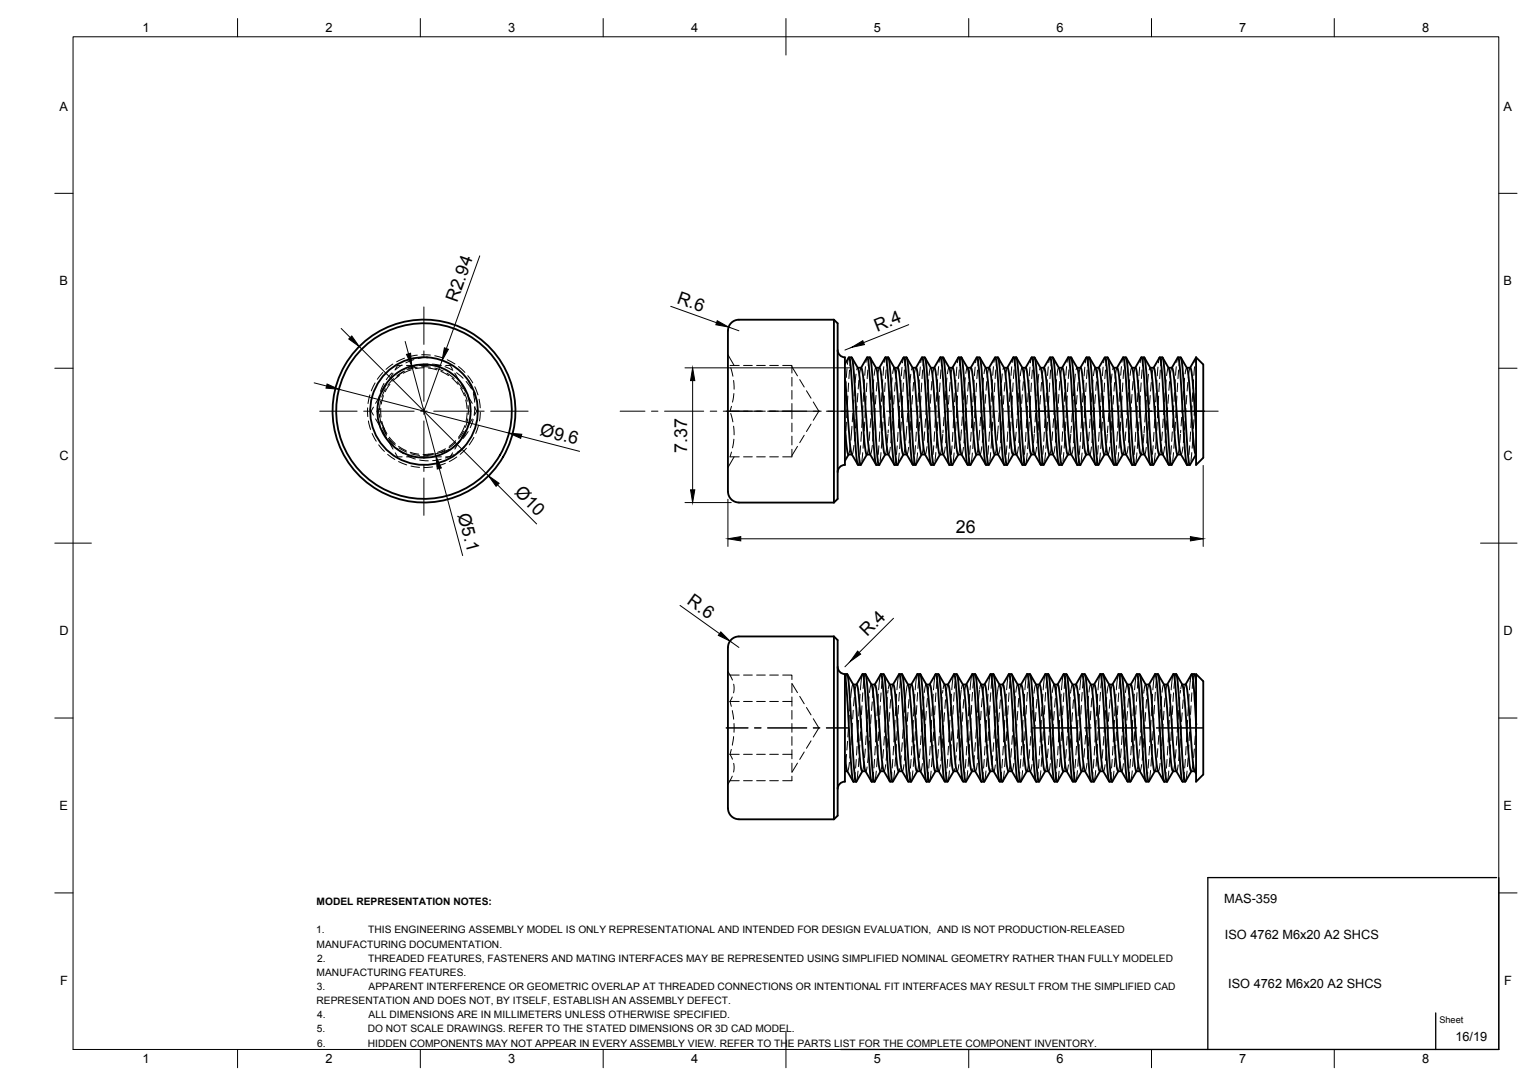
ISO-10303-21;
HEADER;
/* Generated by software containing ST-Developer
 * from STEP Tools, Inc. (www.steptools.com) 
 */

FILE_DESCRIPTION(
/* description */ (''),
/* implementation_level */ '2;1');

FILE_NAME(
/* name */ 'ISO 4762 M6x20 A2 SHCS.step',
/* time_stamp */ '2026-10-15T14:25:16-07:00',
/* author */ (''),
/* organization */ (''),
/* preprocessor_version */ 'ST-DEVELOPER v20.2',
/* originating_system */ 'Autodesk Translation Framework v15.15.0.0',
/* authorisation */ '');

FILE_SCHEMA (('AUTOMOTIVE_DESIGN { 1 0 10303 214 3 1 1 }'));
ENDSEC;

DATA;
#10=MECHANICAL_DESIGN_GEOMETRIC_PRESENTATION_REPRESENTATION('',(#338),#86429);
#157=TOROIDAL_SURFACE('',#17154,0.3342,0.04);
#158=TOROIDAL_SURFACE('',#17170,0.44,0.06);
#256=B_SPLINE_SURFACE_WITH_KNOTS('',3,3,((#76225,#76226,#76227,#76228,#76229,
#76230,#76231,#76232,#76233,#76234,#76235,#76236,#76237,#76238,#76239,#76240,
#76241,#76242,#76243,#76244,#76245,#76246,#76247,#76248,#76249,#76250,#76251,
#76252,#76253,#76254,#76255,#76256,#76257,#76258,#76259,#76260,#76261,#76262,
#76263,#76264,#76265,#76266,#76267,#76268,#76269,#76270,#76271,#76272,#76273,
#76274,#76275,#76276,#76277,#76278,#76279,#76280,#76281,#76282,#76283,#76284,
#76285,#76286,#76287,#76288,#76289,#76290,#76291,#76292,#76293,#76294,#76295,
#76296,#76297,#76298,#76299,#76300,#76301,#76302,#76303,#76304,#76305,#76306,
#76307,#76308,#76309,#76310,#76311,#76312,#76313,#76314,#76315,#76316,#76317,
#76318,#76319,#76320,#76321,#76322,#76323,#76324,#76325,#76326,#76327,#76328,
#76329,#76330,#76331,#76332,#76333,#76334,#76335,#76336,#76337,#76338,#76339,
#76340,#76341,#76342,#76343,#76344,#76345,#76346,#76347,#76348,#76349,#76350),
(#76351,#76352,#76353,#76354,#76355,#76356,#76357,#76358,#76359,#76360,
#76361,#76362,#76363,#76364,#76365,#76366,#76367,#76368,#76369,#76370,#76371,
#76372,#76373,#76374,#76375,#76376,#76377,#76378,#76379,#76380,#76381,#76382,
#76383,#76384,#76385,#76386,#76387,#76388,#76389,#76390,#76391,#76392,#76393,
#76394,#76395,#76396,#76397,#76398,#76399,#76400,#76401,#76402,#76403,#76404,
#76405,#76406,#76407,#76408,#76409,#76410,#76411,#76412,#76413,#76414,#76415,
#76416,#76417,#76418,#76419,#76420,#76421,#76422,#76423,#76424,#76425,#76426,
#76427,#76428,#76429,#76430,#76431,#76432,#76433,#76434,#76435,#76436,#76437,
#76438,#76439,#76440,#76441,#76442,#76443,#76444,#76445,#76446,#76447,#76448,
#76449,#76450,#76451,#76452,#76453,#76454,#76455,#76456,#76457,#76458,#76459,
#76460,#76461,#76462,#76463,#76464,#76465,#76466,#76467,#76468,#76469,#76470,
#76471,#76472,#76473,#76474,#76475,#76476),(#76477,#76478,#76479,#76480,
#76481,#76482,#76483,#76484,#76485,#76486,#76487,#76488,#76489,#76490,#76491,
#76492,#76493,#76494,#76495,#76496,#76497,#76498,#76499,#76500,#76501,#76502,
#76503,#76504,#76505,#76506,#76507,#76508,#76509,#76510,#76511,#76512,#76513,
#76514,#76515,#76516,#76517,#76518,#76519,#76520,#76521,#76522,#76523,#76524,
#76525,#76526,#76527,#76528,#76529,#76530,#76531,#76532,#76533,#76534,#76535,
#76536,#76537,#76538,#76539,#76540,#76541,#76542,#76543,#76544,#76545,#76546,
#76547,#76548,#76549,#76550,#76551,#76552,#76553,#76554,#76555,#76556,#76557,
#76558,#76559,#76560,#76561,#76562,#76563,#76564,#76565,#76566,#76567,#76568,
#76569,#76570,#76571,#76572,#76573,#76574,#76575,#76576,#76577,#76578,#76579,
#76580,#76581,#76582,#76583,#76584,#76585,#76586,#76587,#76588,#76589,#76590,
#76591,#76592,#76593,#76594,#76595,#76596,#76597,#76598,#76599,#76600,#76601,
#76602),(#76603,#76604,#76605,#76606,#76607,#76608,#76609,#76610,#76611,
#76612,#76613,#76614,#76615,#76616,#76617,#76618,#76619,#76620,#76621,#76622,
#76623,#76624,#76625,#76626,#76627,#76628,#76629,#76630,#76631,#76632,#76633,
#76634,#76635,#76636,#76637,#76638,#76639,#76640,#76641,#76642,#76643,#76644,
#76645,#76646,#76647,#76648,#76649,#76650,#76651,#76652,#76653,#76654,#76655,
#76656,#76657,#76658,#76659,#76660,#76661,#76662,#76663,#76664,#76665,#76666,
#76667,#76668,#76669,#76670,#76671,#76672,#76673,#76674,#76675,#76676,#76677,
#76678,#76679,#76680,#76681,#76682,#76683,#76684,#76685,#76686,#76687,#76688,
#76689,#76690,#76691,#76692,#76693,#76694,#76695,#76696,#76697,#76698,#76699,
#76700,#76701,#76702,#76703,#76704,#76705,#76706,#76707,#76708,#76709,#76710,
#76711,#76712,#76713,#76714,#76715,#76716,#76717,#76718,#76719,#76720,#76721,
#76722,#76723,#76724,#76725,#76726,#76727,#76728)),.UNSPECIFIED.,.F.,.F.,
 .F.,(4,4),(4,1,1,1,1,1,1,1,1,1,1,1,1,1,1,1,1,1,1,1,1,1,1,1,1,1,1,1,1,1,
1,1,1,1,1,1,1,1,1,1,1,1,1,1,1,1,1,1,1,1,1,1,1,1,1,1,1,1,1,1,1,1,1,1,1,1,
1,1,1,1,1,1,1,1,1,1,1,1,1,1,1,1,1,1,1,1,1,1,1,1,1,1,1,1,1,1,1,1,1,1,1,1,
1,1,1,1,1,1,1,1,1,1,1,1,1,1,1,1,1,1,1,1,1,4),(-0.000489095128896854,0.0662888134554226),
(8.30725886192223,9.30549431301254,10.303511073624,11.3015278342355,12.299544594847,
13.2975613554585,14.29557811607,15.2935948766815,16.291611637293,17.2896283979046,
18.287645158516,19.2856619191276,20.2836786797391,21.2816954403506,22.2797122009621,
23.2777289615736,24.2757457221851,25.2737624827966,26.2717792434081,27.2697960040196,
28.2678127646311,29.2658295252426,30.2638462858541,31.2618630464656,32.2598798070771,
33.2578965676886,34.2559133283001,35.2539300889116,36.2519468495231,37.2499636101346,
38.2479803707461,39.2459971313576,40.2440138919691,41.2420306525806,42.2400474131921,
43.2380641738036,44.2360809344151,45.2340976950266,46.2321144556381,47.2301312162496,
48.2281479768611,49.2261647374726,50.2241814980841,51.2221982586956,52.2202150193071,
53.2182317799186,54.2162485405301,55.2142653011416,56.2122820617531,57.2102988223646,
58.2083155829761,59.2063323435876,60.2043491041991,61.2023658648106,62.2003826254221,
63.1983993860336,64.1964161466451,65.1944329072566,66.1924496678681,67.1904664284796,
68.1884831890911,69.1864999497026,70.1845167103141,71.1825334709256,72.1805502315371,
73.1785669921486,74.1765837527601,75.1746005133716,76.1726172739831,77.1706340345946,
78.1686507952061,79.1666675558176,80.1646843164291,81.1627010770406,82.1607178376521,
83.1587345982636,84.1567513588751,85.1547681194866,86.1527848800981,87.1508016407096,
88.1488184013211,89.1468351619326,90.1448519225441,91.1428686831556,92.1408854437671,
93.1389022043786,94.1369189649901,95.1349357256016,96.1329524862131,97.1309692468246,
98.1289860074361,99.1270027680476,100.125019528659,101.123036289271,102.121053049882,
103.119069810494,104.117086571105,105.115103331717,106.113120092328,107.11113685294,
108.109153613551,109.107170374163,110.105187134774,111.103203895386,112.101220655997,
113.099237416609,114.09725417722,115.095270937832,116.093287698443,117.091304459055,
118.089321219666,119.087337980278,120.085354740889,121.083371501501,122.081388262112,
123.079405022724,124.077421783335,125.075438543947,126.073455304558,127.07147206517,
128.069488825781,129.067505586393,130.065522347004,131.064028202745),
 .UNSPECIFIED.);
#257=B_SPLINE_SURFACE_WITH_KNOTS('',3,3,((#76851,#76852,#76853,#76854,#76855,
#76856,#76857,#76858,#76859,#76860,#76861,#76862,#76863,#76864,#76865,#76866,
#76867,#76868,#76869,#76870,#76871,#76872,#76873,#76874,#76875,#76876,#76877,
#76878,#76879,#76880,#76881,#76882,#76883,#76884,#76885,#76886,#76887,#76888,
#76889,#76890,#76891,#76892,#76893,#76894,#76895,#76896,#76897,#76898,#76899,
#76900,#76901,#76902,#76903,#76904,#76905,#76906,#76907,#76908,#76909,#76910,
#76911,#76912,#76913,#76914,#76915,#76916,#76917,#76918,#76919,#76920,#76921,
#76922,#76923,#76924,#76925,#76926,#76927,#76928,#76929,#76930,#76931,#76932,
#76933,#76934,#76935,#76936,#76937,#76938,#76939,#76940,#76941,#76942,#76943,
#76944,#76945,#76946,#76947,#76948,#76949,#76950,#76951,#76952,#76953,#76954,
#76955,#76956,#76957,#76958,#76959,#76960,#76961,#76962,#76963,#76964,#76965,
#76966,#76967,#76968,#76969,#76970,#76971,#76972,#76973,#76974,#76975,#76976),
(#76977,#76978,#76979,#76980,#76981,#76982,#76983,#76984,#76985,#76986,
#76987,#76988,#76989,#76990,#76991,#76992,#76993,#76994,#76995,#76996,#76997,
#76998,#76999,#77000,#77001,#77002,#77003,#77004,#77005,#77006,#77007,#77008,
#77009,#77010,#77011,#77012,#77013,#77014,#77015,#77016,#77017,#77018,#77019,
#77020,#77021,#77022,#77023,#77024,#77025,#77026,#77027,#77028,#77029,#77030,
#77031,#77032,#77033,#77034,#77035,#77036,#77037,#77038,#77039,#77040,#77041,
#77042,#77043,#77044,#77045,#77046,#77047,#77048,#77049,#77050,#77051,#77052,
#77053,#77054,#77055,#77056,#77057,#77058,#77059,#77060,#77061,#77062,#77063,
#77064,#77065,#77066,#77067,#77068,#77069,#77070,#77071,#77072,#77073,#77074,
#77075,#77076,#77077,#77078,#77079,#77080,#77081,#77082,#77083,#77084,#77085,
#77086,#77087,#77088,#77089,#77090,#77091,#77092,#77093,#77094,#77095,#77096,
#77097,#77098,#77099,#77100,#77101,#77102),(#77103,#77104,#77105,#77106,
#77107,#77108,#77109,#77110,#77111,#77112,#77113,#77114,#77115,#77116,#77117,
#77118,#77119,#77120,#77121,#77122,#77123,#77124,#77125,#77126,#77127,#77128,
#77129,#77130,#77131,#77132,#77133,#77134,#77135,#77136,#77137,#77138,#77139,
#77140,#77141,#77142,#77143,#77144,#77145,#77146,#77147,#77148,#77149,#77150,
#77151,#77152,#77153,#77154,#77155,#77156,#77157,#77158,#77159,#77160,#77161,
#77162,#77163,#77164,#77165,#77166,#77167,#77168,#77169,#77170,#77171,#77172,
#77173,#77174,#77175,#77176,#77177,#77178,#77179,#77180,#77181,#77182,#77183,
#77184,#77185,#77186,#77187,#77188,#77189,#77190,#77191,#77192,#77193,#77194,
#77195,#77196,#77197,#77198,#77199,#77200,#77201,#77202,#77203,#77204,#77205,
#77206,#77207,#77208,#77209,#77210,#77211,#77212,#77213,#77214,#77215,#77216,
#77217,#77218,#77219,#77220,#77221,#77222,#77223,#77224,#77225,#77226,#77227,
#77228),(#77229,#77230,#77231,#77232,#77233,#77234,#77235,#77236,#77237,
#77238,#77239,#77240,#77241,#77242,#77243,#77244,#77245,#77246,#77247,#77248,
#77249,#77250,#77251,#77252,#77253,#77254,#77255,#77256,#77257,#77258,#77259,
#77260,#77261,#77262,#77263,#77264,#77265,#77266,#77267,#77268,#77269,#77270,
#77271,#77272,#77273,#77274,#77275,#77276,#77277,#77278,#77279,#77280,#77281,
#77282,#77283,#77284,#77285,#77286,#77287,#77288,#77289,#77290,#77291,#77292,
#77293,#77294,#77295,#77296,#77297,#77298,#77299,#77300,#77301,#77302,#77303,
#77304,#77305,#77306,#77307,#77308,#77309,#77310,#77311,#77312,#77313,#77314,
#77315,#77316,#77317,#77318,#77319,#77320,#77321,#77322,#77323,#77324,#77325,
#77326,#77327,#77328,#77329,#77330,#77331,#77332,#77333,#77334,#77335,#77336,
#77337,#77338,#77339,#77340,#77341,#77342,#77343,#77344,#77345,#77346,#77347,
#77348,#77349,#77350,#77351,#77352,#77353,#77354)),.UNSPECIFIED.,.F.,.F.,
 .F.,(4,4),(4,1,1,1,1,1,1,1,1,1,1,1,1,1,1,1,1,1,1,1,1,1,1,1,1,1,1,1,1,1,
1,1,1,1,1,1,1,1,1,1,1,1,1,1,1,1,1,1,1,1,1,1,1,1,1,1,1,1,1,1,1,1,1,1,1,1,
1,1,1,1,1,1,1,1,1,1,1,1,1,1,1,1,1,1,1,1,1,1,1,1,1,1,1,1,1,1,1,1,1,1,1,1,
1,1,1,1,1,1,1,1,1,1,1,1,1,1,1,1,1,1,1,1,1,4),(-0.000418746624015696,0.0663359285465069),
(11.6145437174728,12.6130496084297,13.6110663690412,14.6090831296527,15.6070998902642,
16.6051166508757,17.6031334114872,18.6011501720987,19.5991669327102,20.5971836933217,
21.5952004539332,22.5932172145448,23.5912339751562,24.5892507357678,25.5872674963793,
26.5852842569908,27.5833010176023,28.5813177782138,29.5793345388253,30.5773512994368,
31.5753680600483,32.5733848206598,33.5714015812713,34.5694183418828,35.5674351024943,
36.5654518631058,37.5634686237173,38.5614853843288,39.5595021449403,40.5575189055518,
41.5555356661633,42.5535524267748,43.5515691873863,44.5495859479978,45.5476027086093,
46.5456194692208,47.5436362298323,48.5416529904438,49.5396697510553,50.5376865116668,
51.5357032722783,52.5337200328898,53.5317367935013,54.5297535541128,55.5277703147243,
56.5257870753358,57.5238038359473,58.5218205965588,59.5198373571703,60.5178541177818,
61.5158708783933,62.5138876390048,63.5119043996163,64.5099211602278,65.5079379208393,
66.5059546814508,67.5039714420623,68.5019882026738,69.5000049632853,70.4980217238968,
71.4960384845083,72.4940552451198,73.4920720057313,74.4900887663428,75.4881055269543,
76.4861222875658,77.4841390481773,78.4821558087888,79.4801725694003,80.4781893300118,
81.4762060906233,82.4742228512348,83.4722396118463,84.4702563724578,85.4682731330693,
86.4662898936808,87.4643066542923,88.4623234149038,89.4603401755153,90.4583569361268,
91.4563736967383,92.4543904573498,93.4524072179613,94.4504239785728,95.4484407391843,
96.4464574997958,97.4444742604073,98.4424910210188,99.4405077816303,100.438524542242,
101.436541302853,102.434558063465,103.432574824076,104.430591584688,105.428608345299,
106.426625105911,107.424641866522,108.422658627134,109.420675387745,110.418692148357,
111.416708908968,112.41472566958,113.412742430191,114.410759190803,115.408775951414,
116.406792712026,117.404809472637,118.402826233249,119.40084299386,120.398859754472,
121.396876515083,122.394893275695,123.392910036306,124.390926796918,125.388943557529,
126.386960318141,127.384977078752,128.382993839364,129.381010599975,130.379027360587,
131.377044121198,132.37506088181,133.373077642421,134.371094403033),
 .UNSPECIFIED.);
#273=(
BOUNDED_CURVE()
B_SPLINE_CURVE(2,(#77369,#77370,#77371),.UNSPECIFIED.,.F.,.F.)
B_SPLINE_CURVE_WITH_KNOTS((3,3),(-0.639366558443436,-0.433164349146202),
 .UNSPECIFIED.)
CURVE()
GEOMETRIC_REPRESENTATION_ITEM()
RATIONAL_B_SPLINE_CURVE((1.35866716012837,1.4637604307034,1.4637604307034))
REPRESENTATION_ITEM('')
);
#274=(
BOUNDED_CURVE()
B_SPLINE_CURVE(2,(#77373,#77374,#77375),.UNSPECIFIED.,.F.,.F.)
B_SPLINE_CURVE_WITH_KNOTS((3,3),(0.0319010196424347,0.336489692457453),
 .UNSPECIFIED.)
CURVE()
GEOMETRIC_REPRESENTATION_ITEM()
RATIONAL_B_SPLINE_CURVE((1.03712812921102,1.19757240916823,1.03712812921102))
REPRESENTATION_ITEM('')
);
#275=(
BOUNDED_CURVE()
B_SPLINE_CURVE(2,(#77377,#77378,#77379),.UNSPECIFIED.,.F.,.F.)
B_SPLINE_CURVE_WITH_KNOTS((3,3),(0.0319010196424348,0.336489692457454),
 .UNSPECIFIED.)
CURVE()
GEOMETRIC_REPRESENTATION_ITEM()
RATIONAL_B_SPLINE_CURVE((1.03712812921102,1.19757240916823,1.03712812921102))
REPRESENTATION_ITEM('')
);
#276=(
BOUNDED_CURVE()
B_SPLINE_CURVE(2,(#77381,#77382,#77383),.UNSPECIFIED.,.F.,.F.)
B_SPLINE_CURVE_WITH_KNOTS((3,3),(0.031901019642435,0.336489692457454),
 .UNSPECIFIED.)
CURVE()
GEOMETRIC_REPRESENTATION_ITEM()
RATIONAL_B_SPLINE_CURVE((1.03712812921102,1.19757240916823,1.03712812921102))
REPRESENTATION_ITEM('')
);
#277=(
BOUNDED_CURVE()
B_SPLINE_CURVE(2,(#77385,#77386,#77387),.UNSPECIFIED.,.F.,.F.)
B_SPLINE_CURVE_WITH_KNOTS((3,3),(0.0319010196424349,0.336489692457453),
 .UNSPECIFIED.)
CURVE()
GEOMETRIC_REPRESENTATION_ITEM()
RATIONAL_B_SPLINE_CURVE((1.03712812921102,1.19757240916823,1.03712812921102))
REPRESENTATION_ITEM('')
);
#278=(
BOUNDED_CURVE()
B_SPLINE_CURVE(2,(#77389,#77390,#77391),.UNSPECIFIED.,.F.,.F.)
B_SPLINE_CURVE_WITH_KNOTS((3,3),(0.0319010196424348,0.336489692457453),
 .UNSPECIFIED.)
CURVE()
GEOMETRIC_REPRESENTATION_ITEM()
RATIONAL_B_SPLINE_CURVE((1.03712812921102,1.19757240916823,1.03712812921102))
REPRESENTATION_ITEM('')
);
#279=(
BOUNDED_CURVE()
B_SPLINE_CURVE(2,(#77392,#77393,#77394),.UNSPECIFIED.,.F.,.F.)
B_SPLINE_CURVE_WITH_KNOTS((3,3),(-0.433164349146202,-0.226962139848967),
 .UNSPECIFIED.)
CURVE()
GEOMETRIC_REPRESENTATION_ITEM()
RATIONAL_B_SPLINE_CURVE((1.4637604307034,1.4637604307034,1.35866716012837))
REPRESENTATION_ITEM('')
);
#302=SHAPE_REPRESENTATION_RELATIONSHIP('SRR','None',#86517,#320);
#320=ADVANCED_BREP_SHAPE_REPRESENTATION('',(#356),#86426);
#338=STYLED_ITEM('',(#86616),#356);
#356=MANIFOLD_SOLID_BREP('Body1',#15628);
#947=B_SPLINE_CURVE_WITH_KNOTS('',3,(#66636,#66637,#66638,#66639,#66640,
#66641,#66642,#66643,#66644,#66645,#66646,#66647,#66648,#66649,#66650,#66651,
#66652,#66653,#66654,#66655,#66656,#66657,#66658,#66659,#66660,#66661,#66662,
#66663,#66664,#66665,#66666,#66667,#66668,#66669,#66670,#66671,#66672,#66673,
#66674,#66675,#66676,#66677,#66678,#66679,#66680,#66681,#66682,#66683,#66684,
#66685,#66686,#66687,#66688,#66689,#66690,#66691,#66692,#66693,#66694,#66695,
#66696,#66697,#66698,#66699,#66700,#66701,#66702,#66703,#66704,#66705,#66706,
#66707,#66708,#66709,#66710,#66711),.UNSPECIFIED.,.F.,.F.,(4,3,3,3,3,3,
3,3,3,3,3,3,3,3,3,3,3,3,3,3,3,3,3,3,3,4),(10.3765110117404,10.553450790841,
10.7300519237118,10.9066404614712,11.0832321762531,11.2602038202997,11.3015278342355,
11.4805049057995,11.6591300536428,11.837736646534,12.0163195055085,12.1953225046721,
12.299544594847,12.477964982007,12.6560183737272,12.8340392590285,13.0120277045372,
13.190434319541,13.2975613554585,13.4762752215219,13.6546274568134,13.8329507487056,
14.0112440633789,14.1899534235983,14.29557811607,14.315035395632),
 .UNSPECIFIED.);
#948=B_SPLINE_CURVE_WITH_KNOTS('',3,(#66714,#66715,#66716,#66717,#66718,
#66719,#66720,#66721,#66722,#66723,#66724,#66725,#66726,#66727,#66728,#66729,
#66730,#66731,#66732,#66733,#66734,#66735,#66736,#66737,#66738,#66739,#66740,
#66741,#66742,#66743,#66744,#66745,#66746,#66747,#66748,#66749,#66750,#66751,
#66752,#66753,#66754,#66755,#66756,#66757,#66758,#66759,#66760,#66761,#66762),
 .UNSPECIFIED.,.F.,.F.,(4,3,3,3,3,3,3,3,3,3,3,3,3,3,3,3,4),(11.6150328478182,
11.7979606486813,11.9807538318031,12.1637609224241,12.3468733973939,12.5304979994706,
12.6130496084297,12.7898803693582,12.9663087351348,13.1426740016011,13.3189861820381,
13.4957160141166,13.6110663690412,13.790004086606,13.9685863611197,14.1471565225389,
14.3143732599613),.UNSPECIFIED.);
#949=B_SPLINE_CURVE_WITH_KNOTS('',3,(#66768,#66769,#66770,#66771,#66772,
#66773,#66774,#66775,#66776,#66777,#66778,#66779,#66780,#66781,#66782,#66783,
#66784,#66785,#66786,#66787,#66788,#66789,#66790,#66791,#66792,#66793,#66794,
#66795,#66796,#66797,#66798,#66799,#66800,#66801,#66802,#66803,#66804,#66805,
#66806,#66807,#66808,#66809,#66810,#66811,#66812,#66813,#66814,#66815,#66816,
#66817,#66818,#66819,#66820,#66821,#66822,#66823,#66824,#66825,#66826,#66827,
#66828,#66829,#66830,#66831,#66832,#66833,#66834,#66835,#66836,#66837,#66838,
#66839,#66840,#66841,#66842,#66843,#66844,#66845,#66846,#66847,#66848,#66849,
#66850,#66851,#66852,#66853,#66854,#66855,#66856,#66857,#66858,#66859,#66860,
#66861,#66862,#66863,#66864,#66865,#66866,#66867,#66868,#66869,#66870,#66871,
#66872,#66873,#66874,#66875,#66876,#66877,#66878,#66879,#66880,#66881,#66882,
#66883,#66884,#66885,#66886,#66887,#66888,#66889,#66890,#66891,#66892,#66893,
#66894,#66895,#66896,#66897,#66898,#66899,#66900,#66901,#66902,#66903,#66904,
#66905,#66906,#66907,#66908,#66909,#66910,#66911,#66912,#66913,#66914,#66915,
#66916,#66917,#66918,#66919,#66920,#66921,#66922,#66923,#66924,#66925,#66926,
#66927,#66928,#66929,#66930,#66931,#66932,#66933,#66934,#66935,#66936,#66937,
#66938,#66939,#66940,#66941,#66942,#66943),.UNSPECIFIED.,.F.,.F.,(4,2,2,
2,2,2,2,2,2,2,2,2,2,2,2,2,2,2,2,2,2,2,2,2,2,2,2,2,2,2,2,2,2,2,2,2,2,2,2,
2,2,2,2,2,2,2,2,2,2,2,2,2,2,2,2,2,2,2,2,2,2,2,2,2,2,2,2,2,2,2,2,2,2,2,2,
2,2,2,2,2,2,2,2,2,2,2,2,4),(-1.16393024442893,-1.1221121315859,-1.10881872775493,
-1.09544934716449,-1.09173058973152,-1.08953019556074,-1.08752664172342,
-1.08475168761754,-1.07807017871904,-1.06837433006326,-1.03766271561164,
-0.986967317852749,-0.977454673078762,-0.972924462585128,-0.969395708425164,
-0.965480163368157,-0.958971176180976,-0.932462287603271,-0.898938534238497,
-0.862323864343115,-0.856094385560679,-0.853588717151212,-0.851567613516379,
-0.849448493062549,-0.846097056573953,-0.835079364231314,-0.81540391299286,
-0.803966476133666,-0.749205411550143,-0.739933534931748,-0.735449519421135,
-0.731926722665925,-0.727986733892083,-0.721362440590357,-0.693068305980396,
-0.661126188336577,-0.62498318336144,-0.618724065166356,-0.616213585950999,
-0.614191439698589,-0.612074386397869,-0.608732469713031,-0.597803658723205,
-0.578369392903072,-0.565103910874299,-0.512002169030124,-0.502609093783704,
-0.498101699222849,-0.494575904380125,-0.490648422164753,-0.484083268407897,
-0.456726688401616,-0.424134078931558,-0.387566159612312,-0.38133545021858,
-0.37882929357464,-0.376807817974159,-0.374687075157398,-0.371333009017104,
-0.360304955609168,-0.340603341285605,-0.333711435315054,-0.273565360251425,
-0.264992529056898,-0.260586706715257,-0.257245427320754,-0.253405341354982,
-0.249363595655126,-0.24334388884479,-0.232352183683043,-0.205509402738985,
-0.167177413247694,-0.146863476916789,-0.142705047485694,-0.14038371096495,
-0.138409430867859,-0.135855093702301,-0.130411237430462,-0.123009150411749,
-0.103368057562215,-0.0503645383585366,-0.0314881958645743,-0.02544491739472,
-0.0216335334546739,-0.0182616452424589,-0.0148096369960941,-0.00864602604130215,
-0.00070557473632002),.UNSPECIFIED.);
#950=B_SPLINE_CURVE_WITH_KNOTS('',3,(#66944,#66945,#66946,#66947,#66948,
#66949,#66950,#66951,#66952,#66953,#66954,#66955,#66956,#66957,#66958,#66959,
#66960,#66961,#66962,#66963,#66964,#66965,#66966,#66967,#66968,#66969,#66970,
#66971),.UNSPECIFIED.,.F.,.F.,(4,3,3,3,3,3,3,3,3,4),(14.315035395632,14.4936872514172,
14.6719976991658,14.8502987123366,15.0285878152494,15.2072891407824,15.2935948766815,
15.4900540694702,15.685111908359,15.7079632676251),.UNSPECIFIED.);
#951=B_SPLINE_CURVE_WITH_KNOTS('',3,(#66973,#66974,#66975,#66976,#66977,
#66978,#66979,#66980,#66981,#66982,#66983,#66984,#66985,#66986,#66987,#66988,
#66989,#66990,#66991,#66992,#66993,#66994,#66995,#66996,#66997,#66998,#66999,
#67000),.UNSPECIFIED.,.F.,.F.,(4,3,3,3,3,3,3,3,3,4),(14.3143732599613,14.4932818470659,
14.6090831296527,14.7880601048648,14.9666851520948,15.1452916394554,15.3238743899854,
15.5028772782052,15.6070998902642,15.7079632679489),.UNSPECIFIED.);
#952=B_SPLINE_CURVE_WITH_KNOTS('',3,(#67001,#67002,#67003,#67004,#67005,
#67006,#67007,#67008,#67009,#67010,#67011,#67012,#67013,#67014,#67015,#67016,
#67017,#67018,#67019,#67020,#67021,#67022,#67023,#67024,#67025,#67026,#67027,
#67028,#67029,#67030,#67031,#67032,#67033,#67034,#67035,#67036,#67037,#67038,
#67039,#67040,#67041,#67042,#67043,#67044,#67045,#67046,#67047,#67048,#67049,
#67050,#67051,#67052,#67053,#67054,#67055,#67056,#67057,#67058,#67059,#67060,
#67061,#67062,#67063,#67064,#67065,#67066,#67067,#67068,#67069,#67070,#67071,
#67072,#67073,#67074,#67075,#67076,#67077,#67078,#67079,#67080,#67081,#67082,
#67083,#67084,#67085,#67086,#67087,#67088,#67089,#67090,#67091,#67092,#67093,
#67094,#67095,#67096,#67097,#67098,#67099,#67100,#67101,#67102,#67103,#67104,
#67105,#67106,#67107,#67108,#67109,#67110,#67111,#67112,#67113,#67114,#67115,
#67116,#67117,#67118,#67119,#67120,#67121,#67122,#67123,#67124,#67125,#67126,
#67127,#67128,#67129,#67130,#67131,#67132,#67133,#67134,#67135,#67136,#67137,
#67138,#67139,#67140,#67141,#67142,#67143,#67144,#67145,#67146,#67147,#67148,
#67149,#67150,#67151,#67152,#67153,#67154,#67155,#67156,#67157,#67158,#67159,
#67160,#67161,#67162),.UNSPECIFIED.,.F.,.F.,(4,2,2,2,2,2,2,2,2,2,2,2,2,
2,2,2,2,2,2,2,2,2,2,2,2,2,2,2,2,2,2,2,2,2,2,2,2,2,2,2,2,2,2,2,2,2,2,2,2,
2,2,2,2,2,2,2,2,2,2,2,2,2,2,2,2,2,2,2,2,2,2,2,2,2,2,2,2,2,2,2,4),(-2.98942615939622,
-2.94687744843447,-2.90737887780196,-2.90028833462003,-2.89626757009887,
-2.89278736806544,-2.88850740594506,-2.88194860504523,-2.83799867893463,
-2.79959280759611,-2.78803138120337,-2.78284147994681,-2.7788283302866,
-2.77655245813013,-2.7747160432841,-2.77226099931904,-2.76840197913877,
-2.74684477299445,-2.7014833079237,-2.66913041899145,-2.66227335609882,
-2.65827801354727,-2.65475565048187,-2.65033879153963,-2.64173110989955,
-2.58217996827536,-2.57531649807323,-2.55547164910086,-2.54439033061707,
-2.5410244222646,-2.53889684010004,-2.53687348626668,-2.53436524742632,
-2.52813036525468,-2.4917679525961,-2.45944377174351,-2.43180998977834,
-2.42522856169367,-2.42129812597274,-2.41777390166482,-2.41327434396693,
-2.40391952697214,-2.35010438134218,-2.33761336325053,-2.31801429303953,
-2.30702655289876,-2.30367990062065,-2.30156294068283,-2.29954488717194,
-2.29704277121525,-2.29082111843716,-2.25423947569581,-2.22151065226755,
-2.19433476155473,-2.18778874877106,-2.18386961472211,-2.18034945389465,
-2.17584679667526,-2.16645503385871,-2.11336918408685,-2.10013504463255,
-2.08062743095894,-2.06967603867303,-2.06633508998146,-2.06422055344751,
-2.06220017101256,-2.05969362054567,-2.05345255268914,-2.01714235715239,
-1.98492427180508,-1.95706758364123,-1.9504713292746,-1.94653757415735,
-1.94301382477905,-1.9385196018074,-1.92919317744503,-1.87520561547252,
-1.83454429703135,-1.83001991115689,-1.8276461646142,-1.82654679620979),
 .UNSPECIFIED.);
#953=B_SPLINE_CURVE_WITH_KNOTS('',3,(#67167,#67168,#67169,#67170,#67171,
#67172,#67173,#67174,#67175,#67176,#67177,#67178,#67179,#67180,#67181,#67182,
#67183,#67184,#67185,#67186,#67187,#67188,#67189,#67190,#67191,#67192,#67193,
#67194,#67195,#67196,#67197,#67198,#67199,#67200,#67201,#67202,#67203,#67204,
#67205,#67206,#67207,#67208,#67209,#67210,#67211,#67212,#67213,#67214,#67215,
#67216,#67217,#67218,#67219,#67220,#67221,#67222,#67223,#67224,#67225,#67226,
#67227,#67228,#67229,#67230,#67231,#67232,#67233,#67234,#67235,#67236,#67237,
#67238,#67239,#67240,#67241,#67242,#67243,#67244,#67245,#67246,#67247,#67248,
#67249,#67250,#67251,#67252,#67253,#67254,#67255,#67256,#67257,#67258,#67259,
#67260,#67261,#67262,#67263,#67264,#67265,#67266,#67267,#67268,#67269,#67270,
#67271,#67272,#67273,#67274,#67275,#67276,#67277,#67278,#67279,#67280,#67281,
#67282,#67283,#67284,#67285,#67286,#67287,#67288,#67289,#67290,#67291,#67292,
#67293,#67294,#67295,#67296,#67297,#67298,#67299,#67300,#67301,#67302,#67303,
#67304,#67305,#67306,#67307,#67308,#67309,#67310,#67311,#67312,#67313,#67314,
#67315,#67316,#67317,#67318,#67319,#67320,#67321,#67322,#67323,#67324,#67325,
#67326,#67327,#67328,#67329,#67330,#67331,#67332,#67333,#67334,#67335,#67336,
#67337,#67338,#67339,#67340,#67341,#67342,#67343,#67344,#67345,#67346,#67347,
#67348,#67349,#67350,#67351,#67352,#67353,#67354,#67355,#67356,#67357,#67358,
#67359,#67360,#67361,#67362,#67363,#67364,#67365,#67366,#67367,#67368,#67369,
#67370,#67371,#67372,#67373,#67374,#67375,#67376,#67377,#67378,#67379,#67380,
#67381,#67382),.UNSPECIFIED.,.F.,.F.,(4,2,2,2,2,2,2,2,2,2,2,2,2,2,2,2,2,
2,2,2,2,2,2,2,2,2,2,2,2,2,2,2,2,2,2,2,2,2,2,2,2,2,2,2,2,2,2,2,2,2,2,2,2,
2,2,2,2,2,2,2,2,2,2,2,2,2,2,2,2,2,2,2,2,2,2,2,2,2,2,2,2,2,2,2,2,2,2,2,2,
2,2,2,2,2,2,2,2,2,2,2,2,2,2,2,2,2,2,4),(-2.65811385973918,-2.64341887280631,
-2.63685547945785,-2.63292924488921,-2.62940468727833,-2.62489903708624,
-2.61551025001664,-2.56238128523994,-2.54919264361674,-2.52971894580261,
-2.51877761208218,-2.51543481805796,-2.51331789853485,-2.51129633688125,
-2.50878716273528,-2.50253408200726,-2.46640007387792,-2.43445651631383,
-2.40623004475929,-2.39961108197887,-2.39567265610066,-2.39215024322409,
-2.38766531765506,-2.37838640297329,-2.32371253981176,-2.31218416854247,
-2.29250660917671,-2.28148985781449,-2.27813883561977,-2.27602003237057,
-2.27399956303752,-2.27149476126776,-2.26526776294454,-2.22872118194875,
-2.1961529858716,-2.16881232025688,-2.16224953615428,-2.1583231805186,-2.15479821019637,
-2.15029161224657,-2.14089927817996,-2.08780637972958,-2.07456150657982,
-2.05509772052212,-2.04415967673414,-2.04081702101019,-2.03869999347207,
-2.03667816505093,-2.03416848444712,-2.02791325698376,-1.99179456385597,
-1.95987879084501,-1.93160587948036,-1.924983541931,-1.92104413243149,-1.91752147569834,
-1.91303711126042,-1.90376257244495,-1.84901801727298,-1.83755339109749,
-1.81786820831232,-1.80684826104643,-1.80349666903814,-1.8013775956048,
-1.79935691668679,-1.79685192957958,-1.79062483873777,-1.75406198815898,
-1.72147300873686,-1.69415644155959,-1.68759468993854,-1.68366826775868,
-1.68014280788343,-1.67563498858127,-1.66623787311483,-1.61320062663609,
-1.57165631512584,-1.56711236676727,-1.56473481914091,-1.56276388018841,
-1.56027892884346,-1.55632224374582,-1.53211804490594,-1.49545586039646,
-1.45803901320214,-1.45087621560002,-1.44677758808614,-1.44330536420355,
-1.43906067168766,-1.43099906766286,-1.38669425295883,-1.33778773774552,
-1.33106359083246,-1.32847789303883,-1.32661927783257,-1.32456966534925,
-1.32154352722031,-1.31319780845717,-1.30005877224877,-1.27130435927623,
-1.22453385002851,-1.21502442574756,-1.21047808041805,-1.20693773371413,
-1.20307033969169,-1.19678165452462,-1.17322533761841,-1.16393024442893),
 .UNSPECIFIED.);
#954=B_SPLINE_CURVE_WITH_KNOTS('',3,(#67383,#67384,#67385,#67386,#67387,
#67388,#67389,#67390,#67391,#67392,#67393,#67394,#67395,#67396,#67397,#67398,
#67399,#67400,#67401,#67402,#67403,#67404,#67405,#67406,#67407,#67408,#67409,
#67410,#67411,#67412,#67413,#67414,#67415,#67416,#67417,#67418,#67419,#67420,
#67421,#67422,#67423,#67424,#67425,#67426,#67427,#67428,#67429,#67430,#67431,
#67432,#67433,#67434,#67435,#67436,#67437,#67438,#67439,#67440,#67441,#67442,
#67443,#67444,#67445,#67446,#67447,#67448,#67449,#67450,#67451,#67452,#67453,
#67454,#67455,#67456,#67457,#67458,#67459,#67460,#67461,#67462,#67463,#67464,
#67465,#67466,#67467,#67468,#67469,#67470,#67471,#67472,#67473,#67474,#67475,
#67476,#67477,#67478,#67479,#67480,#67481,#67482,#67483,#67484,#67485,#67486,
#67487,#67488,#67489,#67490,#67491,#67492,#67493,#67494,#67495,#67496,#67497,
#67498,#67499,#67500,#67501,#67502,#67503,#67504,#67505,#67506,#67507,#67508,
#67509,#67510,#67511,#67512,#67513,#67514,#67515,#67516,#67517,#67518,#67519,
#67520,#67521,#67522,#67523,#67524,#67525,#67526,#67527,#67528,#67529,#67530,
#67531,#67532,#67533,#67534,#67535,#67536,#67537,#67538,#67539,#67540,#67541,
#67542,#67543,#67544,#67545,#67546,#67547,#67548,#67549,#67550,#67551,#67552,
#67553,#67554,#67555,#67556,#67557,#67558,#67559,#67560,#67561,#67562,#67563,
#67564,#67565,#67566,#67567,#67568,#67569,#67570,#67571,#67572,#67573,#67574,
#67575,#67576,#67577,#67578,#67579,#67580,#67581,#67582,#67583,#67584,#67585,
#67586,#67587,#67588,#67589,#67590,#67591,#67592),.UNSPECIFIED.,.F.,.F.,
(4,2,2,2,2,2,2,2,2,2,2,2,2,2,2,2,2,2,2,2,2,2,2,2,2,2,2,2,2,2,2,2,2,2,2,
2,2,2,2,2,2,2,2,2,2,2,2,2,2,2,2,2,2,2,2,2,2,2,2,2,2,2,2,2,2,2,2,2,2,2,2,
2,2,2,2,2,2,2,2,2,2,2,2,2,2,2,2,2,2,2,2,2,2,2,2,2,2,2,2,2,2,2,2,2,4),(-1.82654679620979,
-1.82567514256061,-1.82318578987642,-1.81921319040424,-1.7945975999961,
-1.78085997278393,-1.7509591994889,-1.72013307652391,-1.71336497138031,
-1.70939473836614,-1.7058785560794,-1.70144836983348,-1.69274827174082,
-1.63351771519777,-1.59712820036903,-1.59263831113477,-1.59027268554199,
-1.58830213870627,-1.58580575376867,-1.58180878732842,-1.55563188197764,
-1.54336480304901,-1.51968739046691,-1.49541669681936,-1.48036462094594,
-1.4747971116956,-1.47145663595873,-1.4678957223663,-1.46312196202823,-1.45224427397563,
-1.4122393108637,-1.3631967470555,-1.35660554113805,-1.35404011821867,-1.35218727325777,
-1.35013310945877,-1.34708239148078,-1.33855327348186,-1.32500659946013,
-1.25894060115722,-1.24314452828203,-1.23747258219032,-1.23411196404678,
-1.23056076484228,-1.22585342218376,-1.21536014310749,-1.20098137192243,
-1.15815776541184,-1.12236958235826,-1.118324968688,-1.11581402318508,-1.11384229735801,
-1.11148754612972,-1.10705055497943,-1.0743623081271,-1.02123830959475,
-1.00570661802811,-1.00007250684677,-0.996719268033883,-0.99316482249979,
-0.988434287423803,-0.977807444331893,-0.963186142593477,-0.918897988539242,
-0.885062430743449,-0.880985310049003,-0.878464863782423,-0.876492741512126,
-0.874145914767134,-0.869746244582656,-0.838975300467984,-0.79077979564977,
-0.769698590801541,-0.76340651574252,-0.759539578751323,-0.756001334220189,
-0.751382768040408,-0.741383638800634,-0.727888289896724,-0.689928879494222,
-0.650504547981136,-0.6443072230176,-0.641807771155571,-0.639788998631064,
-0.637668699900011,-0.634309761118168,-0.623215004476113,-0.603326541332951,
-0.595162166258294,-0.536884376366843,-0.52796871893014,-0.5235543137147,
-0.520039551252073,-0.51605907889055,-0.509243845237497,-0.477522095825476,
-0.430973442848463,-0.40989771349916,-0.405690896618916,-0.403359372530627,
-0.401385809699974,-0.398845112426623,-0.393478933319888,-0.355248774809182,
-0.332190119670129),.UNSPECIFIED.);
#955=B_SPLINE_CURVE_WITH_KNOTS('',3,(#67598,#67599,#67600,#67601,#67602,
#67603,#67604,#67605,#67606,#67607,#67608,#67609,#67610,#67611,#67612,#67613,
#67614,#67615,#67616,#67617,#67618,#67619,#67620,#67621,#67622,#67623,#67624,
#67625,#67626,#67627,#67628,#67629,#67630,#67631,#67632,#67633,#67634,#67635,
#67636,#67637,#67638,#67639,#67640,#67641,#67642,#67643,#67644,#67645,#67646,
#67647,#67648,#67649,#67650,#67651,#67652,#67653,#67654,#67655,#67656,#67657,
#67658,#67659,#67660,#67661,#67662,#67663,#67664,#67665,#67666,#67667,#67668,
#67669,#67670,#67671,#67672,#67673,#67674,#67675,#67676,#67677,#67678,#67679,
#67680,#67681,#67682,#67683,#67684,#67685,#67686,#67687,#67688,#67689,#67690,
#67691,#67692,#67693,#67694,#67695,#67696,#67697,#67698,#67699,#67700,#67701,
#67702,#67703,#67704,#67705,#67706,#67707,#67708,#67709,#67710,#67711,#67712,
#67713,#67714,#67715,#67716,#67717,#67718,#67719,#67720,#67721,#67722,#67723,
#67724,#67725,#67726,#67727,#67728,#67729,#67730,#67731,#67732,#67733,#67734,
#67735,#67736,#67737,#67738,#67739,#67740,#67741,#67742,#67743,#67744,#67745,
#67746,#67747,#67748,#67749,#67750,#67751,#67752,#67753,#67754,#67755,#67756,
#67757,#67758,#67759,#67760,#67761,#67762,#67763),.UNSPECIFIED.,.F.,.F.,
(4,2,2,2,2,2,2,2,2,2,2,2,2,2,2,2,2,2,2,2,2,2,2,2,2,2,2,2,2,2,2,2,2,2,2,
2,2,2,2,2,2,2,2,2,2,2,2,2,2,2,2,2,2,2,2,2,2,2,2,2,2,2,2,2,2,2,2,2,2,2,2,
2,2,2,2,2,2,2,2,2,2,2,4),(-1.16365104910194,-1.16198873409848,-1.11873333451251,
-1.08007682483228,-1.07289533808751,-1.06879292991221,-1.06532147429848,
-1.06108261121265,-1.05304736223389,-1.01380643672128,-0.974354768874303,
-0.955615421727428,-0.95154095556962,-0.949238925381929,-0.947279975777236,
-0.944706537452359,-0.939168763503621,-0.931601350956711,-0.911272521420545,
-0.864697156551351,-0.841359959454907,-0.834859417924407,-0.830946538256954,
-0.827418656268732,-0.822887438665612,-0.813364699776189,-0.800702995228171,
-0.766805215685698,-0.721392566400016,-0.715391258738159,-0.712957370947077,
-0.710954958021573,-0.708805444312101,-0.705315425122888,-0.692920314092189,
-0.669266049918139,-0.611703523646731,-0.600662162343852,-0.596217640945699,
-0.592926913172538,-0.589328930082488,-0.584341614312926,-0.572173887692835,
-0.506645012856004,-0.504000582658459,-0.493537335427797,-0.480167288699852,
-0.476449005709923,-0.474249008124355,-0.47224603922321,-0.4694720984499,
-0.462793799245578,-0.45310336172613,-0.422417340554128,-0.37169541728193,
-0.362185648162151,-0.357656682611973,-0.35412885374973,-0.35021429531376,
-0.343706866024677,-0.317203459323662,-0.28368579624041,-0.247072372632416,
-0.240849064767332,-0.238124138572478,-0.236151648600852,-0.234309633850536,
-0.231056093345189,-0.220914738422784,-0.203536525041064,-0.150699833390058,
-0.128996687355292,-0.122647285439585,-0.118767180860785,-0.11523123553389,
-0.110636222873976,-0.1007701932916,-0.0875102476811494,-0.0507450523485492,
-0.00710859726825555,-0.00274825577811126,-0.00126848880133153,-0.000702321398189432),
 .UNSPECIFIED.);
#956=B_SPLINE_CURVE_WITH_KNOTS('',3,(#67764,#67765,#67766,#67767,#67768,
#67769,#67770,#67771,#67772,#67773,#67774,#67775,#67776,#67777,#67778,#67779,
#67780,#67781,#67782,#67783,#67784,#67785,#67786,#67787,#67788,#67789,#67790,
#67791,#67792,#67793,#67794,#67795,#67796,#67797,#67798,#67799,#67800,#67801,
#67802,#67803,#67804,#67805,#67806,#67807,#67808,#67809,#67810,#67811,#67812,
#67813,#67814,#67815),.UNSPECIFIED.,.F.,.F.,(4,2,2,2,2,2,2,2,2,2,2,2,2,
2,2,2,2,2,2,2,2,2,2,2,2,4),(-2.9893848513208,-2.98893747316369,-2.9876025158476,
-2.98546557946283,-2.98216250725133,-2.97197352792502,-2.96355815815491,
-2.90631730564084,-2.88926272540383,-2.87733951087504,-2.87239217835099,
-2.86880219859959,-2.86550441099093,-2.86102835754096,-2.84979189282628,
-2.77362471164541,-2.76248320507388,-2.75507907488132,-2.75285138792675,
-2.75074533201809,-2.74881523310293,-2.7460912084198,-2.739870957641,-2.7033280354885,
-2.67077630094081,-2.65811385973918),.UNSPECIFIED.);
#957=B_SPLINE_CURVE_WITH_KNOTS('',3,(#67817,#67818,#67819,#67820,#67821,
#67822,#67823,#67824,#67825,#67826,#67827,#67828,#67829,#67830,#67831,#67832,
#67833,#67834,#67835,#67836,#67837,#67838,#67839,#67840,#67841,#67842,#67843,
#67844,#67845,#67846,#67847,#67848,#67849,#67850,#67851,#67852,#67853,#67854,
#67855,#67856,#67857,#67858,#67859,#67860,#67861,#67862,#67863,#67864,#67865,
#67866,#67867,#67868,#67869,#67870,#67871,#67872,#67873,#67874,#67875,#67876,
#67877,#67878,#67879,#67880,#67881,#67882,#67883,#67884,#67885,#67886,#67887,
#67888,#67889,#67890,#67891,#67892,#67893,#67894,#67895,#67896,#67897,#67898,
#67899,#67900,#67901,#67902,#67903,#67904,#67905,#67906,#67907,#67908,#67909,
#67910,#67911,#67912),.UNSPECIFIED.,.F.,.F.,(4,2,2,2,2,2,2,2,2,2,2,2,2,
2,2,2,2,2,2,2,2,2,2,2,2,2,2,2,2,2,2,2,2,2,2,2,2,2,2,2,2,2,2,2,2,2,2,4),
(-0.332190119670129,-0.299974256783078,-0.29076182289428,-0.286290157332493,
-0.282769813927846,-0.282625201287161,-0.282512604791512,-0.282424919666148,
-0.282356617668773,-0.282303400836696,-0.282223074884288,-0.2821468634119,
-0.282074529573626,-0.282005851482837,-0.281940621293291,-0.281878644309835,
-0.281819738143039,-0.281763731896355,-0.281710465402988,-0.281659788503258,
-0.281611560369081,-0.281565648872144,-0.281521929981461,-0.281480287226152,
-0.28144061117419,-0.281402798955855,-0.281366753823448,-0.277086765497933,
-0.268113946574196,-0.25627891769557,-0.226021878457394,-0.178535972958935,
-0.17031557559799,-0.167215471896808,-0.165356270008634,-0.163309071896805,
-0.160291684989588,-0.152003104953454,-0.10448895096256,-0.0779098348769532,
-0.05747216958326,-0.0512538036654406,-0.0474028352405869,-0.0438597472645543,
-0.0403992630740389,-0.0358762841793266,-0.023929538719514,-0.000702291658524479),
 .UNSPECIFIED.);
#958=B_SPLINE_CURVE_WITH_KNOTS('',3,(#67913,#67914,#67915,#67916,#67917,
#67918,#67919,#67920,#67921,#67922,#67923,#67924,#67925,#67926,#67927,#67928,
#67929,#67930,#67931,#67932,#67933,#67934,#67935,#67936,#67937,#67938,#67939,
#67940,#67941,#67942,#67943,#67944,#67945,#67946,#67947,#67948,#67949,#67950,
#67951,#67952,#67953,#67954,#67955,#67956,#67957,#67958,#67959,#67960,#67961,
#67962,#67963,#67964,#67965,#67966,#67967,#67968,#67969,#67970,#67971,#67972,
#67973,#67974,#67975,#67976,#67977,#67978,#67979,#67980,#67981,#67982,#67983,
#67984,#67985,#67986,#67987,#67988,#67989,#67990,#67991,#67992,#67993,#67994,
#67995,#67996,#67997,#67998,#67999,#68000,#68001,#68002,#68003,#68004,#68005,
#68006,#68007,#68008,#68009,#68010,#68011,#68012,#68013,#68014,#68015,#68016,
#68017,#68018,#68019,#68020,#68021,#68022,#68023,#68024,#68025,#68026,#68027,
#68028,#68029,#68030,#68031,#68032,#68033,#68034,#68035,#68036,#68037,#68038,
#68039,#68040,#68041,#68042,#68043,#68044,#68045,#68046,#68047,#68048,#68049,
#68050,#68051,#68052,#68053,#68054,#68055,#68056,#68057,#68058,#68059,#68060,
#68061,#68062,#68063,#68064,#68065,#68066,#68067,#68068,#68069,#68070,#68071,
#68072,#68073,#68074,#68075,#68076,#68077,#68078,#68079,#68080,#68081,#68082,
#68083,#68084,#68085,#68086,#68087,#68088,#68089,#68090,#68091,#68092,#68093,
#68094,#68095,#68096,#68097,#68098,#68099,#68100,#68101,#68102,#68103,#68104,
#68105,#68106,#68107,#68108),.UNSPECIFIED.,.F.,.F.,(4,2,2,2,2,2,2,2,2,2,
2,2,2,2,2,2,2,2,2,2,2,2,2,2,2,2,2,2,2,2,2,2,2,2,2,2,2,2,2,2,2,2,2,2,2,2,
2,2,2,2,2,2,2,2,2,2,2,2,2,2,2,2,2,2,2,2,2,2,2,2,2,2,2,2,2,2,2,2,2,2,2,2,
2,2,2,2,2,2,2,2,2,2,2,2,2,2,2,4),(-2.98897358008687,-2.92769314209762,-2.92283635649671,
-2.91891607758328,-2.91667246239068,-2.91468429829351,-2.9120511288804,
-2.90602483674824,-2.85973597595541,-2.82644850336208,-2.81392147458867,
-2.80456842641748,-2.80028193766707,-2.80021757807928,-2.80014854592242,
-2.80007429804235,-2.79999420251525,-2.79990751963336,-2.79981337778569,
-2.79971074256605,-2.79959837680186,-2.79947478825607,-2.7993381603811,
-2.79918625944562,-2.79910282444393,-2.79894676733214,-2.7986404194696,
-2.79512089876872,-2.79065274727909,-2.78145663265082,-2.7261184372274,
-2.68653475198969,-2.68201786236957,-2.67964667784219,-2.6776764846138,
-2.67518682288345,-2.67121230847029,-2.6465385500168,-2.60381980183744,
-2.57218735140361,-2.56537747406849,-2.56139840445967,-2.55788383669279,
-2.55346828700893,-2.54454549542632,-2.48629755644931,-2.47808810643394,
-2.45818707535278,-2.44708889637699,-2.44372974284319,-2.44160952912779,
-2.4395909662627,-2.43709198168734,-2.43089673012719,-2.3914888195501,-2.35356167696314,
-2.34007362068281,-2.33007780218808,-2.32545997520698,-2.32192195528628,
-2.31805492340576,-2.3117619328311,-2.29066986050776,-2.24245176471885,
-2.21166913656067,-2.20726891292452,-2.20492200279276,-2.20294992363011,
-2.20042969097544,-2.19635325451221,-2.16252425488423,-2.1577595822794,
-2.12368275873593,-2.09697182148208,-2.09045172116841,-2.08653517742575,
-2.08300913125178,-2.07848745284167,-2.06901214652698,-2.01745666702726,
-1.98731902900585,-1.97772631630079,-1.9710993642418,-1.96833439561336,
-1.96633333461326,-1.96413046746479,-1.96039731815009,-1.94685350251339,
-1.93673283316637,-1.92126868736453,-1.8800268546076,-1.86592293387262,
-1.85558121982064,-1.85090091581163,-1.84735388977835,-1.84351479821116,
-1.83735142483573,-1.82625073863295),.UNSPECIFIED.);
#959=B_SPLINE_CURVE_WITH_KNOTS('',3,(#68113,#68114,#68115,#68116,#68117,
#68118,#68119,#68120,#68121,#68122,#68123,#68124,#68125,#68126,#68127,#68128,
#68129,#68130,#68131,#68132,#68133,#68134,#68135,#68136,#68137,#68138,#68139,
#68140,#68141,#68142,#68143,#68144,#68145,#68146,#68147,#68148,#68149,#68150,
#68151,#68152,#68153,#68154,#68155,#68156,#68157,#68158,#68159,#68160,#68161,
#68162,#68163,#68164,#68165,#68166,#68167,#68168,#68169,#68170,#68171,#68172,
#68173,#68174,#68175,#68176,#68177,#68178,#68179,#68180,#68181,#68182,#68183,
#68184,#68185,#68186,#68187,#68188,#68189,#68190,#68191,#68192,#68193,#68194,
#68195,#68196,#68197,#68198,#68199,#68200,#68201,#68202,#68203,#68204,#68205,
#68206,#68207,#68208,#68209,#68210,#68211,#68212,#68213,#68214,#68215,#68216,
#68217,#68218,#68219,#68220,#68221,#68222,#68223,#68224,#68225,#68226,#68227,
#68228,#68229,#68230,#68231,#68232,#68233,#68234,#68235,#68236,#68237,#68238,
#68239,#68240,#68241,#68242,#68243,#68244,#68245,#68246,#68247,#68248,#68249,
#68250,#68251,#68252,#68253,#68254,#68255,#68256,#68257,#68258,#68259,#68260,
#68261,#68262,#68263,#68264,#68265,#68266,#68267,#68268,#68269,#68270,#68271,
#68272,#68273,#68274,#68275,#68276,#68277,#68278,#68279,#68280,#68281,#68282,
#68283,#68284,#68285,#68286,#68287,#68288,#68289,#68290,#68291,#68292,#68293,
#68294,#68295,#68296,#68297,#68298,#68299,#68300,#68301,#68302,#68303,#68304,
#68305,#68306,#68307,#68308,#68309,#68310,#68311,#68312,#68313,#68314,#68315,
#68316,#68317,#68318,#68319,#68320,#68321,#68322,#68323,#68324,#68325,#68326,
#68327,#68328,#68329,#68330,#68331,#68332),.UNSPECIFIED.,.F.,.F.,(4,2,2,
2,2,2,2,2,2,2,2,2,2,2,2,2,2,2,2,2,2,2,2,2,2,2,2,2,2,2,2,2,2,2,2,2,2,2,2,
2,2,2,2,2,2,2,2,2,2,2,2,2,2,2,2,2,2,2,2,2,2,2,2,2,2,2,2,2,2,2,2,2,2,2,2,
2,2,2,2,2,2,2,2,2,2,2,2,2,2,2,2,2,2,2,2,2,2,2,2,2,2,2,2,2,2,2,2,2,2,4),
(-2.65746774305231,-2.65261804205566,-2.64584623324261,-2.62617272996607,
-2.615158715998,-2.61180870310401,-2.60969057770515,-2.60767078381733,-2.60516685459269,
-2.59894220127053,-2.56240086795725,-2.52983407927815,-2.5025163264511,
-2.4959566011589,-2.49203172690838,-2.48850786796351,-2.48400238850228,
-2.47461125209531,-2.42156657618331,-2.40828353613625,-2.38883638532185,
-2.37790572301896,-2.37456456956123,-2.37244832301837,-2.37042708978095,
-2.36791799108521,-2.36166341956384,-2.3255746626612,-2.2936985406124,-2.26539500955471,
-2.25877237795713,-2.25483372512526,-2.25131232252042,-2.24683034551568,
-2.23756365834511,-2.18277827436322,-2.17137556262963,-2.1516918972459,
-2.14067375523214,-2.13732307541338,-2.13520466037621,-2.13318470453986,
-2.13068069407162,-2.12445643857931,-2.08788702671947,-2.0551634332501,
-2.02799948587829,-2.02144936529857,-2.0175263187276,-2.01400164189302,
-2.00949171294237,-2.00007853200098,-1.94738375203425,-1.91806825964147,
-1.90862556174804,-1.90207648863689,-1.89932450422995,-1.89732548159356,
-1.89511670599879,-1.89135670056093,-1.87751250941603,-1.86804159384396,
-1.82509180481262,-1.79421630215818,-1.78565730401293,-1.78131308838638,
-1.77780387481513,-1.77377471181276,-1.76691604016749,-1.73688615852472,
-1.68578013459207,-1.66727315857274,-1.66332871016514,-1.66107944988934,
-1.6590919804408,-1.65646702327566,-1.65048992885583,-1.60317010610248,
-1.55639897987041,-1.54815030595161,-1.54386836370732,-1.54036272421504,
-1.53628518103136,-1.5292125310971,-1.49473056438907,-1.46722289421195,
-1.46251149378335,-1.43097650505498,-1.4269038680685,-1.42438472433374,
-1.42241262300298,-1.42006456128484,-1.41565919958629,-1.38460982826758,
-1.33569511012369,-1.31546921485392,-1.30927375427337,-1.30542774023406,
-1.30188303067876,-1.29721857384015,-1.28696539389295,-1.27301799952048,
-1.20017970924618,-1.19119696202027,-1.18798359961284,-1.1861022609768,
-1.18407387501954,-1.18115436225658,-1.17354740652748,-1.16365104910194),
 .UNSPECIFIED.);
#960=B_SPLINE_CURVE_WITH_KNOTS('',3,(#68333,#68334,#68335,#68336,#68337,
#68338,#68339,#68340,#68341,#68342,#68343,#68344,#68345,#68346,#68347,#68348,
#68349,#68350,#68351,#68352,#68353,#68354,#68355,#68356,#68357,#68358,#68359,
#68360,#68361,#68362,#68363,#68364,#68365,#68366,#68367,#68368,#68369,#68370,
#68371,#68372,#68373,#68374,#68375,#68376,#68377,#68378,#68379,#68380,#68381,
#68382,#68383,#68384,#68385,#68386,#68387,#68388,#68389,#68390,#68391,#68392,
#68393,#68394,#68395,#68396,#68397,#68398,#68399,#68400,#68401,#68402,#68403,
#68404,#68405,#68406,#68407,#68408,#68409,#68410,#68411,#68412,#68413,#68414,
#68415,#68416,#68417,#68418,#68419,#68420,#68421,#68422,#68423,#68424,#68425,
#68426,#68427,#68428,#68429,#68430,#68431,#68432,#68433,#68434,#68435,#68436,
#68437,#68438,#68439,#68440,#68441,#68442,#68443,#68444,#68445,#68446,#68447,
#68448,#68449,#68450,#68451,#68452,#68453,#68454,#68455,#68456,#68457,#68458,
#68459,#68460,#68461,#68462,#68463,#68464,#68465,#68466,#68467,#68468,#68469,
#68470,#68471,#68472,#68473,#68474,#68475,#68476,#68477,#68478,#68479,#68480,
#68481,#68482,#68483,#68484,#68485,#68486,#68487,#68488,#68489,#68490,#68491,
#68492,#68493,#68494,#68495,#68496,#68497,#68498,#68499,#68500,#68501,#68502,
#68503,#68504,#68505,#68506,#68507,#68508,#68509,#68510,#68511,#68512,#68513,
#68514,#68515,#68516,#68517,#68518,#68519,#68520,#68521,#68522,#68523,#68524,
#68525,#68526,#68527,#68528,#68529,#68530,#68531,#68532,#68533,#68534,#68535,
#68536,#68537,#68538,#68539,#68540,#68541,#68542,#68543,#68544),
 .UNSPECIFIED.,.F.,.F.,(4,2,2,2,2,2,2,2,2,2,2,2,2,2,2,2,2,2,2,2,2,2,2,2,
2,2,2,2,2,2,2,2,2,2,2,2,2,2,2,2,2,2,2,2,2,2,2,2,2,2,2,2,2,2,2,2,2,2,2,2,
2,2,2,2,2,2,2,2,2,2,2,2,2,2,2,2,2,2,2,2,2,2,2,2,2,2,2,2,2,2,2,2,2,2,2,2,
2,2,2,2,2,2,2,2,2,4),(-1.82625073863295,-1.81743048083367,-1.76819131431197,
-1.7370057602039,-1.73259681582595,-1.73024795135637,-1.72827585061212,
-1.72575766004703,-1.72168845751425,-1.69070653630609,-1.65995402162083,
-1.63551189232338,-1.6251599607778,-1.61701484637726,-1.61275381803255,
-1.60958890756908,-1.60561783324043,-1.59884743904035,-1.57172333339439,
-1.57012941610718,-1.5175731179029,-1.49886167212502,-1.49490514287303,
-1.49265312027545,-1.49066610548489,-1.48799963132586,-1.48194934058225,
-1.47345024551375,-1.44894084451354,-1.38857164734317,-1.3800187117489,
-1.37561883703829,-1.3721049547582,-1.36811401181362,-1.36125184949231,
-1.3285933809597,-1.28218877469639,-1.26188622135384,-1.25772928959791,
-1.25540878585404,-1.25343370313395,-1.25087701062807,-1.24542761236607,
-1.23801716266803,-1.21834663865769,-1.20682946572698,-1.15215376976889,
-1.14287592453066,-1.13839133487293,-1.13486912035124,-1.1309308663737,
-1.12431214512924,-1.09609335014294,-1.06409684036266,-1.02791937825338,
-1.02166335560134,-1.01915371437839,-1.0171320839256,-1.01501548487916,
-1.01167399187847,-1.0007439690132,-0.98130423258884,-0.968028781115128,
-0.914962610035953,-0.905570343790112,-0.901064113184676,-0.897539589849428,
-0.893613914261244,-0.887052774060993,-0.859734433934364,-0.827109429478095,
-0.790514602968309,-0.784285731805667,-0.781780760959654,-0.779760412203886,
-0.777642073798023,-0.774292473562495,-0.763286511599889,-0.743640856571713,
-0.731864035548962,-0.677451036256476,-0.668153166831811,-0.663664940887641,
-0.660142527666568,-0.65620680828103,-0.649599014408321,-0.621550080724126,
-0.589434878029331,-0.553184169763361,-0.546934358455406,-0.544425868211862,
-0.542404632110245,-0.54028778475524,-0.536944751713608,-0.525999154515777,
-0.506516698972738,-0.493440679296154,-0.440228348932964,-0.430846043315784,
-0.426341876093813,-0.422817783558311,-0.418891368708921,-0.412326071473523,
-0.384939270089989,-0.352363406606311,-0.33180592744104),.UNSPECIFIED.);
#961=B_SPLINE_CURVE_WITH_KNOTS('',3,(#68550,#68551,#68552,#68553,#68554,
#68555,#68556,#68557,#68558,#68559,#68560,#68561,#68562,#68563,#68564,#68565,
#68566,#68567,#68568,#68569,#68570,#68571,#68572,#68573,#68574,#68575,#68576,
#68577,#68578,#68579,#68580,#68581,#68582,#68583,#68584,#68585,#68586,#68587,
#68588,#68589,#68590,#68591,#68592,#68593,#68594,#68595,#68596,#68597,#68598,
#68599,#68600,#68601,#68602,#68603,#68604,#68605,#68606,#68607,#68608,#68609,
#68610,#68611,#68612,#68613,#68614,#68615,#68616,#68617,#68618,#68619,#68620,
#68621,#68622,#68623,#68624,#68625,#68626,#68627,#68628,#68629,#68630,#68631,
#68632,#68633,#68634,#68635,#68636,#68637,#68638,#68639,#68640,#68641,#68642,
#68643,#68644,#68645,#68646,#68647,#68648,#68649,#68650,#68651,#68652,#68653,
#68654,#68655,#68656,#68657,#68658,#68659,#68660,#68661,#68662,#68663,#68664,
#68665,#68666,#68667,#68668,#68669,#68670,#68671,#68672,#68673,#68674,#68675,
#68676,#68677,#68678,#68679,#68680,#68681,#68682,#68683,#68684,#68685,#68686,
#68687,#68688,#68689,#68690,#68691,#68692,#68693,#68694,#68695,#68696,#68697,
#68698,#68699,#68700,#68701,#68702,#68703,#68704,#68705,#68706,#68707,#68708,
#68709,#68710,#68711,#68712,#68713,#68714,#68715,#68716,#68717,#68718,#68719,
#68720,#68721,#68722,#68723,#68724,#68725,#68726,#68727,#68728,#68729),
 .UNSPECIFIED.,.F.,.F.,(4,2,2,2,2,2,2,2,2,2,2,2,2,2,2,2,2,2,2,2,2,2,2,2,
2,2,2,2,2,2,2,2,2,2,2,2,2,2,2,2,2,2,2,2,2,2,2,2,2,2,2,2,2,2,2,2,2,2,2,2,
2,2,2,2,2,2,2,2,2,2,2,2,2,2,2,2,2,2,2,2,2,2,2,2,2,2,2,2,2,4),(-1.16363369234352,
-1.16295790678583,-1.15898823988006,-1.15222521336478,-1.12151620897351,
-1.0914958340154,-1.07796261271634,-1.05309843885021,-1.04911505999603,
-1.04662240929076,-1.04465156623561,-1.04228158322413,-1.0377723225715,
-0.999306261595195,-0.942744148510771,-0.933643853752399,-0.929193356432228,
-0.925674754874985,-0.921716221149426,-0.915003741001527,-0.885201841163423,
-0.854535777790885,-0.848020169730516,-0.815955518207676,-0.811881134326602,
-0.809361399704959,-0.807389161869915,-0.805041325635805,-0.800637404062841,
-0.769667244373821,-0.720955423652076,-0.700490299246686,-0.694268838917962,
-0.69041704342088,-0.686873898821883,-0.682221590823078,-0.672037005029608,
-0.658212364211504,-0.587646533901273,-0.576690947281024,-0.573223401629135,
-0.57107887319902,-0.569050507351872,-0.566131347764967,-0.558527132688328,
-0.54697430039157,-0.503767844145718,-0.465050987403647,-0.457868502874748,
-0.453765792591738,-0.450294235154145,-0.446055437065266,-0.438020902376893,
-0.398980220917527,-0.359911337502345,-0.340637027524395,-0.33653319357697,
-0.334224483342421,-0.332266412336735,-0.32970263543321,-0.32421663468579,
-0.316741411562477,-0.296800924411448,-0.257284792886249,-0.227183245499586,
-0.220308635565535,-0.216275186853487,-0.212922047147884,-0.212799261089963,
-0.212686912750328,-0.212583554354981,-0.212487997172239,-0.212399255293022,
-0.212316503547186,-0.212239045552849,-0.212166289148202,-0.21209772728177,
-0.207829510722542,-0.202892439011164,-0.194675785088698,-0.177398604672938,
-0.107522448590471,-0.10071895347576,-0.0981229310198588,-0.0962616113804328,
-0.0942146686741461,-0.0912019036092385,-0.0829525861352058,-0.0700249612576247,
-0.000702836714805313),.UNSPECIFIED.);
#962=B_SPLINE_CURVE_WITH_KNOTS('',3,(#68730,#68731,#68732,#68733,#68734,
#68735,#68736,#68737,#68738,#68739,#68740,#68741,#68742,#68743,#68744,#68745,
#68746,#68747,#68748,#68749,#68750,#68751,#68752,#68753,#68754,#68755,#68756,
#68757,#68758,#68759,#68760,#68761,#68762,#68763,#68764,#68765,#68766,#68767,
#68768,#68769,#68770,#68771,#68772,#68773,#68774,#68775,#68776,#68777,#68778,
#68779,#68780,#68781,#68782,#68783),.UNSPECIFIED.,.F.,.F.,(4,2,2,2,2,2,
2,2,2,2,2,2,2,2,2,2,2,2,2,2,2,2,2,2,2,2,4),(-2.98872595129121,-2.97578488693837,
-2.97135777031141,-2.96792934948171,-2.96453074422925,-2.96066679337635,
-2.95438691435237,-2.93333516725447,-2.89683441943583,-2.86718109747591,
-2.85767739453118,-2.85109695767192,-2.8483400404559,-2.84634053495174,
-2.84413463115462,-2.84038652557546,-2.82667029217726,-2.81346715947534,
-2.76270086129221,-2.74713932280744,-2.73949074450365,-2.7331382232944,
-2.72930337547387,-2.72596856016156,-2.72157180516364,-2.71303000503505,
-2.65746774305231),.UNSPECIFIED.);
#963=B_SPLINE_CURVE_WITH_KNOTS('',3,(#68785,#68786,#68787,#68788,#68789,
#68790,#68791,#68792,#68793,#68794,#68795,#68796,#68797,#68798,#68799,#68800,
#68801,#68802,#68803,#68804,#68805,#68806,#68807,#68808,#68809,#68810,#68811,
#68812,#68813,#68814,#68815,#68816,#68817,#68818,#68819,#68820,#68821,#68822,
#68823,#68824,#68825,#68826,#68827,#68828,#68829,#68830,#68831,#68832,#68833,
#68834,#68835,#68836,#68837,#68838,#68839,#68840,#68841,#68842,#68843,#68844,
#68845,#68846),.UNSPECIFIED.,.F.,.F.,(4,2,2,2,2,2,2,2,2,2,2,2,2,2,2,2,2,
2,2,2,2,2,2,2,2,2,2,2,2,2,4),(-0.33180592744104,-0.315805296192904,-0.30957522893432,
-0.307070148343933,-0.305049859303639,-0.302931767633533,-0.299582878262543,
-0.288582218983313,-0.268950293727248,-0.223440144617194,-0.198289806895859,
-0.191646535975279,-0.187703225161834,-0.184182389210223,-0.184091452403489,
-0.184007491759481,-0.183929715066348,-0.183857446652311,-0.183790106661967,
-0.179513058052387,-0.170230254477495,-0.157798514338694,-0.124947258169611,
-0.0779185224010441,-0.071920600512571,-0.0692920138102425,-0.067304111089287,
-0.0650570519110233,-0.0611225601528712,-0.0562441162046279,-0.000702637539615483),
 .UNSPECIFIED.);
#964=B_SPLINE_CURVE_WITH_KNOTS('',3,(#68847,#68848,#68849,#68850,#68851,
#68852,#68853,#68854,#68855,#68856,#68857,#68858,#68859,#68860,#68861,#68862,
#68863,#68864,#68865,#68866,#68867,#68868,#68869,#68870,#68871,#68872,#68873,
#68874,#68875,#68876,#68877,#68878,#68879,#68880,#68881,#68882,#68883,#68884,
#68885,#68886,#68887,#68888,#68889,#68890,#68891,#68892,#68893,#68894,#68895,
#68896,#68897,#68898,#68899,#68900,#68901,#68902,#68903,#68904,#68905,#68906,
#68907,#68908,#68909,#68910,#68911,#68912,#68913,#68914,#68915,#68916,#68917,
#68918,#68919,#68920,#68921,#68922,#68923,#68924,#68925,#68926,#68927,#68928,
#68929,#68930,#68931,#68932,#68933,#68934,#68935,#68936,#68937,#68938,#68939,
#68940,#68941,#68942,#68943,#68944,#68945,#68946,#68947,#68948,#68949,#68950,
#68951,#68952,#68953,#68954,#68955,#68956,#68957,#68958,#68959,#68960,#68961,
#68962,#68963,#68964,#68965,#68966,#68967,#68968,#68969,#68970,#68971,#68972,
#68973,#68974,#68975,#68976,#68977,#68978,#68979,#68980,#68981,#68982,#68983,
#68984,#68985,#68986,#68987,#68988,#68989,#68990,#68991,#68992,#68993,#68994,
#68995,#68996,#68997,#68998,#68999,#69000,#69001,#69002,#69003,#69004,#69005,
#69006,#69007,#69008,#69009,#69010,#69011,#69012,#69013,#69014,#69015,#69016,
#69017,#69018,#69019,#69020,#69021,#69022,#69023,#69024,#69025,#69026,#69027,
#69028,#69029,#69030,#69031,#69032,#69033,#69034,#69035,#69036),
 .UNSPECIFIED.,.F.,.F.,(4,2,2,2,2,2,2,2,2,2,2,2,2,2,2,2,2,2,2,2,2,2,2,2,
2,2,2,2,2,2,2,2,2,2,2,2,2,2,2,2,2,2,2,2,2,2,2,2,2,2,2,2,2,2,2,2,2,2,2,2,
2,2,2,2,2,2,2,2,2,2,2,2,2,2,2,2,2,2,2,2,2,2,2,2,2,2,2,2,2,2,2,2,2,2,4),
(-2.98905990044328,-2.95356430823409,-2.94714927655617,-2.94294742412976,
-2.93958726252696,-2.93642035663075,-2.93247526267118,-2.92581920350916,
-2.90044284942758,-2.87218225969175,-2.83060653310438,-2.82352687778292,
-2.82064631723278,-2.81862606589344,-2.81673656311586,-2.81347769259623,
-2.80415918418035,-2.7576997624601,-2.7277905846504,-2.7160400495557,-2.70712101398718,
-2.7028506940356,-2.70281464991139,-2.70277684132149,-2.70273717109788,
-2.70269553584728,-2.70265182547647,-2.70260592270797,-2.70255770254141,
-2.7025070316726,-2.70245376787538,-2.69894590063035,-2.69491914062542,
-2.68806671512818,-2.65812725990795,-2.61794577478734,-2.59830842794534,
-2.58730814182006,-2.58396012805575,-2.58184279810661,-2.57982339578818,
-2.57731961897877,-2.5710937022775,-2.53458065956312,-2.50205664648718,
-2.47466666310888,-2.46810324453046,-2.46417821058729,-2.46065551227561,
-2.45615334249306,-2.44677607040895,-2.39350809743223,-2.38051082805457,
-2.36099740625163,-2.35004264717796,-2.3466994201717,-2.34458307379871,
-2.34256283750361,-2.34005617094636,-2.33381372445072,-2.29756491818998,
-2.26543748373493,-2.23747517261891,-2.23087486133189,-2.22694169388657,
-2.22342037326959,-2.21893190459706,-2.20962754530034,-2.1553123885653,
-2.1434364330009,-2.12378815647395,-2.112783461603,-2.10943475344116,-2.10731712971016,
-2.10529757302389,-2.10279373648018,-2.09656833243039,-2.06002683241007,
-2.02734362059603,-2.00010997057961,-1.99355628585345,-1.98963311096651,
-1.98610959762098,-1.9816029511122,-1.97220348671927,-1.91927345342404,
-1.90574678403011,-1.88638187126658,-1.87548174853486,-1.8721442025444,
-1.87002896382351,-1.86800762120678,-1.86549731430977,-1.85923432920162,
-1.82631764215159),.UNSPECIFIED.);
#965=B_SPLINE_CURVE_WITH_KNOTS('',3,(#69041,#69042,#69043,#69044,#69045,
#69046,#69047,#69048,#69049,#69050,#69051,#69052,#69053,#69054,#69055,#69056,
#69057,#69058,#69059,#69060,#69061,#69062,#69063,#69064,#69065,#69066,#69067,
#69068,#69069,#69070,#69071,#69072,#69073,#69074,#69075,#69076,#69077,#69078,
#69079,#69080,#69081,#69082,#69083,#69084,#69085,#69086,#69087,#69088,#69089,
#69090,#69091,#69092,#69093,#69094,#69095,#69096,#69097,#69098,#69099,#69100,
#69101,#69102,#69103,#69104,#69105,#69106,#69107,#69108,#69109,#69110,#69111,
#69112,#69113,#69114,#69115,#69116,#69117,#69118,#69119,#69120,#69121,#69122,
#69123,#69124,#69125,#69126,#69127,#69128,#69129,#69130,#69131,#69132,#69133,
#69134,#69135,#69136,#69137,#69138,#69139,#69140,#69141,#69142,#69143,#69144,
#69145,#69146,#69147,#69148,#69149,#69150,#69151,#69152,#69153,#69154,#69155,
#69156,#69157,#69158,#69159,#69160,#69161,#69162,#69163,#69164,#69165,#69166,
#69167,#69168,#69169,#69170,#69171,#69172,#69173,#69174,#69175,#69176,#69177,
#69178,#69179,#69180,#69181,#69182,#69183,#69184,#69185,#69186,#69187,#69188,
#69189,#69190,#69191,#69192,#69193,#69194,#69195,#69196,#69197,#69198,#69199,
#69200,#69201,#69202,#69203,#69204,#69205,#69206,#69207,#69208,#69209,#69210,
#69211,#69212,#69213,#69214,#69215,#69216,#69217,#69218,#69219,#69220,#69221,
#69222,#69223,#69224,#69225,#69226,#69227,#69228,#69229,#69230,#69231,#69232,
#69233,#69234,#69235,#69236,#69237,#69238,#69239,#69240,#69241,#69242,#69243,
#69244,#69245,#69246,#69247,#69248,#69249,#69250),.UNSPECIFIED.,.F.,.F.,
(4,2,2,2,2,2,2,2,2,2,2,2,2,2,2,2,2,2,2,2,2,2,2,2,2,2,2,2,2,2,2,2,2,2,2,
2,2,2,2,2,2,2,2,2,2,2,2,2,2,2,2,2,2,2,2,2,2,2,2,2,2,2,2,2,2,2,2,2,2,2,2,
2,2,2,2,2,2,2,2,2,2,2,2,2,2,2,2,2,2,2,2,2,2,2,2,2,2,2,2,2,2,2,2,2,4),(-2.6576697293675,
-2.62693356030965,-2.59963849603588,-2.59307946384318,-2.58915432577582,
-2.58562980474747,-2.58112289068937,-2.57172656090521,-2.51873274140474,
-2.48961858642228,-2.48021271551229,-2.47368269100481,-2.47093379075845,
-2.46893514628557,-2.46672473782423,-2.46295770961296,-2.44903636057712,
-2.43954294382804,-2.39436598165337,-2.36281043950389,-2.35600381304448,
-2.35202498359897,-2.34850960811236,-2.34409166081447,-2.33545163989856,
-2.27577310478329,-2.25085890700078,-2.23806197693863,-2.23453475396773,
-2.23237720420162,-2.23037924308025,-2.22796302615207,-2.22182444982963,
-2.17736848466244,-2.14290057013905,-2.13011709390181,-2.12052339222402,
-2.11597916116625,-2.11244999659881,-2.10854468958577,-2.10207793278101,
-2.07920785943265,-2.03232312870307,-2.01180635265277,-2.00048504251354,
-1.99710191148193,-1.99497609620949,-1.99296031424258,-1.99047317134783,
-1.98434861621092,-1.94257217718088,-1.89025929208093,-1.88225382280685,
-1.87802128220995,-1.87455031213367,-1.87044296804023,-1.86323859252951,
-1.81779630197473,-1.78212141129576,-1.76415924880125,-1.76024667591471,
-1.75800423330561,-1.75601480347933,-1.7533768933276,-1.7473267197513,-1.70154696723194,
-1.66792529726364,-1.65532409981282,-1.64583566378124,-1.64131107444241,
-1.63778416204394,-1.63386807193642,-1.62735205102452,-1.60381133978621,
-1.55276607090862,-1.53560612823849,-1.52882308708679,-1.52373322947704,
-1.521245662974,-1.51946507544915,-1.51717209842833,-1.51313743318411,-1.49504714805063,
-1.4450067163768,-1.41388150306682,-1.40696678787983,-1.40292451817069,
-1.39941582134603,-1.39508757850367,-1.38661091855988,-1.35633736598825,
-1.30995296866614,-1.29001898432536,-1.28588066376219,-1.28356424957872,
-1.28158848375927,-1.27902543211187,-1.27354285316252,-1.26607358491697,
-1.24615740771257,-1.23867188706878,-1.17962157045517,-1.17090847983914,
-1.16647506272123,-1.16363369234352),.UNSPECIFIED.);
#966=B_SPLINE_CURVE_WITH_KNOTS('',3,(#69251,#69252,#69253,#69254,#69255,
#69256,#69257,#69258,#69259,#69260,#69261,#69262,#69263,#69264,#69265,#69266,
#69267,#69268,#69269,#69270,#69271,#69272,#69273,#69274,#69275,#69276,#69277,
#69278,#69279,#69280,#69281,#69282,#69283,#69284,#69285,#69286,#69287,#69288,
#69289,#69290,#69291,#69292,#69293,#69294,#69295,#69296,#69297,#69298,#69299,
#69300,#69301,#69302,#69303,#69304,#69305,#69306,#69307,#69308,#69309,#69310,
#69311,#69312,#69313,#69314,#69315,#69316,#69317,#69318,#69319,#69320,#69321,
#69322,#69323,#69324,#69325,#69326,#69327,#69328,#69329,#69330,#69331,#69332,
#69333,#69334,#69335,#69336,#69337,#69338,#69339,#69340,#69341,#69342,#69343,
#69344,#69345,#69346,#69347,#69348,#69349,#69350,#69351,#69352,#69353,#69354,
#69355,#69356,#69357,#69358,#69359,#69360,#69361,#69362,#69363,#69364,#69365,
#69366,#69367,#69368,#69369,#69370,#69371,#69372,#69373,#69374,#69375,#69376,
#69377,#69378,#69379,#69380,#69381,#69382,#69383,#69384,#69385,#69386,#69387,
#69388,#69389,#69390,#69391,#69392,#69393,#69394,#69395,#69396,#69397,#69398,
#69399,#69400,#69401,#69402,#69403,#69404,#69405,#69406,#69407,#69408,#69409,
#69410,#69411,#69412,#69413,#69414,#69415,#69416,#69417,#69418,#69419,#69420,
#69421,#69422,#69423,#69424,#69425,#69426,#69427,#69428,#69429,#69430,#69431,
#69432,#69433,#69434,#69435,#69436,#69437,#69438,#69439,#69440,#69441,#69442,
#69443,#69444,#69445,#69446,#69447,#69448,#69449,#69450,#69451,#69452,#69453,
#69454,#69455,#69456,#69457,#69458,#69459,#69460,#69461,#69462,#69463,#69464),
 .UNSPECIFIED.,.F.,.F.,(4,2,2,2,2,2,2,2,2,2,2,2,2,2,2,2,2,2,2,2,2,2,2,2,
2,2,2,2,2,2,2,2,2,2,2,2,2,2,2,2,2,2,2,2,2,2,2,2,2,2,2,2,2,2,2,2,2,2,2,2,
2,2,2,2,2,2,2,2,2,2,2,2,2,2,2,2,2,2,2,2,2,2,2,2,2,2,2,2,2,2,2,2,2,2,2,2,
2,2,2,2,2,2,2,2,2,2,4),(-1.82631764215159,-1.82323974212304,-1.79152376162018,
-1.76298270207981,-1.75634601678174,-1.75240470270774,-1.7488844669152,
-1.74440884748864,-1.73517333886562,-1.68030290659254,-1.66893018834484,
-1.64923526092079,-1.63821301849764,-1.63486220669421,-1.63274397836327,
-1.63072447281904,-1.62822135636435,-1.62200103721747,-1.58529636144442,
-1.55240489308472,-1.53457520866803,-1.52225548237389,-1.51724535046799,
-1.5136442226595,-1.51035968068673,-1.50593724067268,-1.49502235607148,
-1.46641734018428,-1.41376880896186,-1.40143651065848,-1.39781812808716,
-1.39564074228537,-1.39362991864508,-1.39080498538834,-1.38380786990236,
-1.37348959983616,-1.33905515883292,-1.29336992537318,-1.28372885815686,
-1.27922518629899,-1.27569230725627,-1.27180675209643,-1.26542817952572,
-1.24069225165136,-1.21145855783858,-1.16831607828925,-1.16271586727901,
-1.15977174715401,-1.15775926294019,-1.1556295362013,-1.15222711975135,
-1.14071368640189,-1.11965761476887,-1.07149671322946,-1.05038166234853,
-1.04408730632017,-1.04022007618033,-1.03668228958125,-1.03206536782902,
-1.02207402192909,-1.00859207388014,-0.970698662292824,-0.931210051675819,
-0.925002414273407,-0.922501318435399,-0.9204822266186,-0.918362882974066,
-0.915007637560058,-0.903945438473393,-0.884144897893716,-0.87447230987607,
-0.817879517185717,-0.808781412387799,-0.804331924231257,-0.800814120046543,
-0.796856502207348,-0.790145679118282,-0.760357682053604,-0.729674442472779,
-0.723479132630582,-0.691080046457897,-0.687005713714386,-0.684486280566667,
-0.682514476102601,-0.680167455892698,-0.675765919938365,-0.644881191381222,
-0.59639145952434,-0.575658933696101,-0.569408308775917,-0.565550734919029,
-0.562010421665312,-0.557373719609624,-0.547272360132232,-0.533595227739597,
-0.465426385481745,-0.452249073871324,-0.448548758491545,-0.446353157148726,
-0.444349470748219,-0.44156802406071,-0.434840934298955,-0.425054789053505,
-0.393819644382117,-0.343853452397251,-0.334314329759046,-0.33219634213793),
 .UNSPECIFIED.);
#967=B_SPLINE_CURVE_WITH_KNOTS('',3,(#69470,#69471,#69472,#69473,#69474,
#69475,#69476,#69477,#69478,#69479,#69480,#69481,#69482,#69483,#69484,#69485,
#69486,#69487,#69488,#69489,#69490,#69491,#69492,#69493,#69494,#69495,#69496,
#69497,#69498,#69499,#69500,#69501,#69502,#69503,#69504,#69505,#69506,#69507,
#69508,#69509,#69510,#69511,#69512,#69513,#69514,#69515,#69516,#69517,#69518,
#69519,#69520,#69521,#69522,#69523,#69524,#69525,#69526,#69527,#69528,#69529,
#69530,#69531,#69532,#69533,#69534,#69535,#69536,#69537,#69538,#69539,#69540,
#69541,#69542,#69543,#69544,#69545,#69546,#69547,#69548,#69549,#69550,#69551,
#69552,#69553,#69554,#69555,#69556,#69557,#69558,#69559,#69560,#69561,#69562,
#69563,#69564,#69565,#69566,#69567,#69568,#69569,#69570,#69571,#69572,#69573,
#69574,#69575,#69576,#69577,#69578,#69579,#69580,#69581,#69582,#69583,#69584,
#69585,#69586,#69587,#69588,#69589,#69590,#69591,#69592,#69593,#69594,#69595,
#69596,#69597,#69598,#69599,#69600,#69601,#69602,#69603,#69604,#69605,#69606,
#69607,#69608,#69609,#69610,#69611,#69612,#69613,#69614,#69615,#69616,#69617,
#69618,#69619,#69620,#69621,#69622,#69623,#69624,#69625,#69626,#69627,#69628,
#69629,#69630,#69631,#69632,#69633,#69634,#69635,#69636,#69637,#69638,#69639),
 .UNSPECIFIED.,.F.,.F.,(4,2,2,2,2,2,2,2,2,2,2,2,2,2,2,2,2,2,2,2,2,2,2,2,
2,2,2,2,2,2,2,2,2,2,2,2,2,2,2,2,2,2,2,2,2,2,2,2,2,2,2,2,2,2,2,2,2,2,2,2,
2,2,2,2,2,2,2,2,2,2,2,2,2,2,2,2,2,2,2,2,2,2,2,2,4),(-1.16381432242618,-1.15034453016281,
-1.14631361253183,-1.14380639924013,-1.1418343141596,-1.13947512224484,
-1.13501933608295,-1.10126307762493,-1.0452562761488,-1.03269120026321,
-1.02750312689733,-1.02423060693756,-1.02061422553913,-1.01552903802334,
-1.00273318698385,-0.983952151595484,-0.952057083173095,-0.915945783339466,
-0.909684730090513,-0.907173882166337,-0.905151596850594,-0.903034654707083,
-0.899693143534105,-0.888767569158273,-0.869340850180665,-0.856065961602515,
-0.802992184677781,-0.793600653706283,-0.789093910665508,-0.785568581601447,
-0.781641572301792,-0.775077103363844,-0.747722473777219,-0.715128091659899,
-0.6785584465486,-0.672328478162737,-0.669822970196079,-0.667802145157618,
-0.66568320272998,-0.662332394461906,-0.651319826716066,-0.631657243601803,
-0.620145463170004,-0.565471201201982,-0.556194577841849,-0.55170975195013,
-0.548186959735666,-0.544247633236188,-0.537626020356028,-0.509371007157941,
-0.477410593962117,-0.441245410368045,-0.434998076656561,-0.432489660282702,
-0.430468112729463,-0.428350427699331,-0.425005112437636,-0.414042930755737,
-0.394516619777133,-0.354898625088743,-0.324321711259594,-0.317434046355778,
-0.31339760889738,-0.309887953821573,-0.305550787110016,-0.297030998979092,
-0.266448197437599,-0.238090252622209,-0.203906000392167,-0.197684221561562,
-0.195180178397643,-0.19315980353295,-0.191040424325782,-0.187904420915456,
-0.178134655517359,-0.161526159435422,-0.127555530489142,-0.0875799587176907,
-0.0803823977286344,-0.0762762174834137,-0.0728046715442998,-0.0685695107018069,
-0.0605531604702257,-0.0504090877965985,-0.000702609627408209),
 .UNSPECIFIED.);
#968=B_SPLINE_CURVE_WITH_KNOTS('',3,(#69640,#69641,#69642,#69643,#69644,
#69645,#69646,#69647,#69648,#69649,#69650,#69651,#69652,#69653,#69654,#69655,
#69656,#69657,#69658,#69659,#69660,#69661,#69662,#69663,#69664,#69665,#69666,
#69667,#69668,#69669,#69670,#69671,#69672,#69673,#69674,#69675,#69676,#69677,
#69678,#69679,#69680,#69681,#69682,#69683,#69684,#69685,#69686,#69687,#69688,
#69689,#69690,#69691,#69692,#69693),.UNSPECIFIED.,.F.,.F.,(4,2,2,2,2,2,
2,2,2,2,2,2,2,2,2,2,2,2,2,2,2,2,2,2,2,2,4),(-2.98863346158678,-2.95253752221994,
-2.94897276709526,-2.94663648454277,-2.94476052864309,-2.94278912902029,
-2.94027942844017,-2.93623823846993,-2.90733953023107,-2.8748582676774,
-2.84132911968313,-2.83243581119988,-2.82788190376301,-2.82435205343567,
-2.82045290143933,-2.8140125313558,-2.79167428337775,-2.73689658821841,
-2.72132198789988,-2.7119512193783,-2.70895448893227,-2.70683556543818,
-2.70481573709573,-2.70231252513109,-2.69609346536451,-2.65952388738373,
-2.6576697293675),.UNSPECIFIED.);
#969=B_SPLINE_CURVE_WITH_KNOTS('',3,(#69695,#69696,#69697,#69698,#69699,
#69700,#69701,#69702,#69703,#69704,#69705,#69706,#69707,#69708,#69709,#69710,
#69711,#69712,#69713,#69714,#69715,#69716,#69717,#69718,#69719,#69720,#69721,
#69722,#69723,#69724,#69725,#69726,#69727,#69728,#69729,#69730,#69731,#69732,
#69733,#69734,#69735,#69736,#69737,#69738,#69739,#69740,#69741,#69742,#69743,
#69744,#69745,#69746,#69747,#69748,#69749,#69750,#69751,#69752,#69753,#69754,
#69755,#69756,#69757,#69758,#69759,#69760,#69761,#69762,#69763,#69764,#69765,
#69766,#69767,#69768,#69769,#69770,#69771,#69772,#69773,#69774,#69775,#69776,
#69777,#69778,#69779,#69780,#69781,#69782,#69783,#69784,#69785,#69786,#69787,
#69788,#69789,#69790,#69791,#69792,#69793,#69794,#69795,#69796,#69797,#69798),
 .UNSPECIFIED.,.F.,.F.,(4,2,2,2,2,2,2,2,2,2,2,2,2,2,2,2,2,2,2,2,2,2,2,2,
2,2,2,2,2,2,2,2,2,2,2,2,2,2,2,2,2,2,2,2,2,2,2,2,2,2,2,4),(-0.33219634213793,
-0.329780700017932,-0.326253263705674,-0.322343264986936,-0.315853218990654,
-0.289583593405523,-0.240675456116879,-0.216126043784944,-0.212163567942123,
-0.209677339654646,-0.207707026878352,-0.207685818623493,-0.207665034510622,
-0.207644659488958,-0.207624679188235,-0.207605079886582,-0.207585848468491,
-0.207566972395925,-0.207548439674398,-0.207530238828,-0.207512358866656,
-0.207494789267665,-0.207477519942781,-0.207460541221191,-0.207443843830181,
-0.207427418870173,-0.207411257791869,-0.207395352392427,-0.207379694790389,
-0.207364277408578,-0.207349092953033,-0.207334134421264,-0.207319395067114,
-0.207304868397298,-0.207290548154628,-0.207276428318404,-0.207262503074969,
-0.207248766830948,-0.207235214184885,-0.204785005062128,-0.199598524919195,
-0.192479352495597,-0.173996545250957,-0.113184680549314,-0.0991360032477435,
-0.0937136929300639,-0.0904001021820661,-0.0868217068297628,-0.0819424221188083,
-0.0704389941047528,-0.0285220420113346,-0.000702939858132017),
 .UNSPECIFIED.);
#970=B_SPLINE_CURVE_WITH_KNOTS('',3,(#69799,#69800,#69801,#69802,#69803,
#69804,#69805,#69806,#69807,#69808,#69809,#69810,#69811,#69812,#69813,#69814,
#69815,#69816,#69817,#69818,#69819,#69820,#69821,#69822,#69823,#69824,#69825,
#69826,#69827,#69828,#69829,#69830,#69831,#69832,#69833,#69834,#69835,#69836,
#69837,#69838,#69839,#69840,#69841,#69842,#69843,#69844,#69845,#69846,#69847,
#69848,#69849,#69850,#69851,#69852,#69853,#69854,#69855,#69856,#69857,#69858,
#69859,#69860,#69861,#69862,#69863,#69864,#69865,#69866,#69867,#69868,#69869,
#69870,#69871,#69872,#69873,#69874,#69875,#69876,#69877,#69878,#69879,#69880,
#69881,#69882,#69883,#69884,#69885,#69886,#69887,#69888,#69889,#69890,#69891,
#69892,#69893,#69894,#69895,#69896,#69897,#69898,#69899,#69900,#69901,#69902,
#69903,#69904,#69905,#69906,#69907,#69908,#69909,#69910,#69911,#69912,#69913,
#69914,#69915,#69916,#69917,#69918,#69919,#69920,#69921,#69922,#69923,#69924,
#69925,#69926,#69927,#69928,#69929,#69930,#69931,#69932,#69933,#69934,#69935,
#69936,#69937,#69938,#69939,#69940,#69941,#69942,#69943,#69944,#69945,#69946,
#69947,#69948,#69949,#69950,#69951,#69952,#69953,#69954,#69955,#69956,#69957,
#69958,#69959,#69960,#69961,#69962,#69963,#69964,#69965,#69966,#69967,#69968,
#69969,#69970,#69971,#69972),.UNSPECIFIED.,.F.,.F.,(4,2,2,2,2,2,2,2,2,2,
2,2,2,2,2,2,2,2,2,2,2,2,2,2,2,2,2,2,2,2,2,2,2,2,2,2,2,2,2,2,2,2,2,2,2,2,
2,2,2,2,2,2,2,2,2,2,2,2,2,2,2,2,2,2,2,2,2,2,2,2,2,2,2,2,2,2,2,2,2,2,2,2,
2,2,2,2,4),(-2.98923116400283,-2.97350991870706,-2.96578664491632,-2.9631530988098,
-2.96118316215222,-2.9592775365693,-2.95706493410813,-2.95328622285423,
-2.93922573353853,-2.92064083730378,-2.87219444671895,-2.85163865333969,
-2.84561657895374,-2.841808671401,-2.83825146479957,-2.8335812399366,-2.82300397488092,
-2.76465820540062,-2.75925053834816,-2.7392229460933,-2.73172790408425,
-2.72787624518902,-2.72465974888029,-2.72258397350011,-2.72056443361432,
-2.71806131387319,-2.7118411834863,-2.67548974943746,-2.64324945824292,
-2.61543268406738,-2.60884070663828,-2.60490889453594,-2.60138653790194,
-2.59689365497973,-2.58756866962727,-2.53349571784819,-2.52135871295193,
-2.5017323717477,-2.49073507268459,-2.48738676635101,-2.48526898138358,
-2.48324891131145,-2.48074406192153,-2.47451424885665,-2.4380334791975,
-2.40556070204055,-2.37807405548288,-2.37150300797432,-2.36757561032967,
-2.36405216580092,-2.35955094101059,-2.35018273025426,-2.29671933990866,
-2.2839249369236,-2.26437509173773,-2.25340581595576,-2.25006041290713,
-2.24794319687135,-2.2459225708695,-2.24341588188789,-2.2371757040023,-2.20085924559626,
-2.16863315120153,-2.14078883202881,-2.13419461343616,-2.13026205995826,
-2.12673941009988,-2.12224666344367,-2.1129238549481,-2.05880304139706,
-2.04670865598095,-2.0270758444224,-2.01607577759781,-2.01272695298232,
-2.01060891308836,-2.00858866296235,-2.00608365635305,-1.99985378414873,
-1.9633581611097,-1.92979684230373,-1.90327938960164,-1.89677237860318,
-1.89285864026042,-1.88933192404235,-1.88480493343468,-1.87530159794066,
-1.82652150981059),.UNSPECIFIED.);
#971=B_SPLINE_CURVE_WITH_KNOTS('',3,(#69977,#69978,#69979,#69980,#69981,
#69982,#69983,#69984,#69985,#69986,#69987,#69988,#69989,#69990,#69991,#69992,
#69993,#69994,#69995,#69996,#69997,#69998,#69999,#70000,#70001,#70002,#70003,
#70004,#70005,#70006,#70007,#70008,#70009,#70010,#70011,#70012,#70013,#70014,
#70015,#70016,#70017,#70018,#70019,#70020,#70021,#70022,#70023,#70024,#70025,
#70026,#70027,#70028,#70029,#70030,#70031,#70032,#70033,#70034,#70035,#70036,
#70037,#70038,#70039,#70040,#70041,#70042,#70043,#70044,#70045,#70046,#70047,
#70048,#70049,#70050,#70051,#70052,#70053,#70054,#70055,#70056,#70057,#70058,
#70059,#70060,#70061,#70062,#70063,#70064,#70065,#70066,#70067,#70068,#70069,
#70070,#70071,#70072,#70073,#70074,#70075,#70076,#70077,#70078,#70079,#70080,
#70081,#70082,#70083,#70084,#70085,#70086,#70087,#70088,#70089,#70090,#70091,
#70092,#70093,#70094,#70095,#70096,#70097,#70098,#70099,#70100,#70101,#70102,
#70103,#70104,#70105,#70106,#70107,#70108,#70109,#70110,#70111,#70112,#70113,
#70114,#70115,#70116,#70117,#70118,#70119,#70120,#70121,#70122,#70123,#70124,
#70125,#70126,#70127,#70128,#70129,#70130,#70131,#70132,#70133,#70134,#70135,
#70136,#70137,#70138,#70139,#70140,#70141,#70142,#70143,#70144,#70145,#70146,
#70147,#70148,#70149,#70150,#70151,#70152,#70153,#70154,#70155,#70156,#70157,
#70158,#70159,#70160,#70161,#70162,#70163,#70164,#70165,#70166,#70167,#70168,
#70169,#70170,#70171,#70172,#70173,#70174,#70175,#70176,#70177,#70178,#70179,
#70180,#70181,#70182,#70183,#70184,#70185,#70186,#70187,#70188),
 .UNSPECIFIED.,.F.,.F.,(4,2,2,2,2,2,2,2,2,2,2,2,2,2,2,2,2,2,2,2,2,2,2,2,
2,2,2,2,2,2,2,2,2,2,2,2,2,2,2,2,2,2,2,2,2,2,2,2,2,2,2,2,2,2,2,2,2,2,2,2,
2,2,2,2,2,2,2,2,2,2,2,2,2,2,2,2,2,2,2,2,2,2,2,2,2,2,2,2,2,2,2,2,2,2,2,2,
2,2,2,2,2,2,2,2,2,4),(-2.65803045946379,-2.64226021210847,-2.60283391067027,
-2.58329218308692,-2.57232559666882,-2.56898002275199,-2.56686245524302,
-2.56484124395464,-2.56233351631105,-2.55608914706894,-2.51983657207268,
-2.48770456775849,-2.45973838077491,-2.45313557848874,-2.44920059574953,
-2.44567742349223,-2.44118625988331,-2.43187494238457,-2.37760922753121,
-2.36566710851047,-2.34602694774608,-2.33502386378854,-2.33167425304181,
-2.32955572556937,-2.32753498003707,-2.32502927639262,-2.3187972248936,
-2.28234678185918,-2.24991529951816,-2.2223714872902,-2.21579537799238,
-2.21186605827334,-2.2083415585927,-2.20383988559011,-2.19447396592438,
-2.14096410474271,-2.12821561928296,-2.10866622379194,-2.09769641923997,
-2.09435027580758,-2.09223244070186,-2.09021105455898,-2.08770319432126,
-2.08145892018467,-2.04519237863354,-2.01304098640779,-1.98509444778547,
-1.97849238621133,-1.97455730643255,-1.97103371215114,-1.96654154998093,
-1.95722645550784,-1.90299233039496,-1.89101087342035,-1.87137241950139,
-1.86036957593958,-1.8570197677433,-1.85490105458919,-1.85288007929234,
-1.85037403564063,-1.84414086154228,-1.80812709664916,-1.77646543545933,
-1.74783435016955,-1.74118964342165,-1.73724517377457,-1.73372309304624,
-1.72924643422808,-1.7200134416298,-1.66476460763362,-1.65378875234948,
-1.63406228019062,-1.62302684766798,-1.61967342170932,-1.61755383339211,
-1.6155332456158,-1.61302896097876,-1.60680657728929,-1.57009141689533,
-1.53718816520174,-1.51936037772267,-1.50704009861802,-1.50202816598132,
-1.4984251755891,-1.49513853463789,-1.48987097426619,-1.47582800570569,
-1.45444190853355,-1.4041905518344,-1.38695828426794,-1.38297652127089,
-1.38069523149252,-1.37891235013502,-1.37640686913393,-1.37122724071527,
-1.3294021330354,-1.27783010482171,-1.26835652616225,-1.26383403716591,
-1.26030661010196,-1.25638774530475,-1.24986187247666,-1.22309546951146,
-1.18888163607689,-1.17856793304868,-1.16381432242618),.UNSPECIFIED.);
#972=B_SPLINE_CURVE_WITH_KNOTS('',3,(#70189,#70190,#70191,#70192,#70193,
#70194,#70195,#70196,#70197,#70198,#70199,#70200,#70201,#70202,#70203,#70204,
#70205,#70206,#70207,#70208,#70209,#70210,#70211,#70212,#70213,#70214,#70215,
#70216,#70217,#70218,#70219,#70220,#70221,#70222,#70223,#70224,#70225,#70226,
#70227,#70228,#70229,#70230,#70231,#70232,#70233,#70234,#70235,#70236,#70237,
#70238,#70239,#70240,#70241,#70242,#70243,#70244,#70245,#70246,#70247,#70248,
#70249,#70250,#70251,#70252,#70253,#70254,#70255,#70256,#70257,#70258,#70259,
#70260,#70261,#70262,#70263,#70264,#70265,#70266,#70267,#70268,#70269,#70270,
#70271,#70272,#70273,#70274,#70275,#70276,#70277,#70278,#70279,#70280,#70281,
#70282,#70283,#70284,#70285,#70286,#70287,#70288,#70289,#70290,#70291,#70292,
#70293,#70294,#70295,#70296,#70297,#70298,#70299,#70300,#70301,#70302,#70303,
#70304,#70305,#70306,#70307,#70308,#70309,#70310,#70311,#70312,#70313,#70314,
#70315,#70316,#70317,#70318,#70319,#70320,#70321,#70322,#70323,#70324,#70325,
#70326,#70327,#70328,#70329,#70330,#70331,#70332,#70333,#70334,#70335,#70336,
#70337,#70338,#70339,#70340,#70341,#70342,#70343,#70344,#70345,#70346,#70347,
#70348,#70349,#70350,#70351,#70352,#70353,#70354,#70355,#70356,#70357,#70358,
#70359,#70360,#70361,#70362,#70363,#70364,#70365,#70366,#70367,#70368,#70369,
#70370,#70371,#70372,#70373,#70374,#70375,#70376,#70377,#70378,#70379,#70380,
#70381,#70382,#70383,#70384,#70385,#70386,#70387,#70388,#70389,#70390,#70391,
#70392,#70393,#70394,#70395,#70396,#70397,#70398,#70399,#70400),
 .UNSPECIFIED.,.F.,.F.,(4,2,2,2,2,2,2,2,2,2,2,2,2,2,2,2,2,2,2,2,2,2,2,2,
2,2,2,2,2,2,2,2,2,2,2,2,2,2,2,2,2,2,2,2,2,2,2,2,2,2,2,2,2,2,2,2,2,2,2,2,
2,2,2,2,2,2,2,2,2,2,2,2,2,2,2,2,2,2,2,2,2,2,2,2,2,2,2,2,2,2,2,2,2,2,2,2,
2,2,2,2,2,2,2,2,2,4),(-1.82652150981059,-1.82436938606574,-1.79378793382466,
-1.78411596669254,-1.77744810307633,-1.77467634253647,-1.77267417723345,
-1.7704742614324,-1.76675459371402,-1.75336091165485,-1.6854537792428,-1.6717962571914,
-1.66170480454782,-1.65706968032381,-1.65352934909423,-1.6496705532801,
-1.6434152559009,-1.62264517566521,-1.57414675257705,-1.54325403633256,
-1.53885155126314,-1.53650419059199,-1.53453218780341,-1.53201263398553,
-1.52793840012921,-1.49537953414415,-1.44223245314841,-1.42672908473889,
-1.42109907187152,-1.41774675802364,-1.41419217730081,-1.40945954768364,
-1.39881962681617,-1.38417414468498,-1.33973219926227,-1.30610337622242,
-1.30202704769492,-1.29950689948934,-1.29753488080779,-1.29518801651949,
-1.2907878489589,-1.25998445097343,-1.21170428108578,-1.19072634557033,
-1.18444592019726,-1.1805816385128,-1.17704286144627,-1.17241931567192,
-1.16239202254442,-1.14884662567139,-1.08260439396749,-1.06757070578081,
-1.06370087915275,-1.06146790572012,-1.05947618839625,-1.05677415115838,
-1.05051957739217,-1.02066649511195,-0.967610382248828,-0.952041164521902,
-0.946377203075412,-0.943018172531551,-0.939466357131643,-0.934754296025357,
-0.924233766514298,-0.909805721577833,-0.86669207607966,-0.831351099773498,
-0.827262855721576,-0.82473900642763,-0.822766525063352,-0.820422001333221,
-0.816033770940867,-0.785799250185063,-0.738975316723177,-0.716270409628,
-0.709819769837866,-0.705918173118031,-0.702388533057668,-0.697838333695937,
-0.68821160420976,-0.675369237612917,-0.640628009802294,-0.596500135967312,
-0.590339045007555,-0.587919334539117,-0.585920620319059,-0.583764996257844,
-0.58024619689557,-0.567539328414932,-0.542914600957942,-0.482756059080605,
-0.474177651954468,-0.469772685899731,-0.466258644472913,-0.46227171211274,
-0.455427054685808,-0.423119707345982,-0.372679578173585,-0.355690131192574,
-0.351724357055762,-0.349447245693079,-0.347664550423079,-0.3451553943584,
-0.339953846388684,-0.332047463449011),.UNSPECIFIED.);
#973=B_SPLINE_CURVE_WITH_KNOTS('',3,(#70406,#70407,#70408,#70409,#70410,
#70411,#70412,#70413,#70414,#70415,#70416,#70417,#70418,#70419,#70420,#70421,
#70422,#70423,#70424,#70425,#70426,#70427,#70428,#70429,#70430,#70431,#70432,
#70433,#70434,#70435,#70436,#70437,#70438,#70439,#70440,#70441,#70442,#70443,
#70444,#70445,#70446,#70447,#70448,#70449,#70450,#70451,#70452,#70453,#70454,
#70455,#70456,#70457,#70458,#70459,#70460,#70461,#70462,#70463,#70464,#70465,
#70466,#70467,#70468,#70469,#70470,#70471,#70472,#70473,#70474,#70475,#70476,
#70477,#70478,#70479,#70480,#70481,#70482,#70483,#70484,#70485,#70486,#70487,
#70488,#70489,#70490,#70491,#70492,#70493,#70494,#70495,#70496,#70497,#70498,
#70499,#70500,#70501,#70502,#70503,#70504,#70505,#70506,#70507,#70508,#70509,
#70510,#70511,#70512,#70513,#70514,#70515,#70516,#70517,#70518,#70519,#70520,
#70521,#70522,#70523,#70524,#70525,#70526,#70527,#70528,#70529,#70530,#70531,
#70532,#70533,#70534,#70535,#70536,#70537,#70538,#70539,#70540,#70541,#70542,
#70543,#70544,#70545,#70546,#70547,#70548,#70549,#70550,#70551,#70552,#70553,
#70554,#70555,#70556,#70557,#70558,#70559,#70560,#70561,#70562,#70563,#70564,
#70565,#70566,#70567,#70568,#70569,#70570,#70571),.UNSPECIFIED.,.F.,.F.,
(4,2,2,2,2,2,2,2,2,2,2,2,2,2,2,2,2,2,2,2,2,2,2,2,2,2,2,2,2,2,2,2,2,2,2,
2,2,2,2,2,2,2,2,2,2,2,2,2,2,2,2,2,2,2,2,2,2,2,2,2,2,2,2,2,2,2,2,2,2,2,2,
2,2,2,2,2,2,2,2,2,2,2,4),(-1.16361468862912,-1.13591070982436,-1.12739573960449,
-1.12300314660491,-1.11948904505838,-1.11549133158903,-1.10860087101055,
-1.07536536616905,-1.03468119985899,-1.02350544422435,-1.00866901374354,
-1.00482211471208,-1.00259374415639,-1.00059988696707,-0.997886349066067,
-0.991567796525987,-0.961059762306479,-0.906062231532777,-0.892488769249181,
-0.887138685455116,-0.883837361075105,-0.880247274618603,-0.875306672853713,
-0.863434395695005,-0.798766725195472,-0.772267092181893,-0.768268255093271,
-0.765770573040939,-0.763798912615855,-0.761431740382097,-0.756938082041445,
-0.720301903177363,-0.661447563139146,-0.652707571750098,-0.648267981057946,
-0.644749529661597,-0.640782213240854,-0.634032665434681,-0.603593145875492,
-0.573360863187782,-0.561008217312841,-0.545252152865808,-0.533343227395491,
-0.529768495348602,-0.527600103862438,-0.525583740406508,-0.522731221088097,
-0.515564440822858,-0.504907929194273,-0.468289967457178,-0.425388760078435,
-0.415721958917442,-0.411212280110281,-0.407677194443301,-0.403791761436236,
-0.397419218251263,-0.372788821436176,-0.343797863991551,-0.300246372096205,
-0.294062694279302,-0.291638978528376,-0.289638846278831,-0.287484041524802,
-0.284346546321442,-0.273747708882288,-0.255105795635437,-0.196363923715957,
-0.180923789444152,-0.175301120334041,-0.171949275305025,-0.168392295787703,
-0.163651470457424,-0.153740463298352,-0.122274699879399,-0.0929452027344989,
-0.0603217159816636,-0.0562457572621282,-0.0537252348857149,-0.0517525044125253,
-0.0494042292088944,-0.046882861007685,-0.0428648294254301,-0.000702153330958493),
 .UNSPECIFIED.);
#974=B_SPLINE_CURVE_WITH_KNOTS('',3,(#70572,#70573,#70574,#70575,#70576,
#70577,#70578,#70579,#70580,#70581,#70582,#70583,#70584,#70585,#70586,#70587,
#70588,#70589,#70590,#70591,#70592,#70593,#70594,#70595,#70596,#70597,#70598,
#70599,#70600,#70601,#70602,#70603,#70604,#70605,#70606,#70607,#70608,#70609,
#70610,#70611,#70612,#70613,#70614,#70615,#70616,#70617,#70618,#70619,#70620,
#70621,#70622,#70623),.UNSPECIFIED.,.F.,.F.,(4,2,2,2,2,2,2,2,2,2,2,2,2,
2,2,2,2,2,2,2,2,2,2,2,2,4),(-2.9894592038886,-2.94072867183443,-2.93345639399262,
-2.92890227577676,-2.92463163473601,-2.92112602038026,-2.91703802497621,
-2.90992050663652,-2.8742516809235,-2.84276493212935,-2.81243649597813,
-2.80759053660584,-2.80558680107853,-2.80358191501645,-2.80138808309417,
-2.79769690939084,-2.78462552240191,-2.73789202785937,-2.71125105675867,
-2.70031357867313,-2.69181076867664,-2.68747734045533,-2.68396834782805,
-2.67993006001617,-2.6730328140185,-2.65803045946379),.UNSPECIFIED.);
#975=B_SPLINE_CURVE_WITH_KNOTS('',3,(#70625,#70626,#70627,#70628,#70629,
#70630,#70631,#70632,#70633,#70634,#70635,#70636,#70637,#70638,#70639,#70640,
#70641,#70642,#70643,#70644,#70645,#70646,#70647,#70648,#70649,#70650,#70651,
#70652,#70653,#70654,#70655,#70656,#70657,#70658,#70659,#70660,#70661,#70662,
#70663,#70664,#70665,#70666,#70667,#70668,#70669,#70670,#70671,#70672,#70673,
#70674,#70675,#70676,#70677,#70678,#70679,#70680,#70681,#70682,#70683,#70684,
#70685,#70686,#70687,#70688,#70689,#70690),.UNSPECIFIED.,.F.,.F.,(4,2,2,
2,2,2,2,2,2,2,2,2,2,2,2,2,2,2,2,2,2,2,2,2,2,2,2,2,2,2,2,2,4),(-0.332047463449011,
-0.303400555046417,-0.245829991390745,-0.237026875411861,-0.232534989753045,
-0.229098968084146,-0.228612501900887,-0.228394127212428,-0.228237036682089,
-0.228118050538032,-0.228024810459153,-0.227949958397452,-0.227888773545902,
-0.227731450566128,-0.227578535673357,-0.227428881830288,-0.22728149732593,
-0.227135505124343,-0.226990112389834,-0.226844587029383,-0.222200697807029,
-0.21079088074934,-0.171354894123508,-0.12100868122166,-0.115305898626846,
-0.112729868070505,-0.11074861658915,-0.10847020567436,-0.10439159902682,
-0.0833266707054811,-0.0240188320508272,-0.00836037945646354,-0.000702471133105883),
 .UNSPECIFIED.);
#976=B_SPLINE_CURVE_WITH_KNOTS('',3,(#70691,#70692,#70693,#70694,#70695,
#70696,#70697,#70698,#70699,#70700,#70701,#70702,#70703,#70704,#70705,#70706,
#70707,#70708,#70709,#70710,#70711,#70712,#70713,#70714,#70715,#70716,#70717,
#70718,#70719,#70720,#70721,#70722,#70723,#70724,#70725,#70726,#70727,#70728,
#70729,#70730,#70731,#70732,#70733,#70734,#70735,#70736,#70737,#70738,#70739,
#70740,#70741,#70742,#70743,#70744,#70745,#70746,#70747,#70748,#70749,#70750,
#70751,#70752,#70753,#70754,#70755,#70756,#70757,#70758,#70759,#70760,#70761,
#70762,#70763,#70764,#70765,#70766,#70767,#70768,#70769,#70770,#70771,#70772,
#70773,#70774,#70775,#70776,#70777,#70778,#70779,#70780,#70781,#70782,#70783,
#70784,#70785,#70786,#70787,#70788,#70789,#70790,#70791,#70792,#70793,#70794,
#70795,#70796,#70797,#70798,#70799,#70800,#70801,#70802,#70803,#70804,#70805,
#70806,#70807,#70808,#70809,#70810,#70811,#70812,#70813,#70814,#70815,#70816,
#70817,#70818,#70819,#70820,#70821,#70822,#70823,#70824,#70825,#70826,#70827,
#70828,#70829,#70830,#70831,#70832,#70833,#70834,#70835,#70836,#70837,#70838,
#70839,#70840,#70841,#70842,#70843,#70844,#70845,#70846,#70847,#70848,#70849,
#70850,#70851,#70852,#70853,#70854,#70855,#70856,#70857,#70858),
 .UNSPECIFIED.,.F.,.F.,(4,2,2,2,2,2,2,2,2,2,2,2,2,2,2,2,2,2,2,2,2,2,2,2,
2,2,2,2,2,2,2,2,2,2,2,2,2,2,2,2,2,2,2,2,2,2,2,2,2,2,2,2,2,2,2,2,2,2,2,2,
2,2,2,2,2,2,2,2,2,2,2,2,2,2,2,2,2,2,2,2,2,2,2,4),(-2.9888980801213,-2.98659890828846,
-2.98372924307055,-2.98037750013604,-2.97660887900156,-2.97098364046133,
-2.95463264440861,-2.93999827913173,-2.87627846302085,-2.86732908628589,
-2.86422334486029,-2.86215838745305,-2.86031599248123,-2.85730409716806,
-2.84965403019633,-2.80168606304042,-2.75794759340087,-2.75217033001485,
-2.74822915514659,-2.74445506241092,-2.74108388046826,-2.73654800310842,
-2.72753178281579,-2.67215361141063,-2.66093115514727,-2.64146094801411,
-2.63052210656701,-2.62718055804286,-2.6250645565352,-2.62304402637343,
-2.62053634261057,-2.61428806839151,-2.57811540436078,-2.5461094894657,
-2.51797645940766,-2.51136535820683,-2.50742980576017,-2.5039088629799,
-2.49942432461223,-2.49014086192319,-2.43555592122954,-2.42395092719871,
-2.40427759126799,-2.39326360791122,-2.38991386471929,-2.38779598840643,
-2.38577653862038,-2.38327319847313,-2.37705085480809,-2.34043052757807,
-2.30764415044508,-2.28056641255628,-2.27402292584378,-2.27010192077385,
-2.26657788533634,-2.26206714805437,-2.25264629305985,-2.20008228493633,
-2.15810035807378,-2.15357312426116,-2.15119987183147,-2.14922991060268,
-2.1467430050574,-2.14277743326965,-2.11831344385612,-2.10442749337622,
-2.07456474064297,-2.04368768256641,-2.03691734316567,-2.03294690440117,
-2.02943121059756,-2.02500253803345,-2.01630830097722,-1.9570621397245,
-1.94972305472276,-1.92977916688445,-1.9186654438361,-1.9153046936313,-1.91318416371864,
-1.91116589580897,-1.90866789846227,-1.90247818996896,-1.86296053730906,
-1.82609948607109),.UNSPECIFIED.);
#977=B_SPLINE_CURVE_WITH_KNOTS('',3,(#70863,#70864,#70865,#70866,#70867,
#70868,#70869,#70870,#70871,#70872,#70873,#70874,#70875,#70876,#70877,#70878,
#70879,#70880,#70881,#70882,#70883,#70884,#70885,#70886,#70887,#70888,#70889,
#70890,#70891,#70892,#70893,#70894,#70895,#70896,#70897,#70898,#70899,#70900,
#70901,#70902,#70903,#70904,#70905,#70906,#70907,#70908,#70909,#70910,#70911,
#70912,#70913,#70914,#70915,#70916,#70917,#70918,#70919,#70920,#70921,#70922,
#70923,#70924,#70925,#70926,#70927,#70928,#70929,#70930,#70931,#70932,#70933,
#70934,#70935,#70936,#70937,#70938,#70939,#70940,#70941,#70942,#70943,#70944,
#70945,#70946,#70947,#70948,#70949,#70950,#70951,#70952,#70953,#70954,#70955,
#70956,#70957,#70958,#70959,#70960,#70961,#70962,#70963,#70964,#70965,#70966,
#70967,#70968,#70969,#70970,#70971,#70972,#70973,#70974,#70975,#70976,#70977,
#70978,#70979,#70980,#70981,#70982,#70983,#70984,#70985,#70986,#70987,#70988,
#70989,#70990,#70991,#70992,#70993,#70994,#70995,#70996,#70997,#70998,#70999,
#71000,#71001,#71002,#71003,#71004,#71005,#71006,#71007,#71008,#71009,#71010,
#71011,#71012,#71013,#71014,#71015,#71016,#71017,#71018,#71019,#71020,#71021,
#71022,#71023,#71024,#71025,#71026,#71027,#71028,#71029,#71030,#71031,#71032,
#71033,#71034,#71035,#71036,#71037,#71038,#71039,#71040,#71041,#71042,#71043,
#71044,#71045,#71046,#71047,#71048,#71049,#71050,#71051,#71052,#71053,#71054,
#71055,#71056,#71057,#71058,#71059,#71060,#71061,#71062,#71063,#71064,#71065,
#71066,#71067,#71068,#71069,#71070),.UNSPECIFIED.,.F.,.F.,(4,2,2,2,2,2,
2,2,2,2,2,2,2,2,2,2,2,2,2,2,2,2,2,2,2,2,2,2,2,2,2,2,2,2,2,2,2,2,2,2,2,2,
2,2,2,2,2,2,2,2,2,2,2,2,2,2,2,2,2,2,2,2,2,2,2,2,2,2,2,2,2,2,2,2,2,2,2,2,
2,2,2,2,2,2,2,2,2,2,2,2,2,2,2,2,2,2,2,2,2,2,2,2,2,4),(-2.65786654937229,
-2.6529365402186,-2.61648033408661,-2.58403955006769,-2.55651262958186,
-2.54993782767042,-2.54600890460589,-2.54248452032328,-2.53798266299572,
-2.52861512193393,-2.4751384225726,-2.46235606426173,-2.44281234145399,
-2.43184480118368,-2.42849899929746,-2.4263813016966,-2.42435997855497,
-2.42185212503233,-2.4156075073799,-2.37935127603316,-2.34721496018183,
-2.31925058930345,-2.31264762143709,-2.30871245797945,-2.30518907286372,
-2.30069756776036,-2.29138528235673,-2.23712207514439,-2.22517348335998,
-2.20553274923148,-2.19452923598394,-2.19117945369731,-2.18906080855365,
-2.18703994283401,-2.18453408184178,-2.17830159719707,-2.14235895482372,
-2.11131316535685,-2.08206778362889,-2.07538664539881,-2.07143438562164,
-2.0679138608872,-2.06345075891303,-2.05428791893292,-1.99828144909136,
-1.98803054787728,-1.9682527331741,-1.96081640825548,-1.95535267996113,
-1.95279299150279,-1.95081731400885,-1.94849803922697,-1.94434778233372,
-1.92418216658248,-1.88578275523273,-1.84776166172448,-1.83932250656845,
-1.83500139510386,-1.83149266527866,-1.82744389699321,-1.82050206511842,
-1.78885264813844,-1.73924807985244,-1.72095566464168,-1.71702281726244,
-1.71477564877904,-1.71278686377196,-1.71015607233604,-1.70414857158634,
-1.65734930566419,-1.61503979350774,-1.60351415763342,-1.59863004531015,
-1.59504969827237,-1.59173538834381,-1.58631440511016,-1.5722833382831,
-1.51769942985883,-1.49482590101837,-1.48290401292882,-1.47932779798563,
-1.4771590216465,-1.47514271396149,-1.47229086315159,-1.46512881286195,
-1.4544819843237,-1.41793014562285,-1.37494295816848,-1.36527540143453,
-1.36076547077831,-1.35723023007053,-1.35334467007749,-1.34697201871411,
-1.32234264779079,-1.293355042916,-1.24980343393933,-1.24361357104473,-1.24118882418992,
-1.23918838409349,-1.23703393780808,-1.23352270748998,-1.22090615996886,
-1.1965683325924,-1.16361468862912),.UNSPECIFIED.);
#978=B_SPLINE_CURVE_WITH_KNOTS('',3,(#71071,#71072,#71073,#71074,#71075,
#71076,#71077,#71078,#71079,#71080,#71081,#71082,#71083,#71084,#71085,#71086,
#71087,#71088,#71089,#71090,#71091,#71092,#71093,#71094,#71095,#71096,#71097,
#71098,#71099,#71100,#71101,#71102,#71103,#71104,#71105,#71106,#71107,#71108,
#71109,#71110,#71111,#71112,#71113,#71114,#71115,#71116,#71117,#71118,#71119,
#71120,#71121,#71122,#71123,#71124,#71125,#71126,#71127,#71128,#71129,#71130,
#71131,#71132,#71133,#71134,#71135,#71136,#71137,#71138,#71139,#71140,#71141,
#71142,#71143,#71144,#71145,#71146,#71147,#71148,#71149,#71150,#71151,#71152,
#71153,#71154,#71155,#71156,#71157,#71158,#71159,#71160,#71161,#71162,#71163,
#71164,#71165,#71166,#71167,#71168,#71169,#71170,#71171,#71172,#71173,#71174,
#71175,#71176,#71177,#71178,#71179,#71180,#71181,#71182,#71183,#71184,#71185,
#71186,#71187,#71188,#71189,#71190,#71191,#71192,#71193,#71194,#71195,#71196,
#71197,#71198,#71199,#71200,#71201,#71202,#71203,#71204,#71205,#71206,#71207,
#71208,#71209,#71210,#71211,#71212,#71213,#71214,#71215,#71216,#71217,#71218,
#71219,#71220,#71221,#71222,#71223,#71224,#71225,#71226,#71227,#71228,#71229,
#71230,#71231,#71232,#71233,#71234,#71235,#71236,#71237,#71238,#71239,#71240,
#71241,#71242,#71243,#71244,#71245,#71246,#71247,#71248,#71249,#71250,#71251,
#71252,#71253,#71254,#71255,#71256,#71257,#71258,#71259,#71260,#71261,#71262,
#71263,#71264,#71265,#71266,#71267,#71268,#71269,#71270,#71271,#71272,#71273,
#71274,#71275,#71276,#71277,#71278,#71279,#71280,#71281,#71282,#71283,#71284,
#71285,#71286,#71287,#71288),.UNSPECIFIED.,.F.,.F.,(4,2,2,2,2,2,2,2,2,2,
2,2,2,2,2,2,2,2,2,2,2,2,2,2,2,2,2,2,2,2,2,2,2,2,2,2,2,2,2,2,2,2,2,2,2,2,
2,2,2,2,2,2,2,2,2,2,2,2,2,2,2,2,2,2,2,2,2,2,2,2,2,2,2,2,2,2,2,2,2,2,2,2,
2,2,2,2,2,2,2,2,2,2,2,2,2,2,2,2,2,2,2,2,2,2,2,2,2,2,4),(-1.82609948607109,
-1.82510996968395,-1.8116369689304,-1.80164973155598,-1.79703353778286,
-1.79349581271202,-1.78962815753855,-1.78333200611036,-1.76219866393818,
-1.7140161799052,-1.69294958838722,-1.68143315410374,-1.67803032566534,
-1.67590048245194,-1.67388798876404,-1.67094403250579,-1.66534467890069,
-1.62222450569465,-1.59300891821837,-1.56828106523965,-1.56190305076054,
-1.55801749114935,-1.55448437958399,-1.54998009637972,-1.54033656019384,
-1.49461990550496,-1.44845381150723,-1.44241901832225,-1.43978402625333,
-1.43779528270211,-1.43555188588275,-1.43163397910172,-1.41357468074426,
-1.37798327886645,-1.33259618679356,-1.32539282445486,-1.32128607478548,
-1.31781563837782,-1.31358380528806,-1.30557998214565,-1.29545545103272,
-1.27183423872731,-1.22155547238159,-1.20746257574622,-1.20368033329347,
-1.20146663653604,-1.19946919969576,-1.19672785001681,-1.1902424005164,
-1.18092324402375,-1.15227631392267,-1.09861442112409,-1.08926182411377,
-1.08476328800386,-1.08123983097987,-1.07731023210765,-1.07073026296823,
-1.04311677833627,-1.01069584273963,-0.974246084158036,-0.968010150439186,
-0.965504070479153,-0.963483517706516,-0.96136582288322,-0.958018733058799,
-0.947034812539828,-0.927448293919822,-0.915110099560047,-0.861243594017119,
-0.851905765605036,-0.847410120955484,-0.843887085393732,-0.839956051223714,
-0.833369093855505,-0.805644171055192,-0.773302555622228,-0.736906549956271,
-0.730667552316209,-0.728160997387964,-0.72614036307873,-0.724022957030094,
-0.720676974657335,-0.709702693275992,-0.690141965159893,-0.677593818717236,
-0.623924831487843,-0.614573571971335,-0.610075466793283,-0.606552254456802,
-0.602622832584194,-0.596042929282728,-0.568425609018339,-0.53601068474551,
-0.499565947704492,-0.493330261506392,-0.490824317619946,-0.488803889150593,
-0.486686342727361,-0.483339518987976,-0.472356762702184,-0.452772737415233,
-0.440424670819912,-0.38657171767054,-0.377233780102893,-0.372738291825032,
-0.36921547025124,-0.365284769398792,-0.358698598155218,-0.331874846602485),
 .UNSPECIFIED.);
#979=B_SPLINE_CURVE_WITH_KNOTS('',3,(#71294,#71295,#71296,#71297,#71298,
#71299,#71300,#71301,#71302),.UNSPECIFIED.,.F.,.F.,(4,1,1,1,1,1,4),(78.5398163397448,
79.1666675558176,80.1646843164291,81.1627010770406,82.1607178376521,83.1587345982636,
83.4308627901788),.UNSPECIFIED.);
#980=B_SPLINE_CURVE_WITH_KNOTS('',3,(#71303,#71304,#71305,#71306,#71307,
#71308,#71309,#71310,#71311,#71312,#71313,#71314,#71315,#71316,#71317,#71318,
#71319,#71320,#71321,#71322,#71323,#71324,#71325,#71326,#71327,#71328,#71329,
#71330,#71331,#71332,#71333,#71334,#71335,#71336,#71337,#71338,#71339,#71340,
#71341,#71342,#71343,#71344,#71345,#71346,#71347,#71348,#71349,#71350,#71351,
#71352),.UNSPECIFIED.,.F.,.F.,(4,2,2,2,2,2,2,2,2,2,2,2,2,2,2,2,2,2,2,2,
2,2,2,2,4),(-2.9889941003972,-2.94117567294498,-2.90849158293237,-2.90405444645073,
-2.9016996637602,-2.89972800366745,-2.897217195552,-2.89317276033964,-2.85752537112561,
-2.81606404242647,-2.80089711019658,-2.79338168698881,-2.78714903056937,
-2.78337719866878,-2.77985470062432,-2.77536634470668,-2.76606805850765,
-2.69980828847285,-2.68016585517106,-2.66916210449532,-2.66581251999726,
-2.66369406061272,-2.66167342460859,-2.65916790343206,-2.65786654937229),
 .UNSPECIFIED.);
#981=B_SPLINE_CURVE_WITH_KNOTS('',3,(#71354,#71355,#71356,#71357,#71358,
#71359,#71360,#71361,#71362,#71363,#71364,#71365,#71366,#71367,#71368,#71369,
#71370,#71371,#71372,#71373,#71374,#71375,#71376,#71377,#71378,#71379,#71380,
#71381,#71382,#71383,#71384,#71385,#71386,#71387,#71388,#71389,#71390,#71391,
#71392,#71393,#71394,#71395,#71396,#71397,#71398,#71399,#71400,#71401,#71402,
#71403,#71404,#71405,#71406,#71407,#71408,#71409),.UNSPECIFIED.,.F.,.F.,
(4,2,2,2,2,2,2,2,2,2,2,2,2,2,2,2,2,2,2,2,2,2,2,2,2,2,2,4),(-0.331874846602485,
-0.330981074388004,-0.2986376438995,-0.262216318443132,-0.255994998427963,
-0.25349155534447,-0.25147183558706,-0.249395938112561,-0.246159052427811,
-0.242292995033285,-0.234758194038605,-0.214564724868786,-0.16816964018585,
-0.144500175505225,-0.137975786707741,-0.134058544165221,-0.130533052275814,
-0.126013730315575,-0.116549587179866,-0.0785297517278548,-0.0345880112104803,
-0.0207453104793424,-0.016979886525497,-0.0147700193402066,-0.0128658034662866,
-0.0108942416976137,-0.00825649642932359,-0.000701672936245559),
 .UNSPECIFIED.);
#982=B_SPLINE_CURVE_WITH_KNOTS('',3,(#71410,#71411,#71412,#71413,#71414,
#71415,#71416,#71417,#71418,#71419,#71420,#71421,#71422,#71423,#71424,#71425,
#71426,#71427,#71428,#71429,#71430,#71431,#71432,#71433,#71434,#71435,#71436,
#71437,#71438,#71439,#71440,#71441,#71442,#71443,#71444,#71445,#71446,#71447,
#71448,#71449,#71450,#71451,#71452,#71453,#71454,#71455,#71456,#71457,#71458,
#71459,#71460,#71461,#71462,#71463,#71464,#71465,#71466,#71467,#71468,#71469,
#71470,#71471,#71472,#71473,#71474,#71475,#71476,#71477,#71478,#71479,#71480,
#71481,#71482,#71483,#71484,#71485,#71486,#71487,#71488,#71489,#71490,#71491,
#71492,#71493,#71494,#71495,#71496,#71497,#71498,#71499,#71500,#71501,#71502,
#71503,#71504,#71505,#71506,#71507,#71508,#71509,#71510,#71511,#71512,#71513,
#71514,#71515,#71516,#71517,#71518,#71519,#71520,#71521,#71522,#71523,#71524,
#71525,#71526,#71527,#71528,#71529,#71530,#71531,#71532,#71533,#71534,#71535,
#71536,#71537,#71538,#71539,#71540,#71541,#71542,#71543,#71544,#71545,#71546,
#71547,#71548,#71549,#71550,#71551,#71552,#71553,#71554,#71555,#71556,#71557,
#71558,#71559,#71560,#71561),.UNSPECIFIED.,.F.,.F.,(4,2,2,2,2,2,2,2,2,2,
2,2,2,2,2,2,2,2,2,2,2,2,2,2,2,2,2,2,2,2,2,2,2,2,2,2,2,2,2,2,2,2,2,2,2,2,
2,2,2,2,2,2,2,2,2,2,2,2,2,2,2,2,2,2,2,2,2,2,2,2,2,2,2,2,2,4),(-2.98947308457363,
-2.92733685589138,-2.89638058913975,-2.88960703955114,-2.88563639496454,
-2.88212153340197,-2.87769526821824,-2.8687142454158,-2.81101057210273,
-2.80104428855757,-2.78206038303968,-2.77481822994585,-2.77105751261116,
-2.76795891131662,-2.76589335283727,-2.76387418787005,-2.76137174871138,
-2.75515439156189,-2.71826833183109,-2.68498659539138,-2.65857976050418,
-2.65208173438772,-2.64817069337677,-2.64464469487812,-2.64011623552978,
-2.63060072423233,-2.58004290238287,-2.5374652052823,-2.5321516480703,-2.52962134718892,
-2.52764897186441,-2.52531067471624,-2.52107212068079,-2.49923698824174,
-2.45347336078277,-2.42185104324977,-2.4150423053918,-2.41106378256141,
-2.40754962611141,-2.40313449767996,-2.39450422966814,-2.33474836239405,
-2.30987416940064,-2.29709048226513,-2.29356514861299,-2.2914084367786,
-2.28941103148284,-2.28699531262287,-2.28085713125145,-2.23639916619518,
-2.20192705028659,-2.18914336216528,-2.17955005796697,-2.17500672324226,
-2.17147858558358,-2.16757476978702,-2.16111136876808,-2.1385051038632,
-2.09148709769598,-2.07087062992221,-2.0595142620841,-2.05612812272256,
-2.05400206684067,-2.05198749883866,-2.0495034068519,-2.04339396961612,
-2.00130874120363,-1.95382361140584,-1.94287953002613,-1.93809460359827,
-1.93453209220951,-1.93073634304694,-1.92477136632288,-1.9066149657525,
-1.85584575360824,-1.82652085594837),.UNSPECIFIED.);
#983=B_SPLINE_CURVE_WITH_KNOTS('',3,(#71567,#71568,#71569,#71570,#71571,
#71572,#71573,#71574,#71575,#71576,#71577,#71578,#71579,#71580,#71581,#71582,
#71583,#71584,#71585,#71586,#71587,#71588,#71589,#71590,#71591,#71592,#71593,
#71594,#71595,#71596,#71597,#71598,#71599,#71600,#71601,#71602,#71603,#71604,
#71605,#71606,#71607,#71608,#71609,#71610,#71611,#71612,#71613,#71614,#71615,
#71616,#71617,#71618,#71619,#71620,#71621,#71622,#71623,#71624,#71625,#71626,
#71627,#71628,#71629,#71630,#71631,#71632,#71633,#71634,#71635,#71636,#71637,
#71638,#71639,#71640,#71641,#71642,#71643,#71644,#71645,#71646,#71647,#71648,
#71649,#71650,#71651,#71652,#71653,#71654,#71655,#71656,#71657),
 .UNSPECIFIED.,.F.,.F.,(4,3,3,3,3,3,3,3,3,3,3,3,3,3,3,3,3,3,3,3,3,3,3,3,
3,3,3,3,3,3,4),(84.8230016469244,85.0319268137513,85.1547681194866,85.3334304922201,
85.5117309654079,85.6900028877257,85.8682449824607,86.0469043800704,86.1527848800981,
86.3314472528316,86.5097477260194,86.6880196483371,86.8662617430722,87.0449211406819,
87.1508016407096,87.3294640134431,87.5077644866309,87.6860364089486,87.8642785036837,
88.0429379012934,88.1488184013211,88.3274807740546,88.5057812472424,88.6840531695601,
88.8622952642952,89.0409546619049,89.1468351619326,89.3254945334179,89.503793727625,
89.6819399833619,89.7129494036681),.UNSPECIFIED.);
#984=B_SPLINE_CURVE_WITH_KNOTS('',3,(#71658,#71659,#71660,#71661,#71662),
 .UNSPECIFIED.,.F.,.F.,(4,1,4),(83.4308627901788,84.1567513588751,84.8230016469244),
 .UNSPECIFIED.);
#985=B_SPLINE_CURVE_WITH_KNOTS('',3,(#71663,#71664,#71665,#71666,#71667,
#71668,#71669,#71670,#71671,#71672,#71673,#71674,#71675,#71676,#71677,#71678,
#71679,#71680,#71681,#71682,#71683,#71684,#71685,#71686,#71687,#71688,#71689,
#71690,#71691,#71692,#71693,#71694,#71695,#71696,#71697,#71698,#71699,#71700,
#71701,#71702,#71703,#71704,#71705,#71706,#71707,#71708,#71709,#71710,#71711,
#71712,#71713,#71714,#71715,#71716,#71717,#71718,#71719,#71720,#71721,#71722,
#71723,#71724,#71725,#71726,#71727,#71728,#71729,#71730,#71731,#71732,#71733,
#71734,#71735,#71736,#71737,#71738,#71739,#71740,#71741,#71742,#71743,#71744,
#71745,#71746,#71747,#71748,#71749,#71750,#71751,#71752,#71753,#71754,#71755,
#71756,#71757,#71758,#71759,#71760,#71761,#71762,#71763,#71764,#71765,#71766,
#71767,#71768,#71769,#71770,#71771,#71772,#71773,#71774,#71775,#71776,#71777,
#71778,#71779,#71780,#71781,#71782,#71783,#71784,#71785,#71786,#71787,#71788,
#71789,#71790,#71791,#71792,#71793,#71794,#71795,#71796,#71797,#71798,#71799,
#71800,#71801,#71802,#71803,#71804,#71805,#71806,#71807,#71808,#71809,#71810,
#71811,#71812,#71813,#71814,#71815,#71816,#71817,#71818,#71819,#71820,#71821,
#71822,#71823,#71824,#71825,#71826,#71827,#71828,#71829,#71830,#71831,#71832,
#71833,#71834,#71835,#71836,#71837,#71838,#71839,#71840,#71841,#71842,#71843,
#71844,#71845,#71846,#71847,#71848,#71849,#71850,#71851,#71852,#71853,#71854,
#71855,#71856,#71857,#71858,#71859,#71860,#71861,#71862,#71863,#71864,#71865,
#71866,#71867,#71868,#71869,#71870,#71871,#71872,#71873,#71874,#71875,#71876,
#71877,#71878,#71879,#71880,#71881,#71882),.UNSPECIFIED.,.F.,.F.,(4,2,2,
2,2,2,2,2,2,2,2,2,2,2,2,2,2,2,2,2,2,2,2,2,2,2,2,2,2,2,2,2,2,2,2,2,2,2,2,
2,2,2,2,2,2,2,2,2,2,2,2,2,2,2,2,2,2,2,2,2,2,2,2,2,2,2,2,2,2,2,2,2,2,2,2,
2,2,2,2,2,2,2,2,2,2,2,2,2,2,2,2,2,2,2,2,2,2,2,2,2,2,2,2,2,2,2,2,2,2,4),
(-1.82652085594837,-1.82406204444472,-1.81964186274556,-1.81729087685041,
-1.81531930969633,-1.81280475315443,-1.80874701554698,-1.77878274140315,
-1.73297326394166,-1.70894901209819,-1.70262555105294,-1.69875202399187,
-1.69521604551064,-1.69068911637525,-1.68092074746702,-1.60672232488165,
-1.59279128133492,-1.5868869867704,-1.58231744638724,-1.57993505369438,
-1.57796500509951,-1.57548742120362,-1.571553959497,-1.54794573103635,-1.4953087126614,
-1.47184901451365,-1.46533974043969,-1.46142544076611,-1.45789872425181,
-1.4533724379117,-1.44387325730934,-1.43125181109302,-1.39753912636128,
-1.35181593332644,-1.34575844792861,-1.34311940214136,-1.34112999066883,
-1.33888859263984,-1.33498021751713,-1.31708208510641,-1.28134865949066,
-1.23591896765176,-1.22871491816466,-1.22460786486309,-1.22113722230895,
-1.21690519975155,-1.20890121066523,-1.19877657949399,-1.17515577025408,
-1.12485043332524,-1.11077443273345,-1.10699352183774,-1.10478003475333,
-1.1027823655374,-1.10004011595922,-1.09354991088976,-1.08422183417085,
-1.0555284691054,-1.00192981325635,-0.992572104563909,-0.988072434573773,
-0.9845486682627,-0.980619322144993,-0.97404121268974,-0.946461112941453,
-0.91401398756701,-0.877545494795288,-0.871310154955984,-0.868804089109916,
-0.866783458173022,-0.864665570228491,-0.861317981638216,-0.850330637741892,
-0.830735452233746,-0.818463111266026,-0.764530415381216,-0.75519654034019,
-0.750701482242022,-0.747178329724924,-0.743246568718614,-0.736656957371985,
-0.708895016571605,-0.676576249384858,-0.640194461918078,-0.633954014283076,
-0.631447125315986,-0.629426320719903,-0.62730885913475,-0.623963002758799,
-0.612991104872757,-0.593437445668221,-0.580824086013084,-0.527210797961385,
-0.517854932158082,-0.513355788937934,-0.509832278127396,-0.505903054778885,
-0.499324761201724,-0.471736955864815,-0.439298500178054,-0.402836868352165,
-0.39660167345509,-0.394095726216383,-0.392075214979328,-0.389957482383299,
-0.386610191357697,-0.375624304361944,-0.356032405917324,-0.352157376078528,
-0.332127671321822),.UNSPECIFIED.);
#986=B_SPLINE_CURVE_WITH_KNOTS('',3,(#71888,#71889,#71890,#71891,#71892,
#71893,#71894,#71895,#71896),.UNSPECIFIED.,.F.,.F.,(4,1,1,1,1,1,4),(91.1061869541039,
91.1428686831556,92.1408854437671,93.1389022043786,94.1369189649901,95.1349357256016,
95.9956065629),.UNSPECIFIED.);
#987=B_SPLINE_CURVE_WITH_KNOTS('',3,(#71897,#71898,#71899,#71900,#71901,
#71902,#71903,#71904,#71905,#71906,#71907,#71908,#71909,#71910,#71911,#71912,
#71913,#71914,#71915,#71916,#71917,#71918,#71919,#71920,#71921,#71922,#71923,
#71924),.UNSPECIFIED.,.F.,.F.,(4,3,3,3,3,3,3,3,3,4),(89.7129494036681,89.8912023488036,
90.0698639783069,90.1448519225441,90.3224643810971,90.4997174006465,90.6769397930551,
90.8541428000862,91.031738874977,91.1061866323843),.UNSPECIFIED.);
#988=B_SPLINE_CURVE_WITH_KNOTS('',3,(#71926,#71927,#71928,#71929,#71930,
#71931,#71932,#71933,#71934,#71935,#71936,#71937,#71938,#71939,#71940,#71941,
#71942,#71943,#71944,#71945,#71946,#71947,#71948,#71949,#71950,#71951,#71952,
#71953,#71954,#71955,#71956,#71957,#71958,#71959,#71960,#71961,#71962,#71963,
#71964,#71965,#71966,#71967,#71968,#71969,#71970,#71971,#71972,#71973,#71974,
#71975,#71976,#71977,#71978,#71979,#71980,#71981),.UNSPECIFIED.,.F.,.F.,
(4,2,2,2,2,2,2,2,2,2,2,2,2,2,2,2,2,2,2,2,2,2,2,2,2,2,2,4),(-0.332127671321822,
-0.299591807458999,-0.283455651450869,-0.277740657579193,-0.273998034540904,
-0.270479790062397,-0.265706351666199,-0.260339045591067,-0.251038651666556,
-0.230274082707922,-0.187317120202878,-0.16247760069458,-0.158495652787689,
-0.156003629954979,-0.154033118948062,-0.151663403654923,-0.147154364224762,
-0.10867916126003,-0.0800334345805236,-0.0554583953642009,-0.0443802412136993,
-0.0399300768661818,-0.036638401707461,-0.0333021077236981,-0.0297950850530563,
-0.0251378361559023,-0.0157283595091443,-0.000701629447673439),
 .UNSPECIFIED.);
#989=B_SPLINE_CURVE_WITH_KNOTS('',3,(#71982,#71983,#71984,#71985,#71986,
#71987,#71988,#71989,#71990),.UNSPECIFIED.,.F.,.F.,(4,1,1,1,1,1,4),(91.106194480469,
91.4563736967383,92.4543904573498,93.4524072179613,94.4504239785728,95.4484407391843,
95.996079334354),.UNSPECIFIED.);
#990=B_SPLINE_CURVE_WITH_KNOTS('',3,(#71996,#71997,#71998,#71999,#72000,
#72001,#72002,#72003,#72004,#72005,#72006,#72007,#72008,#72009,#72010,#72011,
#72012,#72013,#72014,#72015,#72016,#72017,#72018,#72019,#72020,#72021,#72022,
#72023,#72024,#72025,#72026,#72027,#72028,#72029,#72030,#72031,#72032,#72033,
#72034,#72035,#72036,#72037,#72038,#72039,#72040,#72041,#72042,#72043,#72044,
#72045,#72046,#72047,#72048,#72049,#72050,#72051,#72052,#72053,#72054,#72055,
#72056,#72057,#72058,#72059,#72060,#72061,#72062,#72063,#72064,#72065,#72066,
#72067,#72068,#72069,#72070,#72071,#72072,#72073,#72074,#72075,#72076,#72077,
#72078,#72079,#72080,#72081,#72082,#72083,#72084,#72085,#72086,#72087,#72088,
#72089,#72090,#72091,#72092,#72093,#72094,#72095,#72096,#72097,#72098,#72099,
#72100,#72101,#72102,#72103,#72104,#72105,#72106,#72107,#72108,#72109,#72110,
#72111,#72112,#72113,#72114,#72115,#72116,#72117,#72118,#72119,#72120,#72121,
#72122,#72123,#72124,#72125,#72126,#72127,#72128,#72129,#72130,#72131,#72132,
#72133,#72134,#72135,#72136,#72137,#72138,#72139,#72140,#72141,#72142,#72143,
#72144,#72145,#72146,#72147,#72148,#72149,#72150,#72151,#72152,#72153,#72154,
#72155,#72156,#72157,#72158,#72159,#72160,#72161,#72162,#72163,#72164,#72165,
#72166,#72167),.UNSPECIFIED.,.F.,.F.,(4,2,2,2,2,2,2,2,2,2,2,2,2,2,2,2,2,
2,2,2,2,2,2,2,2,2,2,2,2,2,2,2,2,2,2,2,2,2,2,2,2,2,2,2,2,2,2,2,2,2,2,2,2,
2,2,2,2,2,2,2,2,2,2,2,2,2,2,2,2,2,2,2,2,2,2,2,2,2,2,2,2,2,2,2,2,4),(-1.16377943473109,
-1.13667956176578,-1.13045090196268,-1.1279456124005,-1.12592484053518,
-1.12380580106815,-1.12045457308714,-1.1094381599184,-1.0897651603648,-1.07837264907427,
-1.02357821268739,-1.01431140261525,-1.00982843926737,-1.00630583920957,
-1.00236540661045,-0.99573873190497,-0.967402188916012,-0.935500534693839,
-0.89938622056169,-0.893125984467853,-0.890615367303459,-0.888593229381796,
-0.88647639381595,-0.883134968107134,-0.872208914988976,-0.852780266295189,
-0.839517205197489,-0.786439707263261,-0.777049210924262,-0.772542836982356,
-0.769017741164505,-0.765090934536453,-0.758526667461252,-0.7311704820101,
-0.698580374647938,-0.662014660086823,-0.655785011257002,-0.65327964941036,
-0.651258949256087,-0.649140146510012,-0.645789574347334,-0.634777923482864,
-0.615117180234838,-0.603599419819502,-0.548935353963225,-0.539658772994035,
-0.535174127642822,-0.531651547760321,-0.527712531956804,-0.521091618809152,
-0.492842901799532,-0.460881269876965,-0.424731042404923,-0.4184742426345,
-0.415964306041933,-0.413942439372104,-0.411825544199055,-0.408483428307811,
-0.3975496540837,-0.378099496376652,-0.338366396719334,-0.307799421267046,
-0.300912601073609,-0.296876512324182,-0.293367072107328,-0.289030057197502,
-0.280715454250318,-0.269957205264194,-0.24400137354993,-0.190223629223084,
-0.181909822594664,-0.178795673811416,-0.176933414545376,-0.174888038183566,
-0.171881907488153,-0.163947871844611,-0.133545860916829,-0.101653494706863,
-0.0705270088481122,-0.0636114617079553,-0.0595686484081738,-0.0560594453317889,
-0.0526885679464537,-0.0484540398396745,-0.0419619959446415,-0.000702059288745545),
 .UNSPECIFIED.);
#991=B_SPLINE_CURVE_WITH_KNOTS('',3,(#72168,#72169,#72170,#72171,#72172,
#72173),.UNSPECIFIED.,.F.,.F.,(4,1,1,4),(95.9956065629,96.1329524862131,
97.1309692468246,97.3893698744215),.UNSPECIFIED.);
#992=B_SPLINE_CURVE_WITH_KNOTS('',3,(#72175,#72176,#72177,#72178,#72179),
 .UNSPECIFIED.,.F.,.F.,(4,1,4),(95.996079334354,96.4464574997958,97.3893656567973),
 .UNSPECIFIED.);
#993=B_SPLINE_CURVE_WITH_KNOTS('',3,(#72180,#72181,#72182,#72183,#72184,
#72185,#72186,#72187,#72188,#72189,#72190,#72191,#72192,#72193,#72194,#72195,
#72196,#72197,#72198,#72199,#72200,#72201,#72202,#72203,#72204,#72205,#72206,
#72207,#72208,#72209,#72210,#72211,#72212,#72213,#72214,#72215,#72216,#72217,
#72218,#72219,#72220,#72221,#72222,#72223,#72224,#72225,#72226,#72227,#72228,
#72229,#72230,#72231,#72232,#72233,#72234,#72235,#72236,#72237,#72238,#72239,
#72240,#72241,#72242,#72243,#72244,#72245,#72246,#72247,#72248,#72249,#72250,
#72251,#72252,#72253,#72254,#72255,#72256,#72257,#72258,#72259,#72260,#72261,
#72262,#72263,#72264,#72265,#72266,#72267,#72268,#72269,#72270,#72271,#72272,
#72273,#72274,#72275,#72276,#72277,#72278,#72279,#72280,#72281,#72282,#72283,
#72284,#72285,#72286,#72287,#72288,#72289,#72290,#72291,#72292,#72293,#72294,
#72295,#72296,#72297,#72298,#72299,#72300,#72301,#72302,#72303,#72304,#72305,
#72306,#72307,#72308,#72309,#72310,#72311,#72312,#72313,#72314,#72315,#72316,
#72317,#72318,#72319,#72320,#72321,#72322,#72323,#72324,#72325,#72326,#72327,
#72328,#72329,#72330,#72331,#72332,#72333,#72334,#72335,#72336,#72337,#72338,
#72339,#72340,#72341,#72342,#72343,#72344,#72345,#72346,#72347,#72348,#72349,
#72350,#72351),.UNSPECIFIED.,.F.,.F.,(4,2,2,2,2,2,2,2,2,2,2,2,2,2,2,2,2,
2,2,2,2,2,2,2,2,2,2,2,2,2,2,2,2,2,2,2,2,2,2,2,2,2,2,2,2,2,2,2,2,2,2,2,2,
2,2,2,2,2,2,2,2,2,2,2,2,2,2,2,2,2,2,2,2,2,2,2,2,2,2,2,2,2,2,2,2,4),(-2.9892703890057,
-2.9823293267889,-2.97967926444857,-2.97770338579837,-2.97580400447087,
-2.97360337628722,-2.96987933182125,-2.95645419292063,-2.91212960597214,
-2.8740695662292,-2.86460074454386,-2.86008076832223,-2.85655543405299,
-2.85263904948626,-2.8461177294965,-2.82248807884642,-2.77601739515326,
-2.75581084499323,-2.74827323306626,-2.74440636965689,-2.74116897950214,
-2.73909314965936,-2.73707361416644,-2.73457056144009,-2.72835090623037,
-2.69180193695157,-2.65924650537483,-2.6318849924972,-2.62532228158849,
-2.62139680131418,-2.61787315794747,-2.6133690279307,-2.60398485832457,
-2.55077735558636,-2.53768969729674,-2.51818634582801,-2.50723441216217,
-2.50389097083125,-2.5017742459579,-2.49975343760858,-2.49724584057276,
-2.49099996339123,-2.45476888944137,-2.42267551461133,-2.39464810273235,
-2.38804253479454,-2.38410762668271,-2.38058561321519,-2.37609745008294,
-2.36679812367136,-2.31237591440713,-2.30059248280992,-2.28093059061991,
-2.26991997875084,-2.26657011535626,-2.26445190593492,-2.26243191603646,
-2.25992767356055,-2.2537019187108,-2.21712539431818,-2.18452001193097,
-2.15722547423224,-2.15066665133557,-2.14674175979895,-2.14321755657897,
-2.13871120606279,-2.12931677500273,-2.07625358640812,-2.06297462148709,
-2.04350718658637,-2.03256816030637,-2.02922589059238,-2.02710928228442,
-2.02508804232384,-2.02257934107501,-2.01632784170074,-1.98015906965377,
-1.94816786533809,-1.91999085337202,-1.9133754341131,-1.90943813318859,
-1.90591613654818,-1.90143095586146,-1.8921487475923,-1.83749295151946,
-1.82646872808304),.UNSPECIFIED.);
#994=B_SPLINE_CURVE_WITH_KNOTS('',3,(#72356,#72357,#72358,#72359,#72360,
#72361,#72362,#72363,#72364,#72365,#72366,#72367,#72368,#72369,#72370,#72371,
#72372,#72373,#72374,#72375,#72376,#72377,#72378,#72379,#72380,#72381,#72382,
#72383,#72384,#72385,#72386,#72387,#72388,#72389,#72390,#72391,#72392,#72393,
#72394,#72395,#72396,#72397,#72398,#72399,#72400,#72401,#72402,#72403,#72404,
#72405,#72406,#72407,#72408,#72409,#72410,#72411,#72412,#72413,#72414,#72415,
#72416,#72417,#72418,#72419,#72420,#72421,#72422,#72423,#72424,#72425,#72426,
#72427,#72428,#72429,#72430,#72431,#72432,#72433,#72434,#72435,#72436,#72437,
#72438,#72439,#72440,#72441,#72442,#72443,#72444,#72445,#72446,#72447,#72448,
#72449,#72450,#72451,#72452,#72453,#72454,#72455,#72456,#72457,#72458,#72459,
#72460,#72461,#72462,#72463,#72464,#72465,#72466,#72467,#72468,#72469,#72470,
#72471,#72472,#72473,#72474,#72475,#72476,#72477,#72478,#72479,#72480,#72481,
#72482,#72483,#72484,#72485,#72486,#72487,#72488,#72489,#72490,#72491,#72492,
#72493,#72494,#72495,#72496,#72497,#72498,#72499,#72500,#72501,#72502,#72503,
#72504,#72505,#72506,#72507,#72508,#72509,#72510,#72511,#72512,#72513,#72514,
#72515,#72516,#72517,#72518,#72519,#72520,#72521,#72522,#72523,#72524,#72525,
#72526,#72527,#72528,#72529,#72530,#72531,#72532,#72533,#72534,#72535,#72536,
#72537,#72538,#72539,#72540,#72541,#72542,#72543,#72544,#72545,#72546,#72547,
#72548,#72549,#72550,#72551,#72552,#72553,#72554,#72555,#72556,#72557,#72558,
#72559),.UNSPECIFIED.,.F.,.F.,(4,2,2,2,2,2,2,2,2,2,2,2,2,2,2,2,2,2,2,2,
2,2,2,2,2,2,2,2,2,2,2,2,2,2,2,2,2,2,2,2,2,2,2,2,2,2,2,2,2,2,2,2,2,2,2,2,
2,2,2,2,2,2,2,2,2,2,2,2,2,2,2,2,2,2,2,2,2,2,2,2,2,2,2,2,2,2,2,2,2,2,2,2,
2,2,2,2,2,2,2,2,2,4),(-2.65808389942519,-2.65277394623415,-2.59767167014398,
-2.58656866339038,-2.56685693963098,-2.55582781778381,-2.55247557922228,
-2.550356577752,-2.54833640780605,-2.54583249295435,-2.53961028581393,-2.50294823173905,
-2.47661926235894,-2.446461040162,-2.43800000313917,-2.43367490672409,-2.43016642202381,
-2.42612180169746,-2.41919665311614,-2.38786795491194,-2.33797449475571,
-2.31964093649969,-2.3157061076181,-2.31345871713196,-2.3114703727123,-2.30884098866981,
-2.30284015364627,-2.25592661949482,-2.21372771078657,-2.20220994318211,
-2.19732758064353,-2.19374794841591,-2.18998454726976,-2.18417468473529,
-2.16729995971609,-2.11538285120956,-2.09325134954899,-2.08136490569739,
-2.07792413295315,-2.07578549389969,-2.07377713317466,-2.07085765068759,
-2.06535387070975,-2.02023711114846,-2.00922190768722,-1.97601274821715,
-1.96476706798689,-1.95992981069991,-1.95635759988333,-1.95257850193309,
-1.94669594264607,-1.92923773811265,-1.87178701369637,-1.85398164354678,
-1.84703265287146,-1.84184670074219,-1.83934017996461,-1.83755738826615,
-1.83527732493811,-1.83130021278135,-1.81412985642557,-1.76387159699003,
-1.73164094020065,-1.72479917716338,-1.72081215389211,-1.71729694034793,
-1.71288903404803,-1.7043001195289,-1.64418347134513,-1.61950836537465,
-1.60678559081765,-1.60326461442913,-1.60110811297851,-1.59910890025017,
-1.59668888897386,-1.59052845049766,-1.54643273564435,-1.49514233000848,
-1.48852206849158,-1.48420538822187,-1.48069687628701,-1.47664459478316,
-1.46949997627083,-1.4294475624368,-1.39139830629019,-1.37070151275081,
-1.3665228907123,-1.36419720629851,-1.36222220233128,-1.35967134039627,
-1.35425453712602,-1.31035598933721,-1.2613934468669,-1.25276784104122,
-1.24835836250884,-1.24507586755536,-1.24146953271487,-1.23643819616118,
-1.22399226690946,-1.20591262178753,-1.17327852828172,-1.16377943473109),
 .UNSPECIFIED.);
#995=B_SPLINE_CURVE_WITH_KNOTS('',3,(#72560,#72561,#72562,#72563,#72564,
#72565,#72566,#72567,#72568,#72569,#72570,#72571,#72572,#72573,#72574,#72575,
#72576,#72577,#72578,#72579,#72580,#72581,#72582,#72583,#72584,#72585,#72586,
#72587,#72588,#72589,#72590,#72591,#72592,#72593,#72594,#72595,#72596,#72597,
#72598,#72599,#72600,#72601,#72602,#72603,#72604,#72605,#72606,#72607,#72608,
#72609,#72610,#72611,#72612,#72613,#72614,#72615,#72616,#72617,#72618,#72619,
#72620,#72621,#72622,#72623,#72624,#72625,#72626,#72627,#72628,#72629,#72630,
#72631,#72632,#72633,#72634,#72635,#72636,#72637,#72638,#72639,#72640,#72641,
#72642,#72643,#72644,#72645,#72646,#72647,#72648,#72649,#72650,#72651,#72652,
#72653,#72654,#72655,#72656,#72657,#72658,#72659,#72660,#72661,#72662,#72663,
#72664,#72665,#72666,#72667,#72668,#72669,#72670,#72671,#72672,#72673,#72674,
#72675,#72676,#72677,#72678,#72679,#72680,#72681,#72682,#72683,#72684,#72685,
#72686,#72687,#72688,#72689,#72690,#72691,#72692,#72693,#72694,#72695,#72696,
#72697,#72698,#72699,#72700,#72701,#72702,#72703,#72704,#72705,#72706,#72707,
#72708,#72709,#72710,#72711,#72712,#72713,#72714,#72715,#72716,#72717,#72718,
#72719,#72720,#72721,#72722,#72723,#72724,#72725,#72726,#72727,#72728,#72729,
#72730,#72731,#72732,#72733,#72734,#72735,#72736,#72737,#72738,#72739,#72740,
#72741,#72742,#72743,#72744,#72745,#72746,#72747,#72748,#72749,#72750,#72751,
#72752,#72753,#72754,#72755,#72756,#72757,#72758,#72759,#72760,#72761,#72762,
#72763,#72764,#72765,#72766,#72767,#72768,#72769,#72770,#72771,#72772,#72773),
 .UNSPECIFIED.,.F.,.F.,(4,2,2,2,2,2,2,2,2,2,2,2,2,2,2,2,2,2,2,2,2,2,2,2,
2,2,2,2,2,2,2,2,2,2,2,2,2,2,2,2,2,2,2,2,2,2,2,2,2,2,2,2,2,2,2,2,2,2,2,2,
2,2,2,2,2,2,2,2,2,2,2,2,2,2,2,2,2,2,2,2,2,2,2,2,2,2,2,2,2,2,2,2,2,2,2,2,
2,2,2,2,2,2,2,2,2,2,4),(-1.82646872808304,-1.79734343065746,-1.79282236795917,
-1.7904500083226,-1.78847942728732,-1.78599002003742,-1.78201728957643,
-1.75740049756953,-1.72082841589016,-1.68574819720403,-1.67732653125684,
-1.67300951028283,-1.66950177302835,-1.66545157743265,-1.65850096993108,
-1.62665625488312,-1.57722097813993,-1.55895366761575,-1.55502285629584,
-1.55277644485429,-1.55078807283716,-1.54815756432633,-1.54214968319553,
-1.49535134001273,-1.45027218291409,-1.44062165500393,-1.4361156264914,
-1.43258176884484,-1.42869602973701,-1.42231921516799,-1.39762001860241,
-1.36847462436808,-1.32516309212689,-1.31896620803045,-1.31654077706124,
-1.31454058610643,-1.312387495636,-1.30888058536324,-1.29630354879562,-1.27208731332166,
-1.21120538561776,-1.20346749532008,-1.19887023285559,-1.19532358250096,
-1.19148257080471,-1.18531097264309,-1.16313173827444,-1.12402804327183,
-1.08802186722329,-1.08178777524824,-1.07928191376428,-1.07726132907201,
-1.07514334239209,-1.07179534149392,-1.06080427782233,-1.04119906276471,
-1.02901769956693,-0.974997981890985,-0.965670356047288,-0.961176469496914,
-0.95765342988398,-0.9537209616307,-0.94712815723658,-0.919316518239307,
-0.88703245040185,-0.850673363228459,-0.844431342045032,-0.841924176859279,
-0.839903291338221,-0.837785920917063,-0.834440514550907,-0.823472911130825,
-0.803930938430001,-0.791229216561297,-0.737695413856313,-0.728334089761734,
-0.723833895929693,-0.720310249841019,-0.716381585360781,-0.709805932497879,
-0.6822595032286,-0.649792237898696,-0.61331073220674,-0.607076629892004,
-0.604570860569829,-0.602550388610375,-0.600432567798541,-0.597084912150998,
-0.586095749011207,-0.566495024707679,-0.55428458656948,-0.500296910439677,
-0.490967807783343,-0.486473817723689,-0.482950963349569,-0.47901897748105,
-0.472427645952877,-0.444634221868152,-0.412340686353847,-0.375976390572374,
-0.369735288842809,-0.367228374182216,-0.36520764329194,-0.363090376161521,
-0.359745030876317,-0.348776687020761,-0.332074222475645),.UNSPECIFIED.);
#996=B_SPLINE_CURVE_WITH_KNOTS('',3,(#72779,#72780,#72781,#72782,#72783,
#72784,#72785,#72786,#72787),.UNSPECIFIED.,.F.,.F.,(4,1,1,1,1,1,4),(109.955742875643,
110.105187134774,111.103203895386,112.101220655997,113.099237416609,114.09725417722,
114.844983025569),.UNSPECIFIED.);
#997=B_SPLINE_CURVE_WITH_KNOTS('',3,(#72788,#72789,#72790,#72791,#72792,
#72793,#72794,#72795,#72796,#72797,#72798,#72799,#72800,#72801,#72802,#72803,
#72804,#72805,#72806,#72807,#72808,#72809,#72810,#72811,#72812,#72813,#72814,
#72815,#72816,#72817,#72818,#72819,#72820,#72821,#72822,#72823,#72824,#72825,
#72826,#72827,#72828,#72829,#72830,#72831,#72832,#72833,#72834,#72835,#72836,
#72837),.UNSPECIFIED.,.F.,.F.,(4,2,2,2,2,2,2,2,2,2,2,2,2,2,2,2,2,2,2,2,
2,2,2,2,4),(-2.98948394067237,-2.93033327020979,-2.920244048379,-2.91226142318022,
-2.90803374835732,-2.9045631617174,-2.9004520241019,-2.89322997407042,-2.84953099677671,
-2.81256119808136,-2.80026151844069,-2.79237614375237,-2.78948716317769,
-2.78764833673942,-2.78562791237046,-2.78312274318819,-2.7768927054734,
-2.74083011361301,-2.70912061365899,-2.6805950398033,-2.67395791026974,
-2.67001567319296,-2.66649418458564,-2.6620163632797,-2.65808389942519),
 .UNSPECIFIED.);
#998=B_SPLINE_CURVE_WITH_KNOTS('',3,(#72839,#72840,#72841,#72842,#72843,
#72844,#72845,#72846,#72847,#72848,#72849,#72850,#72851,#72852,#72853,#72854,
#72855,#72856,#72857,#72858,#72859,#72860,#72861,#72862,#72863,#72864,#72865,
#72866,#72867,#72868,#72869,#72870,#72871,#72872,#72873,#72874,#72875,#72876,
#72877,#72878,#72879,#72880,#72881,#72882,#72883,#72884,#72885,#72886,#72887,
#72888,#72889,#72890,#72891,#72892),.UNSPECIFIED.,.F.,.F.,(4,2,2,2,2,2,
2,2,2,2,2,2,2,2,2,2,2,2,2,2,2,2,2,2,2,2,4),(-0.332074222475645,-0.32923204910345,
-0.318830590678436,-0.262639008314075,-0.253697656003321,-0.249176719081695,
-0.245807769776908,-0.242024917996104,-0.238071186744742,-0.232264168229582,
-0.190630465007277,-0.146639547020774,-0.134181037306488,-0.130549452041593,
-0.128369040640389,-0.126359289402557,-0.123541320311572,-0.116588668380137,
-0.106358990090594,-0.0724794716636102,-0.0352996703932748,-0.0192230682661245,
-0.0136314931449329,-0.00986943951079496,-0.00651983590288715,-0.00346048099933967,
-0.000736392770504616),.UNSPECIFIED.);
#999=B_SPLINE_CURVE_WITH_KNOTS('',3,(#72893,#72894,#72895,#72896,#72897,
#72898,#72899,#72900,#72901),.UNSPECIFIED.,.F.,.F.,(4,1,1,1,1,1,4),(109.955745615411,
110.418692148357,111.416708908968,112.41472566958,113.412742430191,114.410759190803,
114.846231128118),.UNSPECIFIED.);
#1000=B_SPLINE_CURVE_WITH_KNOTS('',3,(#72907,#72908,#72909,#72910,#72911,
#72912,#72913,#72914,#72915,#72916,#72917,#72918,#72919,#72920,#72921,#72922,
#72923,#72924,#72925,#72926,#72927,#72928,#72929,#72930,#72931,#72932,#72933,
#72934,#72935,#72936,#72937,#72938,#72939,#72940,#72941,#72942,#72943,#72944,
#72945,#72946,#72947,#72948,#72949,#72950,#72951,#72952,#72953,#72954,#72955,
#72956,#72957,#72958,#72959,#72960,#72961,#72962,#72963,#72964,#72965,#72966,
#72967,#72968,#72969,#72970,#72971,#72972,#72973,#72974,#72975,#72976,#72977,
#72978,#72979,#72980,#72981,#72982,#72983,#72984,#72985,#72986,#72987,#72988,
#72989,#72990,#72991,#72992,#72993,#72994,#72995,#72996,#72997,#72998,#72999,
#73000,#73001,#73002,#73003,#73004,#73005,#73006,#73007,#73008,#73009,#73010,
#73011,#73012,#73013,#73014,#73015,#73016,#73017,#73018,#73019,#73020,#73021,
#73022,#73023,#73024,#73025,#73026,#73027,#73028,#73029,#73030,#73031,#73032,
#73033,#73034,#73035,#73036,#73037,#73038,#73039,#73040,#73041,#73042,#73043,
#73044,#73045,#73046,#73047,#73048,#73049,#73050,#73051,#73052,#73053,#73054,
#73055,#73056,#73057,#73058,#73059,#73060,#73061,#73062,#73063,#73064,#73065,
#73066),.UNSPECIFIED.,.F.,.F.,(4,2,2,2,2,2,2,2,2,2,2,2,2,2,2,2,2,2,2,2,
2,2,2,2,2,2,2,2,2,2,2,2,2,2,2,2,2,2,2,2,2,2,2,2,2,2,2,2,2,2,2,2,2,2,2,2,
2,2,2,2,2,2,2,2,2,2,2,2,2,2,2,2,2,2,2,2,2,2,2,4),(-1.16399522342669,-1.1607907650581,
-1.15676753883012,-1.15426290904758,-1.15229142577373,-1.14993129837991,
-1.14546917568034,-1.11123091791317,-1.05385890063992,-1.04263838798745,
-1.03816444188207,-1.03486673191996,-1.03127542050177,-1.02632369629155,
-1.01437727086931,-0.997276965565523,-0.930525489122616,-0.92115957748363,
-0.917892990164741,-0.916001193627688,-0.913980141959651,-0.911101445563391,
-0.903766126285405,-0.892768033335116,-0.82025015374059,-0.806202941365025,
-0.800779737705798,-0.797465144405553,-0.793885294240733,-0.789003323779566,
-0.777489870506518,-0.735403155294618,-0.688311462055666,-0.682317213195112,
-0.679688716305464,-0.677700279848191,-0.675451921571445,-0.671513237591417,
-0.653115374970274,-0.602768451457007,-0.571962960154127,-0.565063896818231,
-0.561024964452434,-0.557515663186227,-0.553182178311967,-0.54468038352206,
-0.514227530682404,-0.473045419646851,-0.448495708181078,-0.444525426127836,
-0.442036568138941,-0.4400657108176,-0.437692089561676,-0.433166056534365,
-0.391822425520439,-0.338592459043075,-0.329212056146974,-0.324707748331981,
-0.32118305990655,-0.317255462249331,-0.310686891688175,-0.283260623549618,
-0.25071953658601,-0.214191025847954,-0.20795896562446,-0.205453268244515,
-0.203432551722216,-0.201356549782399,-0.198286203347804,-0.18890777918587,
-0.173270510740528,-0.138720380485088,-0.097876263984719,-0.0906666070068624,
-0.0865578429595567,-0.083086582079581,-0.0788547987316751,-0.0708542543693418,
-0.0607355454979825,-0.000706686318606294),.UNSPECIFIED.);
#1001=B_SPLINE_CURVE_WITH_KNOTS('',3,(#73067,#73068,#73069,#73070,#73071,
#73072),.UNSPECIFIED.,.F.,.F.,(4,1,1,4),(114.844983025569,115.095270937832,
116.093287698443,116.238928182822),.UNSPECIFIED.);
#1002=B_SPLINE_CURVE_WITH_KNOTS('',3,(#73074,#73075,#73076,#73077,#73078),
 .UNSPECIFIED.,.F.,.F.,(4,1,4),(114.846231128118,115.408775951414,116.238922116759),
 .UNSPECIFIED.);
#1003=B_SPLINE_CURVE_WITH_KNOTS('',3,(#73079,#73080,#73081,#73082,#73083,
#73084,#73085,#73086,#73087,#73088,#73089,#73090,#73091,#73092,#73093,#73094,
#73095,#73096,#73097,#73098,#73099,#73100,#73101,#73102,#73103,#73104,#73105,
#73106,#73107,#73108,#73109,#73110,#73111,#73112,#73113,#73114,#73115,#73116,
#73117,#73118,#73119,#73120,#73121,#73122,#73123,#73124,#73125,#73126,#73127,
#73128,#73129,#73130,#73131,#73132,#73133,#73134,#73135,#73136,#73137,#73138,
#73139,#73140,#73141,#73142,#73143,#73144,#73145,#73146,#73147,#73148,#73149,
#73150,#73151,#73152,#73153,#73154,#73155,#73156,#73157,#73158,#73159,#73160,
#73161,#73162,#73163,#73164,#73165,#73166),.UNSPECIFIED.,.F.,.F.,(4,3,3,
3,3,3,3,3,3,3,3,3,3,3,3,3,3,3,3,3,3,3,3,3,3,3,3,3,3,4),(116.238928182822,
116.406792712026,116.585455131904,116.763755652497,116.942027621902,117.120269763611,
117.298929207096,117.404809472637,117.583471744362,117.761772116778,117.940043940156,
118.118285936843,118.296945239705,118.402826233249,118.581488643105,118.759789151972,
118.938061107338,119.116303233685,119.294962660085,119.40084299386,119.579505658284,
119.757806425289,119.936078640185,120.114321027218,120.292980710927,120.398859754472,
120.581274217561,120.759594008658,120.944055807743,121.128517606828),
 .UNSPECIFIED.);
#1004=B_SPLINE_CURVE_WITH_KNOTS('',3,(#73171,#73172,#73173,#73174,#73175,
#73176,#73177,#73178,#73179,#73180,#73181,#73182,#73183,#73184,#73185,#73186,
#73187,#73188,#73189,#73190,#73191,#73192,#73193,#73194,#73195,#73196,#73197,
#73198,#73199,#73200,#73201,#73202,#73203,#73204,#73205,#73206,#73207,#73208,
#73209,#73210,#73211,#73212,#73213,#73214,#73215,#73216,#73217,#73218,#73219,
#73220,#73221,#73222,#73223,#73224,#73225,#73226,#73227,#73228,#73229,#73230,
#73231,#73232,#73233,#73234,#73235,#73236,#73237,#73238,#73239,#73240,#73241,
#73242,#73243,#73244,#73245,#73246,#73247,#73248,#73249,#73250,#73251,#73252,
#73253,#73254,#73255,#73256,#73257,#73258,#73259,#73260,#73261,#73262,#73263,
#73264,#73265,#73266,#73267,#73268,#73269,#73270,#73271,#73272,#73273,#73274,
#73275,#73276,#73277,#73278,#73279,#73280,#73281,#73282,#73283,#73284,#73285,
#73286,#73287,#73288,#73289,#73290,#73291,#73292,#73293,#73294,#73295,#73296,
#73297,#73298,#73299,#73300,#73301,#73302,#73303,#73304,#73305,#73306,#73307,
#73308,#73309,#73310,#73311,#73312,#73313,#73314,#73315,#73316,#73317,#73318,
#73319,#73320,#73321,#73322,#73323,#73324,#73325,#73326,#73327,#73328,#73329,
#73330,#73331,#73332,#73333,#73334,#73335,#73336,#73337,#73338,#73339,#73340,
#73341,#73342,#73343,#73344,#73345,#73346,#73347,#73348,#73349,#73350,#73351,
#73352,#73353,#73354,#73355,#73356,#73357,#73358,#73359,#73360,#73361,#73362,
#73363,#73364,#73365,#73366,#73367,#73368,#73369,#73370,#73371,#73372,#73373,
#73374,#73375,#73376,#73377,#73378),.UNSPECIFIED.,.F.,.F.,(4,2,2,2,2,2,
2,2,2,2,2,2,2,2,2,2,2,2,2,2,2,2,2,2,2,2,2,2,2,2,2,2,2,2,2,2,2,2,2,2,2,2,
2,2,2,2,2,2,2,2,2,2,2,2,2,2,2,2,2,2,2,2,2,2,2,2,2,2,2,2,2,2,2,2,2,2,2,2,
2,2,2,2,2,2,2,2,2,2,2,2,2,2,2,2,2,2,2,2,2,2,2,2,2,4),(-2.65819190440258,
-2.62705712494929,-2.59765357301862,-2.58818230394141,-2.58161464612472,
-2.57885718035791,-2.57685785746737,-2.57466372827504,-2.5709336624315,
-2.55727162657967,-2.54405129398292,-2.47891151641061,-2.46682567394425,
-2.46187307468181,-2.45830137698401,-2.45503587890549,-2.44978666843108,
-2.43675119578249,-2.38090755497794,-2.34715072372975,-2.34271887739022,
-2.34037695799276,-2.33841168866653,-2.33591020129654,-2.33189890701069,
-2.30470322282034,-2.26384368335237,-2.2327840173422,-2.22599043099554,
-2.22200752389696,-2.21848128088368,-2.21403969471864,-2.20531968773966,
-2.14666080293568,-2.12140817522014,-2.10850181955546,-2.10495478144744,
-2.10278655601613,-2.10078436366636,-2.09836423134815,-2.0922148311029,
-2.04793545909769,-2.01339516524246,-2.00059679224079,-1.99099412388749,
-1.9864466300786,-1.98291529562836,-1.97900793568737,-1.97253857652236,
-1.94990948815999,-1.90286790921321,-1.87265483895183,-1.86826625704765,
-1.86592166981243,-1.86395007102146,-1.86142839572219,-1.85734437447908,
-1.82219968803482,-1.7789745800374,-1.764531840932,-1.75400383553291,-1.74929267610803,
-1.74574325456806,-1.74192173749601,-1.73583077706982,-1.71653868529926,
-1.66672544670334,-1.63530910422094,-1.63089788175895,-1.62854973302512,
-1.62657798490348,-1.6240605864961,-1.61999570653607,-1.58957505440082,
-1.58367800376849,-1.58132498720718,-1.55052706117888,-1.52092595187713,
-1.51422201415437,-1.51026361139447,-1.50674208454562,-1.50228372944685,
-1.49519565036645,-1.485286693889,-1.46243578350789,-1.4346822666082,-1.42708549562084,
-1.39817940851973,-1.39413512429057,-1.39162316200219,-1.38965010783394,
-1.38729312070076,-1.38284848244978,-1.3497909124847,-1.29568288511291,
-1.28120802408501,-1.27572128797448,-1.27239497228259,-1.26882314854165,
-1.2639889239166,-1.25276219547068,-1.2205778578495,-1.18863953479716,-1.16399522342669),
 .UNSPECIFIED.);
#1005=B_SPLINE_CURVE_WITH_KNOTS('',3,(#73380,#73381,#73382,#73383,#73384,
#73385,#73386,#73387,#73388,#73389,#73390,#73391,#73392,#73393,#73394,#73395,
#73396,#73397,#73398,#73399,#73400,#73401,#73402,#73403,#73404,#73405,#73406,
#73407),.UNSPECIFIED.,.F.,.F.,(4,3,3,3,3,3,3,3,3,4),(121.128517606828,121.307176749353,
121.396876515083,121.575539354439,121.753840284705,121.932112643433,122.110355163549,
122.289014961266,122.394893275695,122.522113490002),.UNSPECIFIED.);
#1006=B_SPLINE_CURVE_WITH_KNOTS('',3,(#73408,#73409,#73410,#73411,#73412,
#73413,#73414,#73415,#73416,#73417,#73418,#73419,#73420,#73421,#73422,#73423,
#73424,#73425,#73426,#73427,#73428,#73429,#73430,#73431,#73432,#73433,#73434,
#73435,#73436,#73437,#73438,#73439,#73440,#73441,#73442,#73443,#73444,#73445,
#73446,#73447,#73448,#73449,#73450,#73451,#73452,#73453,#73454,#73455,#73456,
#73457,#73458,#73459,#73460,#73461,#73462,#73463,#73464,#73465,#73466,#73467,
#73468,#73469,#73470,#73471,#73472,#73473,#73474,#73475,#73476,#73477,#73478,
#73479,#73480,#73481,#73482,#73483,#73484,#73485,#73486,#73487,#73488,#73489,
#73490,#73491,#73492,#73493,#73494,#73495,#73496,#73497,#73498,#73499,#73500,
#73501,#73502,#73503,#73504,#73505,#73506,#73507,#73508,#73509,#73510,#73511,
#73512,#73513,#73514,#73515,#73516,#73517,#73518,#73519,#73520,#73521,#73522,
#73523,#73524,#73525,#73526,#73527,#73528,#73529,#73530,#73531,#73532,#73533,
#73534,#73535,#73536,#73537,#73538,#73539,#73540,#73541,#73542,#73543,#73544,
#73545,#73546,#73547,#73548,#73549,#73550,#73551,#73552,#73553,#73554,#73555,
#73556,#73557,#73558,#73559,#73560,#73561,#73562,#73563,#73564,#73565,#73566,
#73567,#73568,#73569,#73570,#73571,#73572,#73573,#73574,#73575,#73576,#73577,
#73578,#73579),.UNSPECIFIED.,.F.,.F.,(4,2,2,2,2,2,2,2,2,2,2,2,2,2,2,2,2,
2,2,2,2,2,2,2,2,2,2,2,2,2,2,2,2,2,2,2,2,2,2,2,2,2,2,2,2,2,2,2,2,2,2,2,2,
2,2,2,2,2,2,2,2,2,2,2,2,2,2,2,2,2,2,2,2,2,2,2,2,2,2,2,2,2,2,2,2,4),(1.16375694728592,
1.16380572379371,1.16756314774595,1.16977105475773,1.17176855571367,1.17451819235809,
1.18106226091327,1.19049733908575,1.21977817780083,1.27257455330762,1.28198220795045,
1.28648837836552,1.29000951314699,1.29392790987802,1.30046832523159,1.32754326642328,
1.36036792674952,1.39703180321458,1.40325307475061,1.40575526496874,1.40777345122844,
1.40989154291943,1.41324007375119,1.42423574989435,1.44385599928274,1.45602068439686,
1.51009100934789,1.51942029204224,1.52391532427349,1.52743943895535,1.53137332141279,
1.53796913868854,1.56581731978394,1.59800829457104,1.63428741328967,1.64052917013522,
1.64303692870204,1.64505862845649,1.64717646704278,1.65052381119274,1.66150847642566,
1.68109953840757,1.69354314423061,1.74731784145461,1.75666325606489,1.7611601238046,
1.76468304513515,1.76861284203001,1.77519506653898,1.80285485901953,1.83521594225092,
1.87162355399383,1.87785781582318,1.88036323445556,1.88238327569664,1.88450030533758,
1.88784628997681,1.89882542779452,1.91840370721812,1.93098657621613,1.98463441923818,
1.99398879792609,1.99848679136185,2.00200918517096,2.00593692917007,2.01251217539737,
2.04007898461954,2.07249460519876,2.10894638508053,2.11517037862647,2.11767394279111,
2.11969338955896,2.12176873444242,2.12485030980061,2.12860467378489,2.13582880444578,
2.15473808286976,2.16252615307732,2.22309145171865,2.23161895358931,2.23601272974263,
2.23952516454979,2.24351815164137,2.25039323963597,2.28336705928181,2.32678697888738),
 .UNSPECIFIED.);
#1007=B_SPLINE_CURVE_WITH_KNOTS('',3,(#73583,#73584,#73585,#73586,#73587,
#73588,#73589,#73590,#73591,#73592,#73593,#73594,#73595,#73596,#73597,#73598,
#73599,#73600,#73601,#73602,#73603,#73604,#73605,#73606,#73607,#73608,#73609,
#73610,#73611,#73612,#73613,#73614,#73615,#73616,#73617,#73618,#73619,#73620,
#73621,#73622),.UNSPECIFIED.,.F.,.F.,(4,3,3,3,3,3,3,3,3,3,3,3,3,4),(-4.09293042013065,
-3.992067042446,-3.82244776231553,-3.65315968078964,-3.48390880876262,-3.31470709998066,
-3.14511254726307,-2.9940502818345,-2.82636267585639,-2.65899488979554,
-2.49165994935383,-2.32435113337687,-2.15669226772051,-2.06882272292704),
 .UNSPECIFIED.);
#1008=B_SPLINE_CURVE_WITH_KNOTS('',3,(#73626,#73627,#73628,#73629,#73630,
#73631,#73632,#73633,#73634,#73635,#73636,#73637,#73638,#73639,#73640,#73641,
#73642,#73643,#73644,#73645,#73646,#73647),.UNSPECIFIED.,.F.,.F.,(4,3,3,
3,3,3,3,4),(4.61444669507962E-15,0.17333570362943,0.346547214765417,0.519954753279274,
0.693441640210306,0.867424673888169,0.998016760611494,1.11730040836813),
 .UNSPECIFIED.);
#1009=B_SPLINE_CURVE_WITH_KNOTS('',3,(#73649,#73650,#73651,#73652,#73653,
#73654,#73655,#73656,#73657,#73658,#73659,#73660,#73661,#73662,#73663,#73664,
#73665,#73666,#73667,#73668,#73669,#73670,#73671,#73672,#73673,#73674,#73675,
#73676,#73677,#73678,#73679,#73680,#73681,#73682,#73683,#73684,#73685,#73686,
#73687,#73688,#73689,#73690,#73691,#73692,#73693,#73694,#73695,#73696,#73697,
#73698,#73699,#73700,#73701,#73702,#73703,#73704,#73705,#73706,#73707,#73708,
#73709,#73710,#73711,#73712,#73713,#73714,#73715,#73716,#73717,#73718,#73719,
#73720,#73721,#73722,#73723,#73724,#73725,#73726,#73727,#73728,#73729,#73730,
#73731,#73732,#73733,#73734,#73735,#73736,#73737,#73738,#73739,#73740,#73741,
#73742,#73743,#73744,#73745,#73746,#73747,#73748,#73749,#73750,#73751,#73752,
#73753,#73754,#73755,#73756,#73757,#73758,#73759,#73760,#73761,#73762,#73763,
#73764,#73765,#73766),.UNSPECIFIED.,.F.,.F.,(4,3,3,3,3,3,3,3,3,3,3,3,3,
3,3,3,3,3,3,3,3,3,3,3,3,3,3,3,3,3,3,3,3,3,3,3,3,3,3,4),(1.11730040857138,
1.28258742205918,1.4475801664024,1.61257569629296,1.77757610156023,1.94293553368316,
1.996033521223,2.16557749727504,2.33479223618305,2.50397357895414,2.67310773704729,
2.84263918138715,2.9940502818345,3.16364173365622,3.33291309222664,3.50216444093724,
3.67137606968638,3.84099599146778,3.992067042446,4.16113100258707,4.32986127689689,
4.49855861854032,4.66720816578798,4.83626436321027,4.9900838030575,5.15942585196637,
5.32843906253154,5.49742264590328,5.66636077829777,5.83570339435669,5.988100563669,
6.15742914576441,6.32642978538965,6.49540238342449,6.66433038075115,6.83366451994832,
6.9861173242805,7.17227412937206,7.35714291321279,7.40048531495325),
 .UNSPECIFIED.);
#1010=B_SPLINE_CURVE_WITH_KNOTS('',3,(#73768,#73769,#73770,#73771,#73772,
#73773,#73774,#73775,#73776,#73777),.UNSPECIFIED.,.F.,.F.,(4,1,1,1,1,1,
1,4),(7.40048571554771,7.984134084892,8.98215084550351,9.98016760611501,
10.9781843667265,11.976201127338,12.9742178879495,13.6836710227273),
 .UNSPECIFIED.);
#1011=B_SPLINE_CURVE_WITH_KNOTS('',3,(#73779,#73780,#73781,#73782,#73783,
#73784,#73785,#73786,#73787,#73788,#73789,#73790,#73791,#73792,#73793,#73794,
#73795,#73796,#73797,#73798,#73799,#73800,#73801,#73802,#73803,#73804,#73805,
#73806,#73807,#73808,#73809,#73810,#73811,#73812,#73813,#73814,#73815,#73816,
#73817,#73818,#73819,#73820,#73821,#73822,#73823,#73824,#73825,#73826,#73827,
#73828,#73829,#73830,#73831,#73832,#73833,#73834,#73835,#73836,#73837,#73838,
#73839,#73840,#73841,#73842,#73843,#73844,#73845,#73846,#73847,#73848,#73849,
#73850,#73851,#73852,#73853,#73854,#73855,#73856,#73857,#73858,#73859,#73860,
#73861,#73862,#73863,#73864,#73865,#73866,#73867,#73868,#73869,#73870,#73871,
#73872,#73873,#73874,#73875,#73876,#73877,#73878,#73879,#73880,#73881,#73882,
#73883,#73884,#73885,#73886,#73887,#73888,#73889,#73890,#73891,#73892,#73893,
#73894,#73895,#73896),.UNSPECIFIED.,.F.,.F.,(4,3,3,3,3,3,3,3,3,3,3,3,3,
3,3,3,3,3,3,3,3,3,3,3,3,3,3,3,3,3,3,3,3,3,3,3,3,3,3,4),(13.6836711800844,
13.8911898125104,13.972234648561,14.1415281762225,14.3104926228966,14.4794278048088,
14.6483176482061,14.8176131987297,14.9702514091725,15.1395446921665,15.3085088919621,
15.4774438272913,15.6463334238238,15.8156287322797,15.968268169784,16.137561335811,
16.3065254144919,16.4754602240832,16.6443496921161,16.8136448701357,16.9662849303955,
17.1355782298889,17.3045424449965,17.4734773935573,17.6423670022045,17.8116623206224,
17.964301691007,18.1335949468184,18.302559117701,18.4714940218612,18.6403835859313,
18.8096788604258,18.9623184516185,19.1316116956298,19.3005758542088,19.4695107454679,
19.6384002962861,19.807695557217,19.96033521223,19.9668563299069),
 .UNSPECIFIED.);
#1012=B_SPLINE_CURVE_WITH_KNOTS('',3,(#73898,#73899,#73900,#73901,#73902,
#73903,#73904,#73905,#73906,#73907,#73908,#73909,#73910,#73911,#73912,#73913,
#73914,#73915,#73916,#73917,#73918,#73919,#73920,#73921,#73922,#73923,#73924,
#73925,#73926,#73927,#73928,#73929,#73930,#73931,#73932,#73933,#73934,#73935,
#73936,#73937,#73938,#73939,#73940,#73941,#73942,#73943,#73944,#73945,#73946,
#73947,#73948,#73949,#73950,#73951,#73952,#73953,#73954,#73955,#73956,#73957,
#73958,#73959,#73960,#73961,#73962,#73963,#73964,#73965,#73966,#73967,#73968,
#73969,#73970,#73971,#73972,#73973,#73974,#73975,#73976,#73977,#73978,#73979,
#73980,#73981,#73982,#73983,#73984,#73985,#73986,#73987,#73988,#73989,#73990,
#73991,#73992,#73993,#73994,#73995,#73996,#73997,#73998,#73999,#74000,#74001,
#74002,#74003,#74004,#74005,#74006,#74007,#74008,#74009,#74010,#74011,#74012),
 .UNSPECIFIED.,.F.,.F.,(4,3,3,3,3,3,3,3,3,3,3,3,3,3,3,3,3,3,3,3,3,3,3,3,
3,3,3,3,3,3,3,3,3,3,3,3,3,3,4),(19.9668563300962,20.135952811592,20.3047208147562,
20.4734598895618,20.6421556318704,20.8112536713725,20.9583519728415,21.1276452281632,
21.2966093983786,21.4655443016053,21.6344338645944,21.8037291377806,21.956368733453,
22.1256619878341,22.2946261570513,22.4635610592055,22.6324506210793,22.8017458931016,
22.9543854940645,23.1236787509982,23.2926429228304,23.4615778276573,23.6304673922401,
23.7997626669753,23.952402254676,24.1216955104188,24.2906596810405,24.4595945846445,
24.6284841479956,24.7977794215101,24.9504190152875,25.1197122710063,25.2886764415981,
25.4576113451634,25.6265009084708,25.7957961819343,25.948435775899,26.1527578523688,
26.2500414524452),.UNSPECIFIED.);
#1013=B_SPLINE_CURVE_WITH_KNOTS('',3,(#74014,#74015,#74016,#74017,#74018,
#74019,#74020,#74021,#74022,#74023),.UNSPECIFIED.,.F.,.F.,(4,1,1,1,1,1,
1,4),(26.2500416370865,26.9464525365105,27.944469297122,28.9424860577335,
29.940502818345,30.9385195789565,31.936536339568,32.5332269442661),
 .UNSPECIFIED.);
#1014=B_SPLINE_CURVE_WITH_KNOTS('',3,(#74025,#74026,#74027,#74028,#74029,
#74030,#74031,#74032,#74033,#74034,#74035,#74036,#74037,#74038,#74039,#74040,
#74041,#74042,#74043,#74044,#74045,#74046,#74047,#74048,#74049,#74050,#74051,
#74052,#74053,#74054,#74055,#74056,#74057,#74058,#74059,#74060,#74061,#74062,
#74063,#74064,#74065,#74066,#74067,#74068,#74069,#74070,#74071,#74072,#74073,
#74074,#74075,#74076,#74077,#74078,#74079,#74080,#74081,#74082,#74083,#74084,
#74085,#74086,#74087,#74088,#74089,#74090,#74091,#74092,#74093,#74094,#74095,
#74096,#74097,#74098,#74099,#74100,#74101,#74102,#74103,#74104,#74105,#74106,
#74107,#74108,#74109,#74110,#74111,#74112,#74113,#74114,#74115,#74116,#74117,
#74118,#74119,#74120,#74121,#74122,#74123,#74124,#74125,#74126,#74127,#74128,
#74129,#74130,#74131,#74132,#74133,#74134,#74135,#74136,#74137,#74138,#74139,
#74140,#74141,#74142),.UNSPECIFIED.,.F.,.F.,(4,3,3,3,3,3,3,3,3,3,3,3,3,
3,3,3,3,3,3,3,3,3,3,3,3,3,3,3,3,3,3,3,3,3,3,3,3,3,3,4),(32.5332271627877,
32.7196079893562,32.9074239211681,32.9345531001795,33.1038463560855,33.2728105268702,
33.4417454306341,33.6106349941438,33.7799302678113,33.932569860791,34.1018631166979,
34.2708272874833,34.4397621912481,34.6086517547587,34.7779470284269,34.9305866214025,
35.09987987731,35.2688440480961,35.4377789518616,35.6066685153728,35.7759637890418,
35.928603382014,36.0978966379209,36.2668608087064,36.4357957124713,36.6046852759818,
36.7739805496502,36.9266201426255,37.0959133985326,37.2648775693182,37.4338124730832,
37.602702036594,37.7719973102625,37.924636903237,38.0917435228824,38.258524840331,
38.4252546296913,38.5919573763902,38.758969368588,38.8164122512189),
 .UNSPECIFIED.);
#1015=B_SPLINE_CURVE_WITH_KNOTS('',3,(#74144,#74145,#74146,#74147,#74148,
#74149,#74150,#74151,#74152,#74153,#74154,#74155,#74156,#74157,#74158,#74159,
#74160,#74161,#74162,#74163,#74164,#74165,#74166,#74167,#74168,#74169,#74170,
#74171,#74172,#74173,#74174,#74175,#74176,#74177,#74178,#74179,#74180,#74181,
#74182,#74183,#74184,#74185,#74186,#74187,#74188,#74189,#74190,#74191,#74192,
#74193,#74194,#74195,#74196,#74197,#74198,#74199,#74200,#74201,#74202,#74203,
#74204,#74205,#74206,#74207,#74208,#74209,#74210,#74211,#74212,#74213,#74214,
#74215,#74216,#74217,#74218,#74219,#74220,#74221,#74222,#74223,#74224,#74225,
#74226,#74227,#74228,#74229,#74230,#74231,#74232,#74233,#74234,#74235,#74236,
#74237,#74238,#74239,#74240,#74241,#74242,#74243,#74244,#74245,#74246,#74247,
#74248,#74249,#74250,#74251,#74252,#74253,#74254,#74255,#74256,#74257,#74258),
 .UNSPECIFIED.,.F.,.F.,(4,3,3,3,3,3,3,3,3,3,3,3,3,3,3,3,3,3,3,3,3,3,3,3,
3,3,3,3,3,3,3,3,3,3,3,3,3,3,4),(38.8164122514457,38.9226536638485,39.0919469197561,
39.2609110905423,39.4298459943078,39.5987355578191,39.7680308314881,39.92067042446,
40.089963680367,40.2589278511526,40.4278627549176,40.5967523184283,40.7660475920968,
40.9186871850715,41.0879804409785,41.2569446117641,41.4258795155291,41.5947690790398,
41.7640643527083,41.916703945683,42.0859972015901,42.2549613723759,42.4238962761409,
42.5927858396518,42.7620811133203,42.9147207062945,43.0840139622016,43.2529781329872,
43.4219130367523,43.590802600263,43.7600978739315,43.912737466906,44.0820307228131,
44.2509948935988,44.4199297973638,44.5888193608746,44.7581146345431,44.9107542275175,
45.0995975586252),.UNSPECIFIED.);
#1016=B_SPLINE_CURVE_WITH_KNOTS('',3,(#74260,#74261,#74262,#74263,#74264,
#74265,#74266,#74267,#74268,#74269),.UNSPECIFIED.,.F.,.F.,(4,1,1,1,1,1,
1,4),(45.0996018360204,45.908770988129,46.9067877487405,47.904804509352,
48.9028212699635,49.900838030575,50.8988547911865,51.3827816994375),
 .UNSPECIFIED.);
#1017=B_SPLINE_CURVE_WITH_KNOTS('',3,(#74271,#74272,#74273,#74274,#74275,
#74276,#74277,#74278,#74279,#74280,#74281,#74282,#74283,#74284,#74285,#74286,
#74287,#74288,#74289,#74290,#74291,#74292,#74293,#74294,#74295,#74296,#74297,
#74298,#74299,#74300,#74301,#74302,#74303,#74304,#74305,#74306,#74307,#74308,
#74309,#74310,#74311,#74312,#74313,#74314,#74315,#74316,#74317,#74318,#74319,
#74320,#74321,#74322,#74323,#74324,#74325,#74326,#74327,#74328,#74329,#74330,
#74331,#74332,#74333,#74334,#74335,#74336,#74337,#74338,#74339,#74340,#74341,
#74342,#74343,#74344,#74345,#74346,#74347,#74348,#74349,#74350,#74351,#74352,
#74353,#74354,#74355,#74356,#74357,#74358,#74359,#74360,#74361,#74362,#74363,
#74364,#74365,#74366,#74367,#74368,#74369,#74370,#74371,#74372,#74373,#74374,
#74375,#74376,#74377,#74378,#74379,#74380,#74381,#74382,#74383,#74384,#74385),
 .UNSPECIFIED.,.F.,.F.,(4,3,3,3,3,3,3,3,3,3,3,3,3,3,3,3,3,3,3,3,3,3,3,3,
3,3,3,3,3,3,3,3,3,3,3,3,3,3,4),(51.3827828658048,51.558714250667,51.7353860088453,
51.896871551798,52.0661648077051,52.2351289784908,52.4040638822558,52.5729534457665,
52.742248719435,52.8948883124095,53.0641815683166,53.2331457391023,53.4020806428674,
53.5709702063782,53.7402654800468,53.8929050730211,54.0621983289282,54.2311624997139,
54.4000974034789,54.5689869669897,54.7382822406583,54.8909218336326,55.0602150895396,
55.2291792603252,55.3981141640902,55.567003727601,55.7362990012695,55.8889385942441,
56.0582318501512,56.2271960209369,56.3961309247019,56.5650204882127,56.7343157618812,
56.8869553548556,57.0539545270545,57.2206780393154,57.3872309280649,57.5539523877524,
57.6659681729844),.UNSPECIFIED.);
#1018=B_SPLINE_CURVE_WITH_KNOTS('',3,(#74387,#74388,#74389,#74390,#74391,
#74392,#74393,#74394,#74395,#74396,#74397),.UNSPECIFIED.,.F.,.F.,(4,1,1,
1,1,1,1,1,4),(57.6659681729844,57.8849721154671,58.8829888760786,59.8810056366901,
60.8790223973016,61.8770391579131,62.8750559185246,63.8730726791361,63.949153480164),
 .UNSPECIFIED.);
#1019=B_SPLINE_CURVE_WITH_KNOTS('',3,(#74399,#74400,#74401,#74402,#74403,
#74404,#74405,#74406,#74407,#74408),.UNSPECIFIED.,.F.,.F.,(4,1,1,1,1,1,
1,4),(63.949153480164,64.8710894397476,65.8691062003591,66.8671229609706,
67.8651397215821,68.8631564821936,69.8611732428051,70.2323312382351),
 .UNSPECIFIED.);
#1020=B_SPLINE_CURVE_WITH_KNOTS('',3,(#74410,#74411,#74412,#74413,#74414,
#74415,#74416,#74417,#74418,#74419,#74420,#74421,#74422,#74423,#74424,#74425,
#74426,#74427,#74428,#74429,#74430,#74431,#74432,#74433,#74434,#74435,#74436,
#74437,#74438,#74439,#74440,#74441,#74442,#74443,#74444,#74445,#74446,#74447,
#74448,#74449,#74450,#74451,#74452,#74453,#74454,#74455,#74456,#74457,#74458,
#74459,#74460,#74461,#74462,#74463,#74464,#74465,#74466,#74467,#74468,#74469,
#74470,#74471,#74472,#74473,#74474,#74475,#74476,#74477,#74478,#74479,#74480,
#74481,#74482,#74483,#74484,#74485,#74486,#74487,#74488,#74489,#74490,#74491,
#74492,#74493,#74494,#74495,#74496,#74497,#74498,#74499,#74500,#74501,#74502,
#74503,#74504,#74505,#74506,#74507,#74508,#74509,#74510,#74511,#74512,#74513,
#74514,#74515,#74516,#74517,#74518,#74519,#74520,#74521,#74522,#74523,#74524),
 .UNSPECIFIED.,.F.,.F.,(4,3,3,3,3,3,3,3,3,3,3,3,3,3,3,3,3,3,3,3,3,3,3,3,
3,3,3,3,3,3,3,3,3,3,3,3,3,3,4),(70.2323387873436,70.402412598027,70.5725181553533,
70.7430744181846,70.8591900034166,71.0284832593237,71.1974474301093,71.3663823338743,
71.5352718973851,71.7045671710536,71.8572067640281,72.0265000199352,72.1954641907208,
72.3643990944859,72.5332886579967,72.7025839316653,72.8552235246396,73.0245167805467,
73.1934809513323,73.3624158550973,73.531305418608,73.7006006922766,73.8532402852511,
74.0225335411582,74.1914977119439,74.3604326157089,74.5293221792196,74.6986174528881,
74.8512570458626,75.0205503017697,75.1895144725554,75.3584493763205,75.5273389398313,
75.6966342134998,75.8492738064741,76.0184566568934,76.1873006327343,76.3560790711469,
76.5155240945232),.UNSPECIFIED.);
#1021=B_SPLINE_CURVE_WITH_KNOTS('',3,(#74526,#74527,#74528,#74529,#74530,
#74531,#74532,#74533,#74534,#74535),.UNSPECIFIED.,.F.,.F.,(4,1,1,1,1,1,
1,4),(76.5155312281036,76.8472905670856,77.8453073276971,78.8433240883086,
79.8413408489201,80.8393576095316,81.8373743701431,82.7987045196599),
 .UNSPECIFIED.);
#1022=B_SPLINE_CURVE_WITH_KNOTS('',3,(#74537,#74538,#74539,#74540,#74541,
#74542,#74543,#74544,#74545,#74546,#74547,#74548,#74549,#74550,#74551,#74552,
#74553,#74554,#74555,#74556,#74557,#74558,#74559,#74560,#74561,#74562,#74563,
#74564,#74565,#74566,#74567,#74568,#74569,#74570,#74571,#74572,#74573,#74574,
#74575,#74576,#74577,#74578,#74579,#74580,#74581,#74582,#74583,#74584,#74585,
#74586,#74587,#74588,#74589,#74590,#74591,#74592,#74593,#74594,#74595,#74596,
#74597,#74598,#74599,#74600,#74601,#74602,#74603,#74604,#74605,#74606,#74607,
#74608,#74609,#74610,#74611,#74612,#74613,#74614,#74615,#74616,#74617,#74618,
#74619,#74620,#74621,#74622,#74623,#74624,#74625,#74626,#74627,#74628,#74629,
#74630,#74631,#74632,#74633,#74634,#74635,#74636,#74637,#74638,#74639,#74640,
#74641,#74642,#74643,#74644,#74645,#74646,#74647,#74648,#74649,#74650,#74651,
#74652,#74653,#74654),.UNSPECIFIED.,.F.,.F.,(4,3,3,3,3,3,3,3,3,3,3,3,3,
3,3,3,3,3,3,3,3,3,3,3,3,3,3,3,3,3,3,3,3,3,3,3,3,3,3,4),(82.7987094017028,
82.8353911307546,83.0046843866608,83.1736485574456,83.3425834612097,83.5114730247196,
83.6807682983872,83.8334078913661,84.0027011472735,84.1716653180594,84.3406002218248,
84.5094897853358,84.6787850590047,84.8314246519776,85.0007179078847,85.1696820786705,
85.3386169824355,85.5075065459464,85.676801819615,85.8294414125891,85.9987346684959,
86.1676988392813,86.336633743046,86.5055233065565,86.6748185802248,86.8274581732006,
86.9967514291082,87.1657155998943,87.3346505036598,87.5035400671711,87.6728353408401,
87.8254749338121,87.9947681897189,88.1637323605044,88.3326672642691,88.5015568277797,
88.670852101448,88.8234916944236,89.0397925300301,89.0818945515453),
 .UNSPECIFIED.);
#1023=B_SPLINE_CURVE_WITH_KNOTS('',3,(#74656,#74657,#74658,#74659,#74660,
#74661,#74662,#74663,#74664,#74665),.UNSPECIFIED.,.F.,.F.,(4,1,1,1,1,1,
1,4),(89.0818947088824,89.8215084550351,90.8195252156466,91.8175419762581,
92.8155587368696,93.8135754974811,94.8115922580926,95.365080016062),
 .UNSPECIFIED.);
#1024=B_SPLINE_CURVE_WITH_KNOTS('',3,(#74667,#74668,#74669,#74670,#74671,
#74672,#74673,#74674,#74675,#74676),.UNSPECIFIED.,.F.,.F.,(4,1,1,1,1,1,
1,4),(95.365080016062,95.8096090187041,96.8076257793156,97.8056425399271,
98.8036593005386,99.8016760611501,100.799692821762,101.64825793954),
 .UNSPECIFIED.);
#1025=B_SPLINE_CURVE_WITH_KNOTS('',3,(#74678,#74679,#74680,#74681,#74682,
#74683,#74684,#74685,#74686,#74687,#74688,#74689,#74690,#74691,#74692,#74693,
#74694,#74695,#74696,#74697,#74698,#74699,#74700,#74701,#74702,#74703,#74704,
#74705,#74706,#74707,#74708,#74709,#74710,#74711,#74712,#74713,#74714,#74715,
#74716,#74717,#74718,#74719,#74720,#74721,#74722,#74723,#74724,#74725,#74726,
#74727,#74728,#74729,#74730,#74731,#74732,#74733,#74734,#74735,#74736,#74737,
#74738,#74739,#74740,#74741,#74742,#74743,#74744,#74745,#74746,#74747,#74748,
#74749,#74750,#74751,#74752,#74753,#74754,#74755,#74756,#74757,#74758,#74759,
#74760,#74761,#74762,#74763,#74764,#74765,#74766,#74767,#74768,#74769,#74770,
#74771,#74772,#74773,#74774,#74775,#74776,#74777,#74778,#74779,#74780,#74781,
#74782,#74783,#74784,#74785,#74786,#74787,#74788,#74789,#74790,#74791,#74792),
 .UNSPECIFIED.,.F.,.F.,(4,3,3,3,3,3,3,3,3,3,3,3,3,3,3,3,3,3,3,3,3,3,3,3,
3,3,3,3,3,3,3,3,3,3,3,3,3,3,4),(101.648265323242,101.797709582373,101.967002845301,
102.135967023136,102.304901933891,102.473791504371,102.643086784828,102.795726342985,
102.965019586104,103.133983744144,103.302918635414,103.471808186543,103.641103448279,
103.793743103596,103.963036360376,104.132000531843,104.300935435991,104.469824999722,
104.639120273341,104.791759864208,104.961053164949,105.130017380809,105.298952329355,
105.467841937566,105.637137254857,105.789776624819,105.95906978473,106.128033859723,
106.296968669389,106.465858139561,106.635153323104,106.787793385431,106.957086676536,
107.126050881224,107.294985816453,107.463875410149,107.633170711279,107.785810146042,
107.931450630421),.UNSPECIFIED.);
#1026=B_SPLINE_CURVE_WITH_KNOTS('',3,(#74794,#74795,#74796,#74797,#74798,
#74799,#74800,#74801,#74802,#74803),.UNSPECIFIED.,.F.,.F.,(4,1,1,1,1,1,
1,4),(107.931458239655,108.783826906654,109.781843667265,110.779860427877,
111.777877188488,112.7758939491,113.773910709711,114.214635937601),
 .UNSPECIFIED.);
#1027=B_SPLINE_CURVE_WITH_KNOTS('',3,(#74805,#74806,#74807,#74808,#74809,
#74810,#74811,#74812,#74813,#74814),.UNSPECIFIED.,.F.,.F.,(4,1,1,1,1,1,
1,4),(114.214635937601,114.771927470323,115.769944230934,116.767960991546,
117.765977752157,118.763994512769,119.76201127338,120.49782124478),
 .UNSPECIFIED.);
#1028=B_SPLINE_CURVE_WITH_KNOTS('',3,(#74822,#74823,#74824,#74825,#74826,
#74827,#74828,#74829,#74830),.UNSPECIFIED.,.F.,.F.,(4,1,1,1,1,1,4),(-122.756061555215,
-121.758044794603,-120.760028033992,-119.76201127338,-118.763994512769,
-117.765977752157,-117.190265949363),.UNSPECIFIED.);
#1029=B_SPLINE_CURVE_WITH_KNOTS('',3,(#74832,#74833,#74834,#74835,#74836,
#74837,#74838,#74839,#74840,#74841),.UNSPECIFIED.,.F.,.F.,(4,1,1,1,1,1,
1,4),(-117.190265949363,-116.767960991546,-115.769944230934,-114.771927470323,
-113.773910709711,-112.7758939491,-111.777877188488,-110.907080642184),
 .UNSPECIFIED.);
#1030=B_SPLINE_CURVE_WITH_KNOTS('',3,(#74843,#74844,#74845,#74846,#74847,
#74848,#74849,#74850,#74851,#74852,#74853),.UNSPECIFIED.,.F.,.F.,(4,1,1,
1,1,1,1,1,4),(-110.907080642184,-110.779860427877,-109.781843667265,-108.783826906654,
-107.785810146042,-106.787793385431,-105.789776624819,-104.791759864208,
-104.623895335004),.UNSPECIFIED.);
#1031=B_SPLINE_CURVE_WITH_KNOTS('',3,(#74855,#74856,#74857,#74858,#74859,
#74860,#74861,#74862,#74863,#74864,#74865,#74866,#74867,#74868,#74869,#74870,
#74871,#74872,#74873,#74874,#74875,#74876,#74877,#74878,#74879,#74880,#74881,
#74882,#74883,#74884,#74885,#74886,#74887,#74888,#74889,#74890,#74891,#74892,
#74893,#74894,#74895,#74896,#74897,#74898,#74899,#74900,#74901,#74902,#74903,
#74904,#74905,#74906,#74907,#74908,#74909,#74910,#74911,#74912,#74913,#74914,
#74915,#74916,#74917,#74918,#74919,#74920,#74921,#74922,#74923,#74924,#74925,
#74926,#74927,#74928,#74929,#74930,#74931,#74932,#74933,#74934,#74935,#74936,
#74937,#74938,#74939,#74940,#74941,#74942,#74943,#74944,#74945,#74946,#74947,
#74948,#74949,#74950,#74951,#74952,#74953,#74954,#74955,#74956,#74957,#74958,
#74959,#74960,#74961,#74962,#74963,#74964,#74965,#74966,#74967,#74968,#74969),
 .UNSPECIFIED.,.F.,.F.,(4,3,3,3,3,3,3,3,3,3,3,3,3,3,3,3,3,3,3,3,3,3,3,3,
3,3,3,3,3,3,3,3,3,3,3,3,3,3,4),(-104.623895335004,-104.45732649546,-104.29085058873,
-104.124460630739,-103.957682801808,-103.793743103596,-103.624449859544,
-103.455485700924,-103.286550809622,-103.11766125876,-102.948365997786,
-102.795726342985,-102.626433080327,-102.457468902668,-102.288533991942,
-102.119644421409,-101.950349140766,-101.797709582373,-101.628416327047,
-101.459452156828,-101.290517253598,-101.121627690605,-100.952332417415,
-100.799692821762,-100.630399567375,-100.461435398152,-100.292500495991,
-100.123610934111,-99.9543156620825,-99.8016760611501,-99.6323828042209,
-99.4634186323931,-99.294483727571,-99.1255941629928,-98.9562988882624,
-98.8036593005386,-98.6226668537811,-98.4425781871584,-98.3407102215442),
 .UNSPECIFIED.);
#1032=B_SPLINE_CURVE_WITH_KNOTS('',3,(#74971,#74972,#74973,#74974,#74975,
#74976,#74977,#74978,#74979,#74980),.UNSPECIFIED.,.F.,.F.,(4,1,1,1,1,1,
1,4),(-98.3407100278245,-97.8056425399271,-96.8076257793156,-95.8096090187041,
-94.8115922580926,-93.8135754974811,-92.8155587368696,-92.0575247206449),
 .UNSPECIFIED.);
#1033=B_SPLINE_CURVE_WITH_KNOTS('',3,(#74982,#74983,#74984,#74985,#74986,
#74987,#74988,#74989,#74990,#74991,#74992),.UNSPECIFIED.,.F.,.F.,(4,1,1,
1,1,1,1,1,4),(-92.0575247206449,-91.8175419762581,-90.8195252156466,-89.8215084550351,
-88.8234916944236,-87.8254749338121,-86.8274581732006,-85.8294414125891,
-85.7743394134653),.UNSPECIFIED.);
#1034=B_SPLINE_CURVE_WITH_KNOTS('',3,(#74994,#74995,#74996,#74997,#74998,
#74999,#75000,#75001,#75002,#75003,#75004,#75005,#75006,#75007,#75008,#75009,
#75010,#75011,#75012,#75013,#75014,#75015,#75016,#75017,#75018,#75019,#75020,
#75021,#75022,#75023,#75024,#75025,#75026,#75027,#75028,#75029,#75030,#75031,
#75032,#75033,#75034,#75035,#75036,#75037,#75038,#75039,#75040,#75041,#75042,
#75043,#75044,#75045,#75046,#75047,#75048,#75049,#75050,#75051,#75052,#75053,
#75054,#75055,#75056,#75057,#75058,#75059,#75060,#75061,#75062,#75063,#75064,
#75065,#75066,#75067,#75068,#75069,#75070,#75071,#75072,#75073,#75074,#75075,
#75076,#75077,#75078,#75079,#75080,#75081,#75082,#75083,#75084,#75085,#75086,
#75087,#75088,#75089,#75090,#75091,#75092,#75093,#75094,#75095,#75096,#75097,
#75098,#75099,#75100,#75101,#75102,#75103,#75104,#75105,#75106,#75107,#75108),
 .UNSPECIFIED.,.F.,.F.,(4,3,3,3,3,3,3,3,3,3,3,3,3,3,3,3,3,3,3,3,3,3,3,3,
3,3,3,3,3,3,3,3,3,3,3,3,3,3,4),(-85.7743394134653,-85.6064724999714,-85.4389194739953,
-85.2713832903716,-85.1038697181618,-84.9359767817762,-84.8314246519776,
-84.6621313960704,-84.4931672252848,-84.3242323215197,-84.1553427580088,
-83.9860474843402,-83.8334078913661,-83.664114635459,-83.4951504646734,
-83.3262155609084,-83.1573259973976,-82.9880307237291,-82.8353911307546,
-82.6660978748475,-82.4971337040618,-82.3281988002967,-82.1593092367859,
-81.9900139631174,-81.8373743701431,-81.668081114236,-81.4991169434503,
-81.3301820396853,-81.1612924761746,-80.991997202506,-80.8393576095316,
-80.6700643536246,-80.5011001828388,-80.3321652790738,-80.1632757155631,
-79.9939804418945,-79.8413408489201,-79.6466720371967,-79.4911543477215),
 .UNSPECIFIED.);
#1035=B_SPLINE_CURVE_WITH_KNOTS('',3,(#75110,#75111,#75112,#75113,#75114,
#75115,#75116,#75117,#75118,#75119),.UNSPECIFIED.,.F.,.F.,(4,1,1,1,1,1,
1,4),(-79.4911541062857,-78.8433240883086,-77.8453073276971,-76.8472905670856,
-75.8492738064741,-74.8512570458626,-73.853240285251,-73.2079687991061),
 .UNSPECIFIED.);
#1036=B_SPLINE_CURVE_WITH_KNOTS('',3,(#75121,#75122,#75123,#75124,#75125,
#75126,#75127,#75128,#75129,#75130,#75131,#75132,#75133,#75134,#75135,#75136,
#75137,#75138,#75139,#75140,#75141,#75142,#75143,#75144,#75145,#75146,#75147,
#75148,#75149,#75150,#75151,#75152,#75153,#75154,#75155,#75156,#75157,#75158,
#75159,#75160,#75161,#75162,#75163,#75164,#75165,#75166,#75167,#75168,#75169,
#75170,#75171,#75172,#75173,#75174,#75175,#75176,#75177,#75178,#75179,#75180,
#75181,#75182,#75183,#75184,#75185,#75186,#75187,#75188,#75189,#75190,#75191,
#75192,#75193,#75194,#75195,#75196,#75197,#75198,#75199,#75200,#75201,#75202,
#75203,#75204,#75205,#75206,#75207,#75208,#75209,#75210,#75211,#75212,#75213,
#75214,#75215,#75216,#75217,#75218,#75219,#75220,#75221,#75222,#75223,#75224,
#75225,#75226,#75227,#75228,#75229,#75230,#75231,#75232,#75233,#75234,#75235),
 .UNSPECIFIED.,.F.,.F.,(4,3,3,3,3,3,3,3,3,3,3,3,3,3,3,3,3,3,3,3,3,3,3,3,
3,3,3,3,3,3,3,3,3,3,3,3,3,3,4),(-73.2079685568002,-73.0137286976384,-72.8552235246396,
-72.6859302687325,-72.5169660979467,-72.3480311941816,-72.1791416306707,
-72.0098463570021,-71.8572067640281,-71.687913508121,-71.5189493373353,
-71.3500144335703,-71.1811248700595,-71.011829596391,-70.8591900034166,
-70.6898967475095,-70.5209325767238,-70.3519976729588,-70.183108109448,
-70.0138128357795,-69.8611732428051,-69.691879986898,-69.5229158161123,
-69.3539809123473,-69.1850913488366,-69.015796075168,-68.8631564821936,
-68.6938632262865,-68.5248990555009,-68.3559641517358,-68.1870745882251,
-68.0177793145566,-67.8651397215821,-67.6972941225137,-67.5297746092041,
-67.3622911014372,-67.1948402465308,-67.0270286612039,-66.9247834919265),
 .UNSPECIFIED.);
#1037=B_SPLINE_CURVE_WITH_KNOTS('',3,(#75237,#75238,#75239,#75240,#75241,
#75242,#75243,#75244,#75245,#75246,#75247),.UNSPECIFIED.,.F.,.F.,(4,1,1,
1,1,1,1,1,4),(-66.9247834919265,-66.8671229609706,-65.8691062003591,-64.8710894397476,
-63.8730726791361,-62.8750559185245,-61.8770391579131,-60.8790223973016,
-60.641598184747),.UNSPECIFIED.);
#1038=B_SPLINE_CURVE_WITH_KNOTS('',3,(#75249,#75250,#75251,#75252,#75253,
#75254,#75255,#75256,#75257,#75258),.UNSPECIFIED.,.F.,.F.,(4,1,1,1,1,1,
1,4),(-60.641598184747,-59.8810056366901,-58.8829888760786,-57.8849721154671,
-56.8869553548555,-55.8889385942441,-54.8909218336326,-54.3584128775674),
 .UNSPECIFIED.);
#1039=B_SPLINE_CURVE_WITH_KNOTS('',3,(#75260,#75261,#75262,#75263,#75264,
#75265,#75266,#75267,#75268,#75269,#75270,#75271,#75272,#75273,#75274,#75275,
#75276,#75277,#75278,#75279,#75280,#75281,#75282,#75283,#75284,#75285,#75286,
#75287,#75288,#75289,#75290,#75291,#75292,#75293,#75294,#75295,#75296,#75297,
#75298,#75299,#75300,#75301,#75302,#75303,#75304,#75305,#75306,#75307,#75308,
#75309,#75310,#75311,#75312,#75313,#75314,#75315,#75316,#75317,#75318,#75319,
#75320,#75321,#75322,#75323,#75324,#75325,#75326,#75327,#75328,#75329,#75330,
#75331,#75332,#75333,#75334,#75335,#75336,#75337,#75338,#75339,#75340,#75341,
#75342,#75343,#75344,#75345,#75346,#75347,#75348,#75349,#75350,#75351,#75352,
#75353,#75354,#75355,#75356,#75357,#75358,#75359,#75360,#75361,#75362,#75363,
#75364,#75365,#75366,#75367,#75368,#75369,#75370,#75371,#75372,#75373,#75374),
 .UNSPECIFIED.,.F.,.F.,(4,3,3,3,3,3,3,3,3,3,3,3,3,3,3,3,3,3,3,3,3,3,3,3,
3,3,3,3,3,3,3,3,3,3,3,3,3,3,4),(-54.3584126969109,-54.1786932265056,-53.998027905295,
-53.892905073021,-53.7236118171141,-53.5546476463285,-53.3857127425637,
-53.216823179053,-53.0475279053846,-52.8948883124096,-52.7255950565025,
-52.5566308857167,-52.3876959819517,-52.2188064184408,-52.0495111447722,
-51.896871551798,-51.7275782958909,-51.5586141251052,-51.3896792213402,
-51.2207896578294,-51.0514943841608,-50.8988547911866,-50.7295615352796,
-50.5605973644939,-50.3916624607289,-50.2227728972182,-50.0534776235497,
-49.9008380305751,-49.731544774668,-49.5625806038823,-49.3936457001172,
-49.2247561366064,-49.0554608629379,-48.9028212699636,-48.7360498525631,
-48.5695217660508,-48.4031605705744,-48.236550279102,-48.0752275703878),
 .UNSPECIFIED.);
#1040=B_SPLINE_CURVE_WITH_KNOTS('',3,(#75376,#75377,#75378,#75379,#75380,
#75381,#75382,#75383,#75384,#75385,#75386),.UNSPECIFIED.,.F.,.F.,(4,1,1,
1,1,1,1,1,4),(-48.0752275703878,-47.9048045093521,-46.9067877487405,-45.908770988129,
-44.9107542275176,-43.912737466906,-42.9147207062945,-41.916703945683,-41.7920422632082),
 .UNSPECIFIED.);
#1041=B_SPLINE_CURVE_WITH_KNOTS('',3,(#75388,#75389,#75390,#75391,#75392,
#75393,#75394,#75395,#75396,#75397,#75398,#75399,#75400,#75401,#75402,#75403,
#75404,#75405,#75406,#75407,#75408,#75409,#75410,#75411,#75412,#75413,#75414,
#75415,#75416,#75417,#75418,#75419,#75420,#75421,#75422,#75423,#75424,#75425,
#75426,#75427,#75428,#75429,#75430,#75431,#75432,#75433,#75434,#75435,#75436,
#75437,#75438,#75439,#75440,#75441,#75442,#75443,#75444,#75445,#75446,#75447,
#75448,#75449,#75450,#75451,#75452,#75453,#75454,#75455,#75456,#75457,#75458,
#75459,#75460,#75461,#75462,#75463,#75464,#75465,#75466,#75467,#75468,#75469,
#75470,#75471,#75472,#75473,#75474,#75475,#75476,#75477,#75478,#75479,#75480,
#75481,#75482,#75483,#75484,#75485,#75486,#75487,#75488,#75489,#75490,#75491,
#75492,#75493,#75494,#75495,#75496,#75497,#75498,#75499,#75500,#75501,#75502,
#75503,#75504,#75505),.UNSPECIFIED.,.F.,.F.,(4,3,3,3,3,3,3,3,3,3,3,3,3,
3,3,3,3,3,3,3,3,3,3,3,3,3,3,3,3,3,3,3,3,3,3,3,3,3,3,4),(-41.7920422632082,
-41.6252296124417,-41.4586871830981,-41.2921234036511,-41.1255384648325,
-40.9585984248305,-40.9186871850715,-40.7493939291644,-40.5804297583788,
-40.4114948546138,-40.242605291103,-40.0733100174345,-39.92067042446,-39.751377168553,
-39.5824129977674,-39.4134780940024,-39.2445885304916,-39.0752932568231,
-38.9226536638485,-38.7533604079413,-38.5843962371556,-38.4154613333905,
-38.2465717698797,-38.0772764962111,-37.924636903237,-37.7553436473299,
-37.5863794765442,-37.4174445727792,-37.2485550092685,-37.0792597356,-36.9266201426255,
-36.7573268867186,-36.588362715933,-36.4194278121681,-36.2505382486576,
-36.0812429749892,-35.928603382014,-35.7430372886009,-35.5587073803211,
-35.5088569562119),.UNSPECIFIED.);
#1042=B_SPLINE_CURVE_WITH_KNOTS('',3,(#75507,#75508,#75509,#75510,#75511,
#75512,#75513,#75514,#75515,#75516,#75517,#75518,#75519,#75520,#75521,#75522,
#75523,#75524,#75525,#75526,#75527,#75528,#75529,#75530,#75531,#75532,#75533,
#75534,#75535,#75536,#75537,#75538,#75539,#75540,#75541,#75542,#75543,#75544,
#75545,#75546,#75547,#75548,#75549,#75550,#75551,#75552,#75553,#75554,#75555,
#75556,#75557,#75558,#75559,#75560,#75561,#75562,#75563,#75564,#75565,#75566,
#75567,#75568,#75569,#75570,#75571,#75572,#75573,#75574,#75575,#75576,#75577,
#75578,#75579,#75580,#75581,#75582,#75583,#75584,#75585,#75586,#75587,#75588,
#75589,#75590,#75591,#75592,#75593,#75594,#75595,#75596,#75597,#75598,#75599,
#75600,#75601,#75602,#75603,#75604,#75605,#75606,#75607,#75608,#75609,#75610,
#75611,#75612,#75613,#75614,#75615,#75616,#75617,#75618,#75619,#75620,#75621,
#75622,#75623,#75624),.UNSPECIFIED.,.F.,.F.,(4,3,3,3,3,3,3,3,3,3,3,3,3,
3,3,3,3,3,3,3,3,3,3,3,3,3,3,3,3,3,3,3,3,3,3,3,3,3,3,4),(-35.5088569560286,
-35.3366913932997,-35.1643891329436,-34.9915938457824,-34.9305866214025,
-34.7612933654957,-34.5923291947103,-34.4233942909455,-34.254504727435,
-34.0852094537667,-33.932569860791,-33.763276604885,-33.5943124341005,-33.4253775303366,
-33.256487966827,-33.0871926931595,-32.9345531001795,-32.7652598442691,
-32.5962956734802,-32.4273607697119,-32.258471206198,-32.0891759325263,
-31.936536339568,-31.7672430836636,-31.5982789128805,-31.4293440091181,
-31.2604544456098,-31.0911591719436,-30.9385195789565,-30.7692263230558,
-30.6002621522766,-30.431327248518,-30.2624376850138,-30.0931424113516,
-29.940502818345,-29.7725436020734,-29.6049127376607,-29.4374658129547,
-29.2699561832517,-29.225671648849),.UNSPECIFIED.);
#1043=B_SPLINE_CURVE_WITH_KNOTS('',3,(#75626,#75627,#75628,#75629,#75630,
#75631,#75632,#75633,#75634,#75635,#75636),.UNSPECIFIED.,.F.,.F.,(4,1,1,
1,1,1,1,1,4),(-29.2256671317155,-28.9424860577335,-27.944469297122,-26.9464525365105,
-25.948435775899,-24.9504190152875,-23.952402254676,-22.9543854940645,-22.9424863416694),
 .UNSPECIFIED.);
#1044=B_SPLINE_CURVE_WITH_KNOTS('',3,(#75638,#75639,#75640,#75641,#75642,
#75643,#75644,#75645,#75646,#75647,#75648,#75649,#75650,#75651,#75652,#75653,
#75654,#75655,#75656,#75657,#75658,#75659,#75660,#75661,#75662,#75663,#75664,
#75665,#75666,#75667,#75668,#75669,#75670,#75671,#75672,#75673,#75674,#75675,
#75676,#75677,#75678,#75679,#75680,#75681,#75682,#75683,#75684,#75685,#75686,
#75687,#75688,#75689,#75690,#75691,#75692,#75693,#75694,#75695,#75696,#75697,
#75698,#75699,#75700,#75701,#75702,#75703,#75704,#75705,#75706,#75707,#75708,
#75709,#75710,#75711,#75712,#75713,#75714,#75715,#75716,#75717,#75718,#75719,
#75720,#75721,#75722,#75723,#75724,#75725,#75726,#75727,#75728,#75729,#75730,
#75731,#75732,#75733,#75734,#75735,#75736,#75737,#75738,#75739,#75740,#75741,
#75742,#75743,#75744,#75745,#75746,#75747,#75748,#75749,#75750,#75751,#75752),
 .UNSPECIFIED.,.F.,.F.,(4,3,3,3,3,3,3,3,3,3,3,3,3,3,3,3,3,3,3,3,3,3,3,3,
3,3,3,3,3,3,3,3,3,3,3,3,3,3,4),(-22.9424863416694,-22.7735464381667,-22.6049342401408,
-22.436350429138,-22.2678081433635,-22.0988663171801,-21.956368733453,-21.7870754780197,
-21.6181113077355,-21.4491764045062,-21.280286841551,-21.1109915684584,
-20.9583519728415,-20.7890587099447,-20.6200945321411,-20.451159621418,
-20.2822700509694,-20.1129747705427,-19.96033521223,-19.7910419690666,-19.6220778109816,
-19.4531429196686,-19.2842533684958,-19.1149581067184,-18.9623184516185,
-18.7930251948294,-18.6240610233531,-18.4551261191945,-18.2862365554524,
-18.1169412818215,-17.964301691007,-17.7950083904281,-17.6260441747308,
-17.4571092263467,-17.2882196182969,-17.1189243011628,-16.9662849303955,
-16.763195454698,-16.6593012290017),.UNSPECIFIED.);
#1045=B_SPLINE_CURVE_WITH_KNOTS('',3,(#75754,#75755,#75756,#75757,#75758,
#75759,#75760,#75761,#75762,#75763),.UNSPECIFIED.,.F.,.F.,(4,1,1,1,1,1,
1,4),(-16.6593010344898,-15.968268169784,-14.9702514091725,-13.972234648561,
-12.9742178879495,-11.976201127338,-10.9781843667265,-10.3761157273102),
 .UNSPECIFIED.);
#1046=B_SPLINE_CURVE_WITH_KNOTS('',3,(#75764,#75765,#75766,#75767,#75768,
#75769,#75770,#75771,#75772,#75773),.UNSPECIFIED.,.F.,.F.,(4,1,1,1,1,1,
1,4),(-10.3761157273102,-9.98016760611501,-8.98215084550351,-7.98413408489201,
-6.98611732428051,-5.98810056366901,-4.9900838030575,-4.09293928071616),
 .UNSPECIFIED.);
#1047=B_SPLINE_CURVE_WITH_KNOTS('',3,(#75776,#75777,#75778,#75779,#75780,
#75781,#75782,#75783,#75784,#75785,#75786,#75787,#75788,#75789,#75790,#75791,
#75792,#75793,#75794,#75795,#75796,#75797,#75798,#75799,#75800,#75801,#75802,
#75803,#75804,#75805,#75806,#75807,#75808,#75809,#75810,#75811,#75812,#75813,
#75814,#75815,#75816,#75817,#75818,#75819,#75820,#75821,#75822,#75823,#75824,
#75825,#75826,#75827,#75828,#75829,#75830,#75831,#75832,#75833,#75834,#75835,
#75836,#75837,#75838,#75839,#75840,#75841,#75842,#75843,#75844,#75845,#75846,
#75847,#75848,#75849,#75850,#75851,#75852,#75853,#75854,#75855,#75856,#75857,
#75858,#75859,#75860,#75861,#75862,#75863,#75864,#75865,#75866,#75867,#75868,
#75869,#75870,#75871,#75872,#75873,#75874,#75875,#75876,#75877,#75878,#75879,
#75880,#75881,#75882,#75883,#75884,#75885,#75886,#75887,#75888,#75889,#75890,
#75891,#75892,#75893,#75894,#75895,#75896,#75897,#75898,#75899,#75900,#75901,
#75902,#75903,#75904,#75905,#75906,#75907,#75908,#75909,#75910,#75911,#75912,
#75913,#75914,#75915,#75916,#75917,#75918,#75919,#75920,#75921,#75922,#75923,
#75924,#75925,#75926,#75927,#75928,#75929,#75930,#75931,#75932,#75933,#75934,
#75935,#75936,#75937,#75938,#75939,#75940,#75941,#75942,#75943,#75944,#75945,
#75946,#75947,#75948,#75949,#75950,#75951,#75952,#75953,#75954,#75955,#75956,
#75957,#75958,#75959,#75960,#75961,#75962,#75963,#75964,#75965,#75966,#75967,
#75968,#75969,#75970,#75971,#75972,#75973,#75974,#75975,#75976,#75977,#75978,
#75979,#75980,#75981,#75982,#75983,#75984,#75985,#75986,#75987,#75988,#75989,
#75990,#75991,#75992,#75993,#75994,#75995,#75996,#75997,#75998,#75999,#76000,
#76001,#76002,#76003,#76004,#76005,#76006,#76007),.UNSPECIFIED.,.F.,.F.,
(4,2,2,2,2,2,2,2,2,2,2,2,2,2,2,2,2,2,2,2,2,2,2,2,2,2,2,2,2,2,2,2,2,2,2,
2,2,2,2,2,2,2,2,2,2,2,2,2,2,2,2,2,2,2,2,2,2,2,2,2,2,2,2,2,2,2,2,2,2,2,2,
2,2,2,2,2,2,2,2,2,2,2,2,2,2,2,2,2,2,2,2,2,2,2,2,2,2,2,2,2,2,2,2,2,2,2,2,
2,2,2,2,2,2,2,2,4),(0.00386804990396825,0.0562394845893352,0.0855082425021677,
0.0967963778164743,0.101688678092589,0.105316915758188,0.109170828160612,
0.115206022997764,0.13352155193086,0.18214966217015,0.184505714254096,0.210496838182648,
0.216408804068253,0.21898183194266,0.219001669665326,0.219021656865823,
0.219041800143975,0.219062106303896,0.219082582367891,0.219103235589411,
0.219124073456259,0.219145103705878,0.21916633434941,0.219187773677002,
0.219209430278248,0.219231313055561,0.219253431238468,0.21927579440997,
0.219298412519007,0.219321295907952,0.219344455331709,0.219367901981367,
0.219391647508508,0.219415704054726,0.219440084280359,0.219456149678306,
0.219473316498225,0.219491677543212,0.219511335758724,0.219532405688436,
0.219555015155175,0.219579307277774,0.219605442856093,0.219633603231849,
0.21966399372401,0.219696847787709,0.21973243208813,0.219771052729119,0.219813062929726,
0.219858872626143,0.219896283448798,0.21995497467274,0.220103383909864,
0.222085813063994,0.224833395424335,0.231063205287695,0.267083001906452,
0.298908358386698,0.327015401127584,0.333646285187427,0.337599873377424,
0.341141196559091,0.345657839892338,0.355031731773855,0.409461104368223,
0.42212031792051,0.44147760840121,0.452386379069429,0.455728112289525,0.457846204907444,
0.459857139166811,0.462351221071398,0.468558193129114,0.505221941771184,
0.538022947485726,0.555995885137095,0.568369504724233,0.573366873604649,
0.576946354421215,0.58020234353761,0.584572579694303,0.593107307405052,
0.64484900429152,0.687001284439138,0.692128675899164,0.694610873875239,
0.696383997866516,0.698664122325341,0.702641545605574,0.719799480324097,
0.770150687164016,0.802462215093125,0.809319052133648,0.813315044379787,
0.816838441202234,0.821257209706951,0.829870588557781,0.889369746514473,
0.914109200745218,0.926855260915289,0.930387020161787,0.932551544688672,
0.934554760316714,0.936980728884274,0.943169252980154,0.986704068278608,
1.01565528028879,1.04026175474148,1.04663258402857,1.05051787081069,1.05405341606083,
1.05856448569977,1.0682373468359,1.11278921194253,1.14817633214325,1.16375694728592),
 .UNSPECIFIED.);
#1048=B_SPLINE_CURVE_WITH_KNOTS('',3,(#76011,#76012,#76013,#76014,#76015,
#76016,#76017,#76018,#76019,#76020,#76021,#76022,#76023,#76024,#76025,#76026,
#76027,#76028,#76029,#76030,#76031,#76032,#76033,#76034,#76035,#76036,#76037,
#76038,#76039,#76040,#76041,#76042,#76043,#76044,#76045,#76046,#76047,#76048,
#76049,#76050,#76051,#76052,#76053),.UNSPECIFIED.,.F.,.F.,(4,3,3,3,3,3,
3,3,3,3,3,3,3,3,4),(128.80529879753,129.037126539512,129.067505586393,129.244234518971,
129.420602827541,129.596971260776,129.773322085525,129.950145844604,130.065522347004,
130.24915598036,130.432352008113,130.615311891496,130.798119431239,130.981055100704,
131.063539107616),.UNSPECIFIED.);
#1049=B_SPLINE_CURVE_WITH_KNOTS('',3,(#76054,#76055,#76056,#76057,#76058,
#76059,#76060,#76061,#76062,#76063,#76064,#76065,#76066,#76067,#76068,#76069,
#76070,#76071,#76072,#76073,#76074,#76075,#76076,#76077,#76078,#76079,#76080,
#76081,#76082,#76083,#76084,#76085,#76086,#76087,#76088,#76089,#76090,#76091,
#76092,#76093,#76094,#76095,#76096,#76097,#76098,#76099,#76100,#76101,#76102,
#76103),.UNSPECIFIED.,.F.,.F.,(4,2,2,2,2,2,2,2,2,2,2,2,2,2,2,2,2,2,2,2,
2,2,2,2,4),(-2.98961655725948,-2.95583465484829,-2.9418819665473,-2.93716913675111,
-2.93276629062489,-2.92919655162135,-2.92508182892515,-2.91803211560185,
-2.88502465965471,-2.84900598810215,-2.82377017441525,-2.81864302010618,
-2.81604948517044,-2.81402857579406,-2.81164374604156,-2.80726775189915,
-2.78285881200516,-2.73132000540922,-2.7078524312586,-2.70166823698996,
-2.69772318235366,-2.69417904573976,-2.68964433807738,-2.68017874108153,
-2.65819190440258),.UNSPECIFIED.);
#1050=B_SPLINE_CURVE_WITH_KNOTS('',3,(#76107,#76108,#76109,#76110,#76111,
#76112,#76113,#76114,#76115,#76116,#76117,#76118,#76119,#76120,#76121,#76122,
#76123,#76124,#76125,#76126,#76127,#76128,#76129,#76130,#76131,#76132,#76133,
#76134,#76135,#76136,#76137,#76138,#76139,#76140,#76141,#76142,#76143,#76144,
#76145,#76146,#76147,#76148,#76149,#76150,#76151,#76152,#76153,#76154,#76155,
#76156,#76157,#76158,#76159,#76160,#76161),.UNSPECIFIED.,.F.,.F.,(4,3,3,
3,3,3,3,3,3,3,3,3,3,3,3,3,3,3,4),(-0.547315088709847,-0.531428325283962,
-0.490979859218829,-0.459260446609245,-0.418148761644263,-0.399517638250514,
-0.380002035550477,-0.330811395611051,-0.294813706749318,-0.256386932726606,
-0.252448329891692,-0.213875797295427,-0.196110964560955,-0.178602317878619,
-0.131364170579549,-0.0981581995066324,-0.0854921122832515,-0.0410303375732965,
0.),.UNSPECIFIED.);
#1051=B_SPLINE_CURVE_WITH_KNOTS('',3,(#76163,#76164,#76165,#76166),
 .UNSPECIFIED.,.F.,.F.,(4,4),(0.,0.0133475310981651),.UNSPECIFIED.);
#1052=B_SPLINE_CURVE_WITH_KNOTS('',3,(#76167,#76168,#76169,#76170,#76171,
#76172,#76173,#76174,#76175,#76176,#76177,#76178,#76179,#76180,#76181,#76182,
#76183,#76184,#76185,#76186,#76187,#76188,#76189,#76190,#76191,#76192,#76193,
#76194,#76195,#76196,#76197,#76198,#76199,#76200,#76201,#76202,#76203,#76204,
#76205,#76206,#76207,#76208,#76209,#76210,#76211,#76212,#76213,#76214,#76215,
#76216,#76217,#76218,#76219,#76220,#76221,#76222,#76223,#76224),
 .UNSPECIFIED.,.F.,.F.,(4,3,3,3,3,3,3,3,3,3,3,3,3,3,3,3,3,3,3,4),(-0.555272788399299,
-0.537779111114978,-0.501074110893508,-0.477787886406151,-0.446868439925717,
-0.42563948423308,-0.408907819583257,-0.360744333019942,-0.329827946927358,
-0.312213887820072,-0.282444121695023,-0.234073861148414,-0.224809052384305,
-0.20825707532324,-0.15619280649243,-0.130527661559902,-0.110867144085924,
-0.0896774338839242,-0.0374232998864532,0.),.UNSPECIFIED.);
#1053=B_SPLINE_CURVE_WITH_KNOTS('',3,(#76729,#76730,#76731,#76732),
 .UNSPECIFIED.,.F.,.F.,(4,4),(-0.00544371575786758,0.),.UNSPECIFIED.);
#1054=B_SPLINE_CURVE_WITH_KNOTS('',3,(#76733,#76734,#76735,#76736,#76737,
#76738,#76739,#76740,#76741,#76742,#76743,#76744,#76745,#76746,#76747,#76748,
#76749,#76750,#76751,#76752,#76753,#76754,#76755,#76756,#76757,#76758,#76759,
#76760,#76761,#76762,#76763,#76764,#76765,#76766,#76767,#76768,#76769,#76770,
#76771,#76772,#76773,#76774,#76775,#76776,#76777,#76778,#76779,#76780,#76781,
#76782,#76783,#76784,#76785,#76786,#76787,#76788,#76789,#76790),
 .UNSPECIFIED.,.F.,.F.,(4,3,3,3,3,3,3,3,3,3,3,3,3,3,3,3,3,3,3,4),(-0.555272788399386,
-0.537779111115071,-0.501074112362602,-0.477787892025313,-0.446868055693454,
-0.425638893303973,-0.408906546180235,-0.360743046457414,-0.329827221992677,
-0.312213870800153,-0.282444121695054,-0.247138606483173,-0.225449912105354,
-0.208551551306268,-0.156413663479703,-0.130587374300692,-0.110975709681529,
-0.089976587580161,-0.0377183992018807,-5.54359081993786E-15),
 .UNSPECIFIED.);
#1055=B_SPLINE_CURVE_WITH_KNOTS('',3,(#76796,#76797,#76798,#76799,#76800,
#76801,#76802,#76803,#76804,#76805,#76806,#76807,#76808,#76809,#76810,#76811,
#76812,#76813,#76814,#76815,#76816,#76817,#76818,#76819,#76820,#76821,#76822,
#76823,#76824,#76825,#76826,#76827,#76828,#76829,#76830,#76831,#76832,#76833,
#76834,#76835,#76836,#76837,#76838,#76839,#76840,#76841,#76842,#76843,#76844,
#76845,#76846,#76847,#76848,#76849,#76850),.UNSPECIFIED.,.F.,.F.,(4,3,3,
3,3,3,3,3,3,3,3,3,3,3,3,3,3,3,4),(-0.547315281725085,-0.531428325284014,
-0.496555825859975,-0.475791121788961,-0.449884625300703,-0.41656343962899,
-0.397878131514439,-0.372466266802526,-0.323055462904821,-0.303122396484449,
-0.284649768256134,-0.252448329891705,-0.202775577609412,-0.18183632959102,
-0.136377247193265,-0.103314858687064,-0.0827138692056586,-0.0383174249070739,
0.),.UNSPECIFIED.);
#1056=B_SPLINE_CURVE_WITH_KNOTS('',3,(#77355,#77356,#77357,#77358),
 .UNSPECIFIED.,.F.,.F.,(4,4),(0.,0.00545462077073238),.UNSPECIFIED.);
#1340=CONICAL_SURFACE('',#17159,0.320138837486628,1.0471975511966);
#1341=CONICAL_SURFACE('',#17164,0.1225,1.0267507402002);
#1342=CONICAL_SURFACE('',#17179,0.2775,0.785398163397449);
#1343=CONICAL_SURFACE('',#17180,0.49,0.785398163397449);
#1559=CYLINDRICAL_SURFACE('',#17122,0.237175);
#1560=CYLINDRICAL_SURFACE('',#17124,0.237175);
#1561=CYLINDRICAL_SURFACE('',#17125,0.237175);
#1562=CYLINDRICAL_SURFACE('',#17126,0.237175);
#1563=CYLINDRICAL_SURFACE('',#17127,0.237175);
#1564=CYLINDRICAL_SURFACE('',#17128,0.237175);
#1565=CYLINDRICAL_SURFACE('',#17129,0.237175);
#1566=CYLINDRICAL_SURFACE('',#17130,0.237175);
#1567=CYLINDRICAL_SURFACE('',#17131,0.237175);
#1568=CYLINDRICAL_SURFACE('',#17132,0.237175);
#1569=CYLINDRICAL_SURFACE('',#17133,0.237175);
#1570=CYLINDRICAL_SURFACE('',#17134,0.237175);
#1571=CYLINDRICAL_SURFACE('',#17135,0.237175);
#1572=CYLINDRICAL_SURFACE('',#17136,0.237175);
#1573=CYLINDRICAL_SURFACE('',#17137,0.237175);
#1574=CYLINDRICAL_SURFACE('',#17138,0.237175);
#1575=CYLINDRICAL_SURFACE('',#17139,0.237175);
#1576=CYLINDRICAL_SURFACE('',#17140,0.237175);
#1577=CYLINDRICAL_SURFACE('',#17141,0.237175);
#1578=CYLINDRICAL_SURFACE('',#17142,0.2942);
#1579=CYLINDRICAL_SURFACE('',#17147,0.237175);
#1580=CYLINDRICAL_SURFACE('',#17174,0.5);
#1746=FACE_BOUND('',#4210,.T.);
#1747=FACE_BOUND('',#4220,.T.);
#1748=FACE_BOUND('',#4224,.T.);
#2338=CIRCLE('',#17123,0.237175);
#2339=CIRCLE('',#17143,0.2942);
#2340=CIRCLE('',#17144,0.295065936436295);
#2341=CIRCLE('',#17145,0.2942);
#2342=CIRCLE('',#17146,0.2942);
#2343=CIRCLE('',#17148,0.237175);
#2344=CIRCLE('',#17150,0.2942);
#2345=CIRCLE('',#17152,0.2942);
#2346=CIRCLE('',#17153,0.2942);
#2347=CIRCLE('',#17155,0.3342);
#2348=CIRCLE('',#17156,0.04);
#2349=CIRCLE('',#17158,0.48);
#2350=CIRCLE('',#17160,0.308675134594813);
#2351=CIRCLE('',#17165,0.243346949651439);
#2352=CIRCLE('',#17171,0.44);
#2353=CIRCLE('',#17172,0.06);
#2354=CIRCLE('',#17173,0.5);
#2355=CIRCLE('',#17175,0.5);
#2356=CIRCLE('',#17178,0.255);
#3167=FACE_OUTER_BOUND('',#4183,.T.);
#3168=FACE_OUTER_BOUND('',#4184,.T.);
#3169=FACE_OUTER_BOUND('',#4185,.T.);
#3170=FACE_OUTER_BOUND('',#4186,.T.);
#3171=FACE_OUTER_BOUND('',#4187,.T.);
#3172=FACE_OUTER_BOUND('',#4188,.T.);
#3173=FACE_OUTER_BOUND('',#4189,.T.);
#3174=FACE_OUTER_BOUND('',#4190,.T.);
#3175=FACE_OUTER_BOUND('',#4191,.T.);
#3176=FACE_OUTER_BOUND('',#4192,.T.);
#3177=FACE_OUTER_BOUND('',#4193,.T.);
#3178=FACE_OUTER_BOUND('',#4194,.T.);
#3179=FACE_OUTER_BOUND('',#4195,.T.);
#3180=FACE_OUTER_BOUND('',#4196,.T.);
#3181=FACE_OUTER_BOUND('',#4197,.T.);
#3182=FACE_OUTER_BOUND('',#4198,.T.);
#3183=FACE_OUTER_BOUND('',#4199,.T.);
#3184=FACE_OUTER_BOUND('',#4200,.T.);
#3185=FACE_OUTER_BOUND('',#4201,.T.);
#3186=FACE_OUTER_BOUND('',#4202,.T.);
#3187=FACE_OUTER_BOUND('',#4203,.T.);
#3188=FACE_OUTER_BOUND('',#4204,.T.);
#3189=FACE_OUTER_BOUND('',#4205,.T.);
#3190=FACE_OUTER_BOUND('',#4206,.T.);
#3191=FACE_OUTER_BOUND('',#4207,.T.);
#3192=FACE_OUTER_BOUND('',#4208,.T.);
#3193=FACE_OUTER_BOUND('',#4209,.T.);
#3194=FACE_OUTER_BOUND('',#4211,.T.);
#3195=FACE_OUTER_BOUND('',#4212,.T.);
#3196=FACE_OUTER_BOUND('',#4213,.T.);
#3197=FACE_OUTER_BOUND('',#4214,.T.);
#3198=FACE_OUTER_BOUND('',#4215,.T.);
#3199=FACE_OUTER_BOUND('',#4216,.T.);
#3200=FACE_OUTER_BOUND('',#4217,.T.);
#3201=FACE_OUTER_BOUND('',#4218,.T.);
#3202=FACE_OUTER_BOUND('',#4219,.T.);
#3203=FACE_OUTER_BOUND('',#4221,.T.);
#3204=FACE_OUTER_BOUND('',#4222,.T.);
#3205=FACE_OUTER_BOUND('',#4223,.T.);
#3206=FACE_OUTER_BOUND('',#4225,.T.);
#3207=FACE_OUTER_BOUND('',#4226,.T.);
#3208=FACE_OUTER_BOUND('',#4227,.T.);
#4183=EDGE_LOOP('',(#13793,#13794,#13795,#13796));
#4184=EDGE_LOOP('',(#13797,#13798,#13799,#13800,#13801,#13802));
#4185=EDGE_LOOP('',(#13803,#13804,#13805,#13806));
#4186=EDGE_LOOP('',(#13807,#13808,#13809,#13810,#13811,#13812));
#4187=EDGE_LOOP('',(#13813,#13814,#13815,#13816));
#4188=EDGE_LOOP('',(#13817,#13818,#13819,#13820,#13821,#13822));
#4189=EDGE_LOOP('',(#13823,#13824,#13825,#13826));
#4190=EDGE_LOOP('',(#13827,#13828,#13829,#13830,#13831,#13832));
#4191=EDGE_LOOP('',(#13833,#13834,#13835,#13836));
#4192=EDGE_LOOP('',(#13837,#13838,#13839,#13840,#13841,#13842));
#4193=EDGE_LOOP('',(#13843,#13844,#13845,#13846));
#4194=EDGE_LOOP('',(#13847,#13848,#13849,#13850,#13851,#13852));
#4195=EDGE_LOOP('',(#13853,#13854,#13855,#13856,#13857));
#4196=EDGE_LOOP('',(#13858,#13859,#13860,#13861,#13862,#13863));
#4197=EDGE_LOOP('',(#13864,#13865,#13866,#13867,#13868,#13869));
#4198=EDGE_LOOP('',(#13870,#13871,#13872,#13873));
#4199=EDGE_LOOP('',(#13874,#13875,#13876,#13877,#13878,#13879));
#4200=EDGE_LOOP('',(#13880,#13881,#13882,#13883,#13884,#13885));
#4201=EDGE_LOOP('',(#13886,#13887,#13888,#13889,#13890));
#4202=EDGE_LOOP('',(#13891,#13892,#13893,#13894,#13895,#13896,#13897,#13898,
#13899,#13900,#13901,#13902,#13903,#13904,#13905,#13906,#13907,#13908,#13909,
#13910,#13911,#13912,#13913,#13914,#13915,#13916,#13917,#13918,#13919,#13920,
#13921,#13922,#13923,#13924,#13925,#13926,#13927,#13928,#13929,#13930,#13931,
#13932,#13933,#13934));
#4203=EDGE_LOOP('',(#13935,#13936,#13937,#13938,#13939));
#4204=EDGE_LOOP('',(#13940,#13941,#13942,#13943,#13944));
#4205=EDGE_LOOP('',(#13945,#13946,#13947,#13948,#13949,#13950,#13951,#13952,
#13953,#13954,#13955,#13956,#13957,#13958,#13959,#13960,#13961,#13962,#13963,
#13964,#13965,#13966,#13967,#13968,#13969,#13970,#13971,#13972,#13973,#13974,
#13975,#13976,#13977,#13978,#13979,#13980,#13981,#13982,#13983,#13984,#13985,
#13986,#13987,#13988,#13989,#13990,#13991,#13992,#13993,#13994,#13995,#13996,
#13997,#13998,#13999,#14000));
#4206=EDGE_LOOP('',(#14001,#14002,#14003,#14004,#14005));
#4207=EDGE_LOOP('',(#14006,#14007,#14008,#14009,#14010,#14011,#14012,#14013,
#14014,#14015,#14016,#14017,#14018,#14019,#14020,#14021,#14022,#14023,#14024,
#14025,#14026,#14027,#14028,#14029,#14030,#14031,#14032,#14033,#14034,#14035,
#14036,#14037,#14038,#14039,#14040,#14041,#14042,#14043,#14044,#14045,#14046,
#14047,#14048,#14049,#14050,#14051,#14052,#14053,#14054,#14055,#14056,#14057,
#14058,#14059,#14060));
#4208=EDGE_LOOP('',(#14061,#14062,#14063,#14064,#14065,#14066,#14067));
#4209=EDGE_LOOP('',(#14068));
#4210=EDGE_LOOP('',(#14069));
#4211=EDGE_LOOP('',(#14070,#14071,#14072,#14073,#14074,#14075,#14076,#14077,
#14078,#14079));
#4212=EDGE_LOOP('',(#14080,#14081,#14082,#14083));
#4213=EDGE_LOOP('',(#14084,#14085,#14086,#14087));
#4214=EDGE_LOOP('',(#14088,#14089,#14090,#14091));
#4215=EDGE_LOOP('',(#14092,#14093,#14094));
#4216=EDGE_LOOP('',(#14095,#14096,#14097,#14098));
#4217=EDGE_LOOP('',(#14099,#14100,#14101,#14102));
#4218=EDGE_LOOP('',(#14103,#14104,#14105,#14106,#14107));
#4219=EDGE_LOOP('',(#14108,#14109,#14110,#14111,#14112,#14113));
#4220=EDGE_LOOP('',(#14114));
#4221=EDGE_LOOP('',(#14115,#14116,#14117,#14118));
#4222=EDGE_LOOP('',(#14119,#14120,#14121,#14122));
#4223=EDGE_LOOP('',(#14123));
#4224=EDGE_LOOP('',(#14124));
#4225=EDGE_LOOP('',(#14125));
#4226=EDGE_LOOP('',(#14126,#14127,#14128,#14129,#14130,#14131,#14132));
#4227=EDGE_LOOP('',(#14133,#14134,#14135,#14136));
#5067=LINE('',#66634,#5927);
#5068=LINE('',#66766,#5928);
#5069=LINE('',#67166,#5929);
#5070=LINE('',#67596,#5930);
#5071=LINE('',#68112,#5931);
#5072=LINE('',#68548,#5932);
#5073=LINE('',#69040,#5933);
#5074=LINE('',#69468,#5934);
#5075=LINE('',#69976,#5935);
#5076=LINE('',#70404,#5936);
#5077=LINE('',#70862,#5937);
#5078=LINE('',#71292,#5938);
#5079=LINE('',#71565,#5939);
#5080=LINE('',#71886,#5940);
#5081=LINE('',#71994,#5941);
#5082=LINE('',#72355,#5942);
#5083=LINE('',#72777,#5943);
#5084=LINE('',#72905,#5944);
#5085=LINE('',#73170,#5945);
#5086=LINE('',#77396,#5946);
#5087=LINE('',#77400,#5947);
#5088=LINE('',#77402,#5948);
#5089=LINE('',#77403,#5949);
#5090=LINE('',#77406,#5950);
#5091=LINE('',#77407,#5951);
#5092=LINE('',#77410,#5952);
#5093=LINE('',#77411,#5953);
#5094=LINE('',#77415,#5954);
#5095=LINE('',#77419,#5955);
#5096=LINE('',#77420,#5956);
#5097=LINE('',#77423,#5957);
#5098=LINE('',#77424,#5958);
#5099=LINE('',#77426,#5959);
#5100=LINE('',#77436,#5960);
#5101=LINE('',#77443,#5961);
#5102=LINE('',#77445,#5962);
#5927=VECTOR('',#20658,0.237175);
#5928=VECTOR('',#20663,0.237175);
#5929=VECTOR('',#20666,0.237175);
#5930=VECTOR('',#20669,0.237175);
#5931=VECTOR('',#20672,0.237175);
#5932=VECTOR('',#20675,0.237175);
#5933=VECTOR('',#20678,0.237175);
#5934=VECTOR('',#20681,0.237175);
#5935=VECTOR('',#20684,0.237175);
#5936=VECTOR('',#20687,0.237175);
#5937=VECTOR('',#20690,0.237175);
#5938=VECTOR('',#20693,0.237175);
#5939=VECTOR('',#20696,0.237175);
#5940=VECTOR('',#20699,0.237175);
#5941=VECTOR('',#20702,0.237175);
#5942=VECTOR('',#20705,0.237175);
#5943=VECTOR('',#20708,0.237175);
#5944=VECTOR('',#20711,0.237175);
#5945=VECTOR('',#20714,0.237175);
#5946=VECTOR('',#20751,0.320138837486628);
#5947=VECTOR('',#20756,1.);
#5948=VECTOR('',#20757,1.);
#5949=VECTOR('',#20758,1.);
#5950=VECTOR('',#20761,1.);
#5951=VECTOR('',#20762,1.);
#5952=VECTOR('',#20765,1.);
#5953=VECTOR('',#20766,1.);
#5954=VECTOR('',#20769,0.1225);
#5955=VECTOR('',#20774,1.);
#5956=VECTOR('',#20775,1.);
#5957=VECTOR('',#20778,1.);
#5958=VECTOR('',#20779,1.);
#5959=VECTOR('',#20782,1.);
#5960=VECTOR('',#20795,0.5);
#5961=VECTOR('',#20806,0.2775);
#5962=VECTOR('',#20809,0.49);
#7290=VERTEX_POINT('',#66632);
#7291=VERTEX_POINT('',#66633);
#7292=VERTEX_POINT('',#66635);
#7293=VERTEX_POINT('',#66712);
#7294=VERTEX_POINT('',#66764);
#7295=VERTEX_POINT('',#66765);
#7296=VERTEX_POINT('',#66767);
#7297=VERTEX_POINT('',#66972);
#7298=VERTEX_POINT('',#67164);
#7299=VERTEX_POINT('',#67165);
#7300=VERTEX_POINT('',#67594);
#7301=VERTEX_POINT('',#67595);
#7302=VERTEX_POINT('',#67597);
#7303=VERTEX_POINT('',#67816);
#7304=VERTEX_POINT('',#68110);
#7305=VERTEX_POINT('',#68111);
#7306=VERTEX_POINT('',#68546);
#7307=VERTEX_POINT('',#68547);
#7308=VERTEX_POINT('',#68549);
#7309=VERTEX_POINT('',#68784);
#7310=VERTEX_POINT('',#69038);
#7311=VERTEX_POINT('',#69039);
#7312=VERTEX_POINT('',#69466);
#7313=VERTEX_POINT('',#69467);
#7314=VERTEX_POINT('',#69469);
#7315=VERTEX_POINT('',#69694);
#7316=VERTEX_POINT('',#69974);
#7317=VERTEX_POINT('',#69975);
#7318=VERTEX_POINT('',#70402);
#7319=VERTEX_POINT('',#70403);
#7320=VERTEX_POINT('',#70405);
#7321=VERTEX_POINT('',#70624);
#7322=VERTEX_POINT('',#70860);
#7323=VERTEX_POINT('',#70861);
#7324=VERTEX_POINT('',#71290);
#7325=VERTEX_POINT('',#71291);
#7326=VERTEX_POINT('',#71293);
#7327=VERTEX_POINT('',#71353);
#7328=VERTEX_POINT('',#71563);
#7329=VERTEX_POINT('',#71564);
#7330=VERTEX_POINT('',#71566);
#7331=VERTEX_POINT('',#71884);
#7332=VERTEX_POINT('',#71885);
#7333=VERTEX_POINT('',#71887);
#7334=VERTEX_POINT('',#71925);
#7335=VERTEX_POINT('',#71992);
#7336=VERTEX_POINT('',#71993);
#7337=VERTEX_POINT('',#71995);
#7338=VERTEX_POINT('',#72174);
#7339=VERTEX_POINT('',#72353);
#7340=VERTEX_POINT('',#72354);
#7341=VERTEX_POINT('',#72775);
#7342=VERTEX_POINT('',#72776);
#7343=VERTEX_POINT('',#72778);
#7344=VERTEX_POINT('',#72838);
#7345=VERTEX_POINT('',#72903);
#7346=VERTEX_POINT('',#72904);
#7347=VERTEX_POINT('',#72906);
#7348=VERTEX_POINT('',#73073);
#7349=VERTEX_POINT('',#73168);
#7350=VERTEX_POINT('',#73169);
#7351=VERTEX_POINT('',#73379);
#7352=VERTEX_POINT('',#73581);
#7353=VERTEX_POINT('',#73582);
#7354=VERTEX_POINT('',#73623);
#7355=VERTEX_POINT('',#73625);
#7356=VERTEX_POINT('',#73648);
#7357=VERTEX_POINT('',#73767);
#7358=VERTEX_POINT('',#73778);
#7359=VERTEX_POINT('',#73897);
#7360=VERTEX_POINT('',#74013);
#7361=VERTEX_POINT('',#74024);
#7362=VERTEX_POINT('',#74143);
#7363=VERTEX_POINT('',#74259);
#7364=VERTEX_POINT('',#74270);
#7365=VERTEX_POINT('',#74386);
#7366=VERTEX_POINT('',#74398);
#7367=VERTEX_POINT('',#74409);
#7368=VERTEX_POINT('',#74525);
#7369=VERTEX_POINT('',#74536);
#7370=VERTEX_POINT('',#74655);
#7371=VERTEX_POINT('',#74666);
#7372=VERTEX_POINT('',#74677);
#7373=VERTEX_POINT('',#74793);
#7374=VERTEX_POINT('',#74804);
#7375=VERTEX_POINT('',#74815);
#7376=VERTEX_POINT('',#74817);
#7377=VERTEX_POINT('',#74819);
#7378=VERTEX_POINT('',#74821);
#7379=VERTEX_POINT('',#74831);
#7380=VERTEX_POINT('',#74842);
#7381=VERTEX_POINT('',#74854);
#7382=VERTEX_POINT('',#74970);
#7383=VERTEX_POINT('',#74981);
#7384=VERTEX_POINT('',#74993);
#7385=VERTEX_POINT('',#75109);
#7386=VERTEX_POINT('',#75120);
#7387=VERTEX_POINT('',#75236);
#7388=VERTEX_POINT('',#75248);
#7389=VERTEX_POINT('',#75259);
#7390=VERTEX_POINT('',#75375);
#7391=VERTEX_POINT('',#75387);
#7392=VERTEX_POINT('',#75506);
#7393=VERTEX_POINT('',#75625);
#7394=VERTEX_POINT('',#75637);
#7395=VERTEX_POINT('',#75753);
#7396=VERTEX_POINT('',#75775);
#7397=VERTEX_POINT('',#76008);
#7398=VERTEX_POINT('',#76010);
#7399=VERTEX_POINT('',#76105);
#7400=VERTEX_POINT('',#76162);
#7401=VERTEX_POINT('',#76792);
#7402=VERTEX_POINT('',#76794);
#7403=VERTEX_POINT('',#77360);
#7404=VERTEX_POINT('',#77364);
#7405=VERTEX_POINT('',#77367);
#7406=VERTEX_POINT('',#77368);
#7407=VERTEX_POINT('',#77372);
#7408=VERTEX_POINT('',#77376);
#7409=VERTEX_POINT('',#77380);
#7410=VERTEX_POINT('',#77384);
#7411=VERTEX_POINT('',#77388);
#7412=VERTEX_POINT('',#77395);
#7413=VERTEX_POINT('',#77399);
#7414=VERTEX_POINT('',#77401);
#7415=VERTEX_POINT('',#77405);
#7416=VERTEX_POINT('',#77409);
#7417=VERTEX_POINT('',#77413);
#7418=VERTEX_POINT('',#77414);
#7419=VERTEX_POINT('',#77418);
#7420=VERTEX_POINT('',#77422);
#7421=VERTEX_POINT('',#77429);
#7422=VERTEX_POINT('',#77431);
#7423=VERTEX_POINT('',#77435);
#7424=VERTEX_POINT('',#77440);
#9518=EDGE_CURVE('',#7290,#7291,#5067,.T.);
#9519=EDGE_CURVE('',#7292,#7290,#947,.T.);
#9520=EDGE_CURVE('',#7293,#7292,#2338,.T.);
#9521=EDGE_CURVE('',#7293,#7291,#948,.T.);
#9522=EDGE_CURVE('',#7294,#7295,#5068,.T.);
#9523=EDGE_CURVE('',#7296,#7294,#949,.F.);
#9524=EDGE_CURVE('',#7290,#7296,#950,.T.);
#9525=EDGE_CURVE('',#7291,#7297,#951,.T.);
#9526=EDGE_CURVE('',#7297,#7295,#952,.T.);
#9527=EDGE_CURVE('',#7298,#7299,#5069,.T.);
#9528=EDGE_CURVE('',#7294,#7298,#953,.F.);
#9529=EDGE_CURVE('',#7295,#7299,#954,.T.);
#9530=EDGE_CURVE('',#7300,#7301,#5070,.T.);
#9531=EDGE_CURVE('',#7302,#7300,#955,.F.);
#9532=EDGE_CURVE('',#7298,#7302,#956,.F.);
#9533=EDGE_CURVE('',#7299,#7303,#957,.T.);
#9534=EDGE_CURVE('',#7303,#7301,#958,.T.);
#9535=EDGE_CURVE('',#7304,#7305,#5071,.T.);
#9536=EDGE_CURVE('',#7300,#7304,#959,.F.);
#9537=EDGE_CURVE('',#7301,#7305,#960,.T.);
#9538=EDGE_CURVE('',#7306,#7307,#5072,.T.);
#9539=EDGE_CURVE('',#7308,#7306,#961,.F.);
#9540=EDGE_CURVE('',#7304,#7308,#962,.F.);
#9541=EDGE_CURVE('',#7305,#7309,#963,.T.);
#9542=EDGE_CURVE('',#7309,#7307,#964,.T.);
#9543=EDGE_CURVE('',#7310,#7311,#5073,.T.);
#9544=EDGE_CURVE('',#7306,#7310,#965,.F.);
#9545=EDGE_CURVE('',#7307,#7311,#966,.T.);
#9546=EDGE_CURVE('',#7312,#7313,#5074,.T.);
#9547=EDGE_CURVE('',#7314,#7312,#967,.F.);
#9548=EDGE_CURVE('',#7310,#7314,#968,.F.);
#9549=EDGE_CURVE('',#7311,#7315,#969,.T.);
#9550=EDGE_CURVE('',#7315,#7313,#970,.T.);
#9551=EDGE_CURVE('',#7316,#7317,#5075,.T.);
#9552=EDGE_CURVE('',#7312,#7316,#971,.F.);
#9553=EDGE_CURVE('',#7313,#7317,#972,.T.);
#9554=EDGE_CURVE('',#7318,#7319,#5076,.T.);
#9555=EDGE_CURVE('',#7320,#7318,#973,.F.);
#9556=EDGE_CURVE('',#7316,#7320,#974,.F.);
#9557=EDGE_CURVE('',#7317,#7321,#975,.T.);
#9558=EDGE_CURVE('',#7321,#7319,#976,.T.);
#9559=EDGE_CURVE('',#7322,#7323,#5077,.T.);
#9560=EDGE_CURVE('',#7318,#7322,#977,.F.);
#9561=EDGE_CURVE('',#7319,#7323,#978,.T.);
#9562=EDGE_CURVE('',#7324,#7325,#5078,.T.);
#9563=EDGE_CURVE('',#7326,#7324,#979,.T.);
#9564=EDGE_CURVE('',#7322,#7326,#980,.F.);
#9565=EDGE_CURVE('',#7323,#7327,#981,.T.);
#9566=EDGE_CURVE('',#7327,#7325,#982,.T.);
#9567=EDGE_CURVE('',#7328,#7329,#5079,.T.);
#9568=EDGE_CURVE('',#7330,#7328,#983,.T.);
#9569=EDGE_CURVE('',#7324,#7330,#984,.T.);
#9570=EDGE_CURVE('',#7325,#7329,#985,.T.);
#9571=EDGE_CURVE('',#7331,#7332,#5080,.T.);
#9572=EDGE_CURVE('',#7333,#7331,#986,.T.);
#9573=EDGE_CURVE('',#7328,#7333,#987,.T.);
#9574=EDGE_CURVE('',#7329,#7334,#988,.T.);
#9575=EDGE_CURVE('',#7334,#7332,#989,.T.);
#9576=EDGE_CURVE('',#7335,#7336,#5081,.T.);
#9577=EDGE_CURVE('',#7337,#7335,#990,.F.);
#9578=EDGE_CURVE('',#7331,#7337,#991,.T.);
#9579=EDGE_CURVE('',#7332,#7338,#992,.T.);
#9580=EDGE_CURVE('',#7338,#7336,#993,.T.);
#9581=EDGE_CURVE('',#7339,#7340,#5082,.T.);
#9582=EDGE_CURVE('',#7335,#7339,#994,.F.);
#9583=EDGE_CURVE('',#7336,#7340,#995,.T.);
#9584=EDGE_CURVE('',#7341,#7342,#5083,.T.);
#9585=EDGE_CURVE('',#7343,#7341,#996,.T.);
#9586=EDGE_CURVE('',#7339,#7343,#997,.F.);
#9587=EDGE_CURVE('',#7340,#7344,#998,.T.);
#9588=EDGE_CURVE('',#7344,#7342,#999,.T.);
#9589=EDGE_CURVE('',#7345,#7346,#5084,.T.);
#9590=EDGE_CURVE('',#7347,#7345,#1000,.F.);
#9591=EDGE_CURVE('',#7341,#7347,#1001,.T.);
#9592=EDGE_CURVE('',#7342,#7348,#1002,.T.);
#9593=EDGE_CURVE('',#7348,#7346,#1003,.T.);
#9594=EDGE_CURVE('',#7349,#7350,#5085,.T.);
#9595=EDGE_CURVE('',#7345,#7349,#1004,.F.);
#9596=EDGE_CURVE('',#7346,#7351,#1005,.T.);
#9597=EDGE_CURVE('',#7351,#7350,#1006,.F.);
#9598=EDGE_CURVE('',#7352,#7353,#1007,.T.);
#9599=EDGE_CURVE('',#7353,#7354,#2339,.T.);
#9600=EDGE_CURVE('',#7354,#7355,#1008,.T.);
#9601=EDGE_CURVE('',#7355,#7356,#1009,.T.);
#9602=EDGE_CURVE('',#7356,#7357,#1010,.T.);
#9603=EDGE_CURVE('',#7357,#7358,#1011,.T.);
#9604=EDGE_CURVE('',#7358,#7359,#1012,.T.);
#9605=EDGE_CURVE('',#7359,#7360,#1013,.T.);
#9606=EDGE_CURVE('',#7360,#7361,#1014,.T.);
#9607=EDGE_CURVE('',#7361,#7362,#1015,.T.);
#9608=EDGE_CURVE('',#7362,#7363,#1016,.T.);
#9609=EDGE_CURVE('',#7363,#7364,#1017,.T.);
#9610=EDGE_CURVE('',#7364,#7365,#1018,.T.);
#9611=EDGE_CURVE('',#7365,#7366,#1019,.T.);
#9612=EDGE_CURVE('',#7366,#7367,#1020,.T.);
#9613=EDGE_CURVE('',#7367,#7368,#1021,.T.);
#9614=EDGE_CURVE('',#7368,#7369,#1022,.T.);
#9615=EDGE_CURVE('',#7369,#7370,#1023,.T.);
#9616=EDGE_CURVE('',#7370,#7371,#1024,.T.);
#9617=EDGE_CURVE('',#7371,#7372,#1025,.T.);
#9618=EDGE_CURVE('',#7372,#7373,#1026,.T.);
#9619=EDGE_CURVE('',#7373,#7374,#1027,.T.);
#9620=EDGE_CURVE('',#7374,#7375,#2340,.T.);
#9621=EDGE_CURVE('',#7376,#7375,#2341,.T.);
#9622=EDGE_CURVE('',#7377,#7376,#2342,.T.);
#9623=EDGE_CURVE('',#7377,#7378,#1028,.T.);
#9624=EDGE_CURVE('',#7378,#7379,#1029,.T.);
#9625=EDGE_CURVE('',#7379,#7380,#1030,.T.);
#9626=EDGE_CURVE('',#7380,#7381,#1031,.T.);
#9627=EDGE_CURVE('',#7381,#7382,#1032,.T.);
#9628=EDGE_CURVE('',#7382,#7383,#1033,.T.);
#9629=EDGE_CURVE('',#7383,#7384,#1034,.T.);
#9630=EDGE_CURVE('',#7384,#7385,#1035,.T.);
#9631=EDGE_CURVE('',#7385,#7386,#1036,.T.);
#9632=EDGE_CURVE('',#7386,#7387,#1037,.T.);
#9633=EDGE_CURVE('',#7387,#7388,#1038,.T.);
#9634=EDGE_CURVE('',#7388,#7389,#1039,.T.);
#9635=EDGE_CURVE('',#7389,#7390,#1040,.T.);
#9636=EDGE_CURVE('',#7390,#7391,#1041,.T.);
#9637=EDGE_CURVE('',#7391,#7392,#1042,.T.);
#9638=EDGE_CURVE('',#7392,#7393,#1043,.T.);
#9639=EDGE_CURVE('',#7393,#7394,#1044,.T.);
#9640=EDGE_CURVE('',#7394,#7395,#1045,.T.);
#9641=EDGE_CURVE('',#7395,#7352,#1046,.T.);
#9642=EDGE_CURVE('',#7350,#7396,#1047,.F.);
#9643=EDGE_CURVE('',#7397,#7396,#2343,.T.);
#9644=EDGE_CURVE('',#7398,#7397,#1048,.T.);
#9645=EDGE_CURVE('',#7349,#7398,#1049,.F.);
#9646=EDGE_CURVE('',#7399,#7377,#2344,.T.);
#9647=EDGE_CURVE('',#7399,#7397,#1050,.T.);
#9648=EDGE_CURVE('',#7396,#7400,#1051,.T.);
#9649=EDGE_CURVE('',#7400,#7377,#1052,.T.);
#9650=EDGE_CURVE('',#7375,#7399,#1053,.T.);
#9651=EDGE_CURVE('',#7292,#7354,#1054,.T.);
#9652=EDGE_CURVE('',#7354,#7401,#2345,.T.);
#9653=EDGE_CURVE('',#7401,#7402,#2346,.T.);
#9654=EDGE_CURVE('',#7402,#7293,#1055,.T.);
#9655=EDGE_CURVE('',#7402,#7353,#1056,.T.);
#9656=EDGE_CURVE('',#7403,#7403,#2347,.T.);
#9657=EDGE_CURVE('',#7403,#7376,#2348,.T.);
#9658=EDGE_CURVE('',#7404,#7404,#2349,.T.);
#9659=EDGE_CURVE('',#7405,#7406,#273,.T.);
#9660=EDGE_CURVE('',#7407,#7405,#274,.T.);
#9661=EDGE_CURVE('',#7408,#7407,#275,.T.);
#9662=EDGE_CURVE('',#7409,#7408,#276,.T.);
#9663=EDGE_CURVE('',#7410,#7409,#277,.T.);
#9664=EDGE_CURVE('',#7411,#7410,#278,.T.);
#9665=EDGE_CURVE('',#7406,#7411,#279,.T.);
#9666=EDGE_CURVE('',#7406,#7412,#5086,.T.);
#9667=EDGE_CURVE('',#7412,#7412,#2350,.T.);
#9668=EDGE_CURVE('',#7410,#7413,#5087,.T.);
#9669=EDGE_CURVE('',#7413,#7414,#5088,.T.);
#9670=EDGE_CURVE('',#7411,#7414,#5089,.T.);
#9671=EDGE_CURVE('',#7409,#7415,#5090,.T.);
#9672=EDGE_CURVE('',#7415,#7413,#5091,.T.);
#9673=EDGE_CURVE('',#7408,#7416,#5092,.T.);
#9674=EDGE_CURVE('',#7416,#7415,#5093,.T.);
#9675=EDGE_CURVE('',#7417,#7418,#5094,.T.);
#9676=EDGE_CURVE('',#7418,#7418,#2351,.T.);
#9677=EDGE_CURVE('',#7407,#7419,#5095,.T.);
#9678=EDGE_CURVE('',#7419,#7416,#5096,.T.);
#9679=EDGE_CURVE('',#7405,#7420,#5097,.T.);
#9680=EDGE_CURVE('',#7420,#7419,#5098,.T.);
#9681=EDGE_CURVE('',#7414,#7420,#5099,.T.);
#9682=EDGE_CURVE('',#7421,#7421,#2352,.T.);
#9683=EDGE_CURVE('',#7421,#7422,#2353,.T.);
#9684=EDGE_CURVE('',#7422,#7422,#2354,.T.);
#9685=EDGE_CURVE('',#7422,#7423,#5100,.T.);
#9686=EDGE_CURVE('',#7423,#7423,#2355,.T.);
#9687=EDGE_CURVE('',#7424,#7424,#2356,.T.);
#9688=EDGE_CURVE('',#7401,#7424,#5101,.T.);
#9689=EDGE_CURVE('',#7423,#7404,#5102,.T.);
#13793=ORIENTED_EDGE('',*,*,#9518,.F.);
#13794=ORIENTED_EDGE('',*,*,#9519,.F.);
#13795=ORIENTED_EDGE('',*,*,#9520,.F.);
#13796=ORIENTED_EDGE('',*,*,#9521,.T.);
#13797=ORIENTED_EDGE('',*,*,#9522,.F.);
#13798=ORIENTED_EDGE('',*,*,#9523,.F.);
#13799=ORIENTED_EDGE('',*,*,#9524,.F.);
#13800=ORIENTED_EDGE('',*,*,#9518,.T.);
#13801=ORIENTED_EDGE('',*,*,#9525,.T.);
#13802=ORIENTED_EDGE('',*,*,#9526,.T.);
#13803=ORIENTED_EDGE('',*,*,#9527,.F.);
#13804=ORIENTED_EDGE('',*,*,#9528,.F.);
#13805=ORIENTED_EDGE('',*,*,#9522,.T.);
#13806=ORIENTED_EDGE('',*,*,#9529,.T.);
#13807=ORIENTED_EDGE('',*,*,#9530,.F.);
#13808=ORIENTED_EDGE('',*,*,#9531,.F.);
#13809=ORIENTED_EDGE('',*,*,#9532,.F.);
#13810=ORIENTED_EDGE('',*,*,#9527,.T.);
#13811=ORIENTED_EDGE('',*,*,#9533,.T.);
#13812=ORIENTED_EDGE('',*,*,#9534,.T.);
#13813=ORIENTED_EDGE('',*,*,#9535,.F.);
#13814=ORIENTED_EDGE('',*,*,#9536,.F.);
#13815=ORIENTED_EDGE('',*,*,#9530,.T.);
#13816=ORIENTED_EDGE('',*,*,#9537,.T.);
#13817=ORIENTED_EDGE('',*,*,#9538,.F.);
#13818=ORIENTED_EDGE('',*,*,#9539,.F.);
#13819=ORIENTED_EDGE('',*,*,#9540,.F.);
#13820=ORIENTED_EDGE('',*,*,#9535,.T.);
#13821=ORIENTED_EDGE('',*,*,#9541,.T.);
#13822=ORIENTED_EDGE('',*,*,#9542,.T.);
#13823=ORIENTED_EDGE('',*,*,#9543,.F.);
#13824=ORIENTED_EDGE('',*,*,#9544,.F.);
#13825=ORIENTED_EDGE('',*,*,#9538,.T.);
#13826=ORIENTED_EDGE('',*,*,#9545,.T.);
#13827=ORIENTED_EDGE('',*,*,#9546,.F.);
#13828=ORIENTED_EDGE('',*,*,#9547,.F.);
#13829=ORIENTED_EDGE('',*,*,#9548,.F.);
#13830=ORIENTED_EDGE('',*,*,#9543,.T.);
#13831=ORIENTED_EDGE('',*,*,#9549,.T.);
#13832=ORIENTED_EDGE('',*,*,#9550,.T.);
#13833=ORIENTED_EDGE('',*,*,#9551,.F.);
#13834=ORIENTED_EDGE('',*,*,#9552,.F.);
#13835=ORIENTED_EDGE('',*,*,#9546,.T.);
#13836=ORIENTED_EDGE('',*,*,#9553,.T.);
#13837=ORIENTED_EDGE('',*,*,#9554,.F.);
#13838=ORIENTED_EDGE('',*,*,#9555,.F.);
#13839=ORIENTED_EDGE('',*,*,#9556,.F.);
#13840=ORIENTED_EDGE('',*,*,#9551,.T.);
#13841=ORIENTED_EDGE('',*,*,#9557,.T.);
#13842=ORIENTED_EDGE('',*,*,#9558,.T.);
#13843=ORIENTED_EDGE('',*,*,#9559,.F.);
#13844=ORIENTED_EDGE('',*,*,#9560,.F.);
#13845=ORIENTED_EDGE('',*,*,#9554,.T.);
#13846=ORIENTED_EDGE('',*,*,#9561,.T.);
#13847=ORIENTED_EDGE('',*,*,#9562,.F.);
#13848=ORIENTED_EDGE('',*,*,#9563,.F.);
#13849=ORIENTED_EDGE('',*,*,#9564,.F.);
#13850=ORIENTED_EDGE('',*,*,#9559,.T.);
#13851=ORIENTED_EDGE('',*,*,#9565,.T.);
#13852=ORIENTED_EDGE('',*,*,#9566,.T.);
#13853=ORIENTED_EDGE('',*,*,#9567,.F.);
#13854=ORIENTED_EDGE('',*,*,#9568,.F.);
#13855=ORIENTED_EDGE('',*,*,#9569,.F.);
#13856=ORIENTED_EDGE('',*,*,#9562,.T.);
#13857=ORIENTED_EDGE('',*,*,#9570,.T.);
#13858=ORIENTED_EDGE('',*,*,#9571,.F.);
#13859=ORIENTED_EDGE('',*,*,#9572,.F.);
#13860=ORIENTED_EDGE('',*,*,#9573,.F.);
#13861=ORIENTED_EDGE('',*,*,#9567,.T.);
#13862=ORIENTED_EDGE('',*,*,#9574,.T.);
#13863=ORIENTED_EDGE('',*,*,#9575,.T.);
#13864=ORIENTED_EDGE('',*,*,#9576,.F.);
#13865=ORIENTED_EDGE('',*,*,#9577,.F.);
#13866=ORIENTED_EDGE('',*,*,#9578,.F.);
#13867=ORIENTED_EDGE('',*,*,#9571,.T.);
#13868=ORIENTED_EDGE('',*,*,#9579,.T.);
#13869=ORIENTED_EDGE('',*,*,#9580,.T.);
#13870=ORIENTED_EDGE('',*,*,#9581,.F.);
#13871=ORIENTED_EDGE('',*,*,#9582,.F.);
#13872=ORIENTED_EDGE('',*,*,#9576,.T.);
#13873=ORIENTED_EDGE('',*,*,#9583,.T.);
#13874=ORIENTED_EDGE('',*,*,#9584,.F.);
#13875=ORIENTED_EDGE('',*,*,#9585,.F.);
#13876=ORIENTED_EDGE('',*,*,#9586,.F.);
#13877=ORIENTED_EDGE('',*,*,#9581,.T.);
#13878=ORIENTED_EDGE('',*,*,#9587,.T.);
#13879=ORIENTED_EDGE('',*,*,#9588,.T.);
#13880=ORIENTED_EDGE('',*,*,#9589,.F.);
#13881=ORIENTED_EDGE('',*,*,#9590,.F.);
#13882=ORIENTED_EDGE('',*,*,#9591,.F.);
#13883=ORIENTED_EDGE('',*,*,#9584,.T.);
#13884=ORIENTED_EDGE('',*,*,#9592,.T.);
#13885=ORIENTED_EDGE('',*,*,#9593,.T.);
#13886=ORIENTED_EDGE('',*,*,#9594,.F.);
#13887=ORIENTED_EDGE('',*,*,#9595,.F.);
#13888=ORIENTED_EDGE('',*,*,#9589,.T.);
#13889=ORIENTED_EDGE('',*,*,#9596,.T.);
#13890=ORIENTED_EDGE('',*,*,#9597,.T.);
#13891=ORIENTED_EDGE('',*,*,#9598,.T.);
#13892=ORIENTED_EDGE('',*,*,#9599,.T.);
#13893=ORIENTED_EDGE('',*,*,#9600,.T.);
#13894=ORIENTED_EDGE('',*,*,#9601,.T.);
#13895=ORIENTED_EDGE('',*,*,#9602,.T.);
#13896=ORIENTED_EDGE('',*,*,#9603,.T.);
#13897=ORIENTED_EDGE('',*,*,#9604,.T.);
#13898=ORIENTED_EDGE('',*,*,#9605,.T.);
#13899=ORIENTED_EDGE('',*,*,#9606,.T.);
#13900=ORIENTED_EDGE('',*,*,#9607,.T.);
#13901=ORIENTED_EDGE('',*,*,#9608,.T.);
#13902=ORIENTED_EDGE('',*,*,#9609,.T.);
#13903=ORIENTED_EDGE('',*,*,#9610,.T.);
#13904=ORIENTED_EDGE('',*,*,#9611,.T.);
#13905=ORIENTED_EDGE('',*,*,#9612,.T.);
#13906=ORIENTED_EDGE('',*,*,#9613,.T.);
#13907=ORIENTED_EDGE('',*,*,#9614,.T.);
#13908=ORIENTED_EDGE('',*,*,#9615,.T.);
#13909=ORIENTED_EDGE('',*,*,#9616,.T.);
#13910=ORIENTED_EDGE('',*,*,#9617,.T.);
#13911=ORIENTED_EDGE('',*,*,#9618,.T.);
#13912=ORIENTED_EDGE('',*,*,#9619,.T.);
#13913=ORIENTED_EDGE('',*,*,#9620,.T.);
#13914=ORIENTED_EDGE('',*,*,#9621,.F.);
#13915=ORIENTED_EDGE('',*,*,#9622,.F.);
#13916=ORIENTED_EDGE('',*,*,#9623,.T.);
#13917=ORIENTED_EDGE('',*,*,#9624,.T.);
#13918=ORIENTED_EDGE('',*,*,#9625,.T.);
#13919=ORIENTED_EDGE('',*,*,#9626,.T.);
#13920=ORIENTED_EDGE('',*,*,#9627,.T.);
#13921=ORIENTED_EDGE('',*,*,#9628,.T.);
#13922=ORIENTED_EDGE('',*,*,#9629,.T.);
#13923=ORIENTED_EDGE('',*,*,#9630,.T.);
#13924=ORIENTED_EDGE('',*,*,#9631,.T.);
#13925=ORIENTED_EDGE('',*,*,#9632,.T.);
#13926=ORIENTED_EDGE('',*,*,#9633,.T.);
#13927=ORIENTED_EDGE('',*,*,#9634,.T.);
#13928=ORIENTED_EDGE('',*,*,#9635,.T.);
#13929=ORIENTED_EDGE('',*,*,#9636,.T.);
#13930=ORIENTED_EDGE('',*,*,#9637,.T.);
#13931=ORIENTED_EDGE('',*,*,#9638,.T.);
#13932=ORIENTED_EDGE('',*,*,#9639,.T.);
#13933=ORIENTED_EDGE('',*,*,#9640,.T.);
#13934=ORIENTED_EDGE('',*,*,#9641,.T.);
#13935=ORIENTED_EDGE('',*,*,#9594,.T.);
#13936=ORIENTED_EDGE('',*,*,#9642,.T.);
#13937=ORIENTED_EDGE('',*,*,#9643,.F.);
#13938=ORIENTED_EDGE('',*,*,#9644,.F.);
#13939=ORIENTED_EDGE('',*,*,#9645,.F.);
#13940=ORIENTED_EDGE('',*,*,#9646,.F.);
#13941=ORIENTED_EDGE('',*,*,#9647,.T.);
#13942=ORIENTED_EDGE('',*,*,#9643,.T.);
#13943=ORIENTED_EDGE('',*,*,#9648,.T.);
#13944=ORIENTED_EDGE('',*,*,#9649,.T.);
#13945=ORIENTED_EDGE('',*,*,#9647,.F.);
#13946=ORIENTED_EDGE('',*,*,#9650,.F.);
#13947=ORIENTED_EDGE('',*,*,#9620,.F.);
#13948=ORIENTED_EDGE('',*,*,#9619,.F.);
#13949=ORIENTED_EDGE('',*,*,#9618,.F.);
#13950=ORIENTED_EDGE('',*,*,#9617,.F.);
#13951=ORIENTED_EDGE('',*,*,#9616,.F.);
#13952=ORIENTED_EDGE('',*,*,#9615,.F.);
#13953=ORIENTED_EDGE('',*,*,#9614,.F.);
#13954=ORIENTED_EDGE('',*,*,#9613,.F.);
#13955=ORIENTED_EDGE('',*,*,#9612,.F.);
#13956=ORIENTED_EDGE('',*,*,#9611,.F.);
#13957=ORIENTED_EDGE('',*,*,#9610,.F.);
#13958=ORIENTED_EDGE('',*,*,#9609,.F.);
#13959=ORIENTED_EDGE('',*,*,#9608,.F.);
#13960=ORIENTED_EDGE('',*,*,#9607,.F.);
#13961=ORIENTED_EDGE('',*,*,#9606,.F.);
#13962=ORIENTED_EDGE('',*,*,#9605,.F.);
#13963=ORIENTED_EDGE('',*,*,#9604,.F.);
#13964=ORIENTED_EDGE('',*,*,#9603,.F.);
#13965=ORIENTED_EDGE('',*,*,#9602,.F.);
#13966=ORIENTED_EDGE('',*,*,#9601,.F.);
#13967=ORIENTED_EDGE('',*,*,#9600,.F.);
#13968=ORIENTED_EDGE('',*,*,#9651,.F.);
#13969=ORIENTED_EDGE('',*,*,#9519,.T.);
#13970=ORIENTED_EDGE('',*,*,#9524,.T.);
#13971=ORIENTED_EDGE('',*,*,#9523,.T.);
#13972=ORIENTED_EDGE('',*,*,#9528,.T.);
#13973=ORIENTED_EDGE('',*,*,#9532,.T.);
#13974=ORIENTED_EDGE('',*,*,#9531,.T.);
#13975=ORIENTED_EDGE('',*,*,#9536,.T.);
#13976=ORIENTED_EDGE('',*,*,#9540,.T.);
#13977=ORIENTED_EDGE('',*,*,#9539,.T.);
#13978=ORIENTED_EDGE('',*,*,#9544,.T.);
#13979=ORIENTED_EDGE('',*,*,#9548,.T.);
#13980=ORIENTED_EDGE('',*,*,#9547,.T.);
#13981=ORIENTED_EDGE('',*,*,#9552,.T.);
#13982=ORIENTED_EDGE('',*,*,#9556,.T.);
#13983=ORIENTED_EDGE('',*,*,#9555,.T.);
#13984=ORIENTED_EDGE('',*,*,#9560,.T.);
#13985=ORIENTED_EDGE('',*,*,#9564,.T.);
#13986=ORIENTED_EDGE('',*,*,#9563,.T.);
#13987=ORIENTED_EDGE('',*,*,#9569,.T.);
#13988=ORIENTED_EDGE('',*,*,#9568,.T.);
#13989=ORIENTED_EDGE('',*,*,#9573,.T.);
#13990=ORIENTED_EDGE('',*,*,#9572,.T.);
#13991=ORIENTED_EDGE('',*,*,#9578,.T.);
#13992=ORIENTED_EDGE('',*,*,#9577,.T.);
#13993=ORIENTED_EDGE('',*,*,#9582,.T.);
#13994=ORIENTED_EDGE('',*,*,#9586,.T.);
#13995=ORIENTED_EDGE('',*,*,#9585,.T.);
#13996=ORIENTED_EDGE('',*,*,#9591,.T.);
#13997=ORIENTED_EDGE('',*,*,#9590,.T.);
#13998=ORIENTED_EDGE('',*,*,#9595,.T.);
#13999=ORIENTED_EDGE('',*,*,#9645,.T.);
#14000=ORIENTED_EDGE('',*,*,#9644,.T.);
#14001=ORIENTED_EDGE('',*,*,#9652,.T.);
#14002=ORIENTED_EDGE('',*,*,#9653,.T.);
#14003=ORIENTED_EDGE('',*,*,#9654,.T.);
#14004=ORIENTED_EDGE('',*,*,#9520,.T.);
#14005=ORIENTED_EDGE('',*,*,#9651,.T.);
#14006=ORIENTED_EDGE('',*,*,#9649,.F.);
#14007=ORIENTED_EDGE('',*,*,#9648,.F.);
#14008=ORIENTED_EDGE('',*,*,#9642,.F.);
#14009=ORIENTED_EDGE('',*,*,#9597,.F.);
#14010=ORIENTED_EDGE('',*,*,#9596,.F.);
#14011=ORIENTED_EDGE('',*,*,#9593,.F.);
#14012=ORIENTED_EDGE('',*,*,#9592,.F.);
#14013=ORIENTED_EDGE('',*,*,#9588,.F.);
#14014=ORIENTED_EDGE('',*,*,#9587,.F.);
#14015=ORIENTED_EDGE('',*,*,#9583,.F.);
#14016=ORIENTED_EDGE('',*,*,#9580,.F.);
#14017=ORIENTED_EDGE('',*,*,#9579,.F.);
#14018=ORIENTED_EDGE('',*,*,#9575,.F.);
#14019=ORIENTED_EDGE('',*,*,#9574,.F.);
#14020=ORIENTED_EDGE('',*,*,#9570,.F.);
#14021=ORIENTED_EDGE('',*,*,#9566,.F.);
#14022=ORIENTED_EDGE('',*,*,#9565,.F.);
#14023=ORIENTED_EDGE('',*,*,#9561,.F.);
#14024=ORIENTED_EDGE('',*,*,#9558,.F.);
#14025=ORIENTED_EDGE('',*,*,#9557,.F.);
#14026=ORIENTED_EDGE('',*,*,#9553,.F.);
#14027=ORIENTED_EDGE('',*,*,#9550,.F.);
#14028=ORIENTED_EDGE('',*,*,#9549,.F.);
#14029=ORIENTED_EDGE('',*,*,#9545,.F.);
#14030=ORIENTED_EDGE('',*,*,#9542,.F.);
#14031=ORIENTED_EDGE('',*,*,#9541,.F.);
#14032=ORIENTED_EDGE('',*,*,#9537,.F.);
#14033=ORIENTED_EDGE('',*,*,#9534,.F.);
#14034=ORIENTED_EDGE('',*,*,#9533,.F.);
#14035=ORIENTED_EDGE('',*,*,#9529,.F.);
#14036=ORIENTED_EDGE('',*,*,#9526,.F.);
#14037=ORIENTED_EDGE('',*,*,#9525,.F.);
#14038=ORIENTED_EDGE('',*,*,#9521,.F.);
#14039=ORIENTED_EDGE('',*,*,#9654,.F.);
#14040=ORIENTED_EDGE('',*,*,#9655,.T.);
#14041=ORIENTED_EDGE('',*,*,#9598,.F.);
#14042=ORIENTED_EDGE('',*,*,#9641,.F.);
#14043=ORIENTED_EDGE('',*,*,#9640,.F.);
#14044=ORIENTED_EDGE('',*,*,#9639,.F.);
#14045=ORIENTED_EDGE('',*,*,#9638,.F.);
#14046=ORIENTED_EDGE('',*,*,#9637,.F.);
#14047=ORIENTED_EDGE('',*,*,#9636,.F.);
#14048=ORIENTED_EDGE('',*,*,#9635,.F.);
#14049=ORIENTED_EDGE('',*,*,#9634,.F.);
#14050=ORIENTED_EDGE('',*,*,#9633,.F.);
#14051=ORIENTED_EDGE('',*,*,#9632,.F.);
#14052=ORIENTED_EDGE('',*,*,#9631,.F.);
#14053=ORIENTED_EDGE('',*,*,#9630,.F.);
#14054=ORIENTED_EDGE('',*,*,#9629,.F.);
#14055=ORIENTED_EDGE('',*,*,#9628,.F.);
#14056=ORIENTED_EDGE('',*,*,#9627,.F.);
#14057=ORIENTED_EDGE('',*,*,#9626,.F.);
#14058=ORIENTED_EDGE('',*,*,#9625,.F.);
#14059=ORIENTED_EDGE('',*,*,#9624,.F.);
#14060=ORIENTED_EDGE('',*,*,#9623,.F.);
#14061=ORIENTED_EDGE('',*,*,#9656,.T.);
#14062=ORIENTED_EDGE('',*,*,#9657,.T.);
#14063=ORIENTED_EDGE('',*,*,#9621,.T.);
#14064=ORIENTED_EDGE('',*,*,#9650,.T.);
#14065=ORIENTED_EDGE('',*,*,#9646,.T.);
#14066=ORIENTED_EDGE('',*,*,#9622,.T.);
#14067=ORIENTED_EDGE('',*,*,#9657,.F.);
#14068=ORIENTED_EDGE('',*,*,#9658,.F.);
#14069=ORIENTED_EDGE('',*,*,#9656,.F.);
#14070=ORIENTED_EDGE('',*,*,#9659,.F.);
#14071=ORIENTED_EDGE('',*,*,#9660,.F.);
#14072=ORIENTED_EDGE('',*,*,#9661,.F.);
#14073=ORIENTED_EDGE('',*,*,#9662,.F.);
#14074=ORIENTED_EDGE('',*,*,#9663,.F.);
#14075=ORIENTED_EDGE('',*,*,#9664,.F.);
#14076=ORIENTED_EDGE('',*,*,#9665,.F.);
#14077=ORIENTED_EDGE('',*,*,#9666,.T.);
#14078=ORIENTED_EDGE('',*,*,#9667,.F.);
#14079=ORIENTED_EDGE('',*,*,#9666,.F.);
#14080=ORIENTED_EDGE('',*,*,#9664,.T.);
#14081=ORIENTED_EDGE('',*,*,#9668,.T.);
#14082=ORIENTED_EDGE('',*,*,#9669,.T.);
#14083=ORIENTED_EDGE('',*,*,#9670,.F.);
#14084=ORIENTED_EDGE('',*,*,#9663,.T.);
#14085=ORIENTED_EDGE('',*,*,#9671,.T.);
#14086=ORIENTED_EDGE('',*,*,#9672,.T.);
#14087=ORIENTED_EDGE('',*,*,#9668,.F.);
#14088=ORIENTED_EDGE('',*,*,#9662,.T.);
#14089=ORIENTED_EDGE('',*,*,#9673,.T.);
#14090=ORIENTED_EDGE('',*,*,#9674,.T.);
#14091=ORIENTED_EDGE('',*,*,#9671,.F.);
#14092=ORIENTED_EDGE('',*,*,#9675,.T.);
#14093=ORIENTED_EDGE('',*,*,#9676,.F.);
#14094=ORIENTED_EDGE('',*,*,#9675,.F.);
#14095=ORIENTED_EDGE('',*,*,#9661,.T.);
#14096=ORIENTED_EDGE('',*,*,#9677,.T.);
#14097=ORIENTED_EDGE('',*,*,#9678,.T.);
#14098=ORIENTED_EDGE('',*,*,#9673,.F.);
#14099=ORIENTED_EDGE('',*,*,#9660,.T.);
#14100=ORIENTED_EDGE('',*,*,#9679,.T.);
#14101=ORIENTED_EDGE('',*,*,#9680,.T.);
#14102=ORIENTED_EDGE('',*,*,#9677,.F.);
#14103=ORIENTED_EDGE('',*,*,#9659,.T.);
#14104=ORIENTED_EDGE('',*,*,#9665,.T.);
#14105=ORIENTED_EDGE('',*,*,#9670,.T.);
#14106=ORIENTED_EDGE('',*,*,#9681,.T.);
#14107=ORIENTED_EDGE('',*,*,#9679,.F.);
#14108=ORIENTED_EDGE('',*,*,#9674,.F.);
#14109=ORIENTED_EDGE('',*,*,#9678,.F.);
#14110=ORIENTED_EDGE('',*,*,#9680,.F.);
#14111=ORIENTED_EDGE('',*,*,#9681,.F.);
#14112=ORIENTED_EDGE('',*,*,#9669,.F.);
#14113=ORIENTED_EDGE('',*,*,#9672,.F.);
#14114=ORIENTED_EDGE('',*,*,#9676,.T.);
#14115=ORIENTED_EDGE('',*,*,#9682,.T.);
#14116=ORIENTED_EDGE('',*,*,#9683,.T.);
#14117=ORIENTED_EDGE('',*,*,#9684,.T.);
#14118=ORIENTED_EDGE('',*,*,#9683,.F.);
#14119=ORIENTED_EDGE('',*,*,#9684,.F.);
#14120=ORIENTED_EDGE('',*,*,#9685,.T.);
#14121=ORIENTED_EDGE('',*,*,#9686,.T.);
#14122=ORIENTED_EDGE('',*,*,#9685,.F.);
#14123=ORIENTED_EDGE('',*,*,#9682,.F.);
#14124=ORIENTED_EDGE('',*,*,#9667,.T.);
#14125=ORIENTED_EDGE('',*,*,#9687,.F.);
#14126=ORIENTED_EDGE('',*,*,#9655,.F.);
#14127=ORIENTED_EDGE('',*,*,#9653,.F.);
#14128=ORIENTED_EDGE('',*,*,#9688,.T.);
#14129=ORIENTED_EDGE('',*,*,#9687,.T.);
#14130=ORIENTED_EDGE('',*,*,#9688,.F.);
#14131=ORIENTED_EDGE('',*,*,#9652,.F.);
#14132=ORIENTED_EDGE('',*,*,#9599,.F.);
#14133=ORIENTED_EDGE('',*,*,#9686,.F.);
#14134=ORIENTED_EDGE('',*,*,#9689,.T.);
#14135=ORIENTED_EDGE('',*,*,#9658,.T.);
#14136=ORIENTED_EDGE('',*,*,#9689,.F.);
#14713=PLANE('',#17149);
#14714=PLANE('',#17151);
#14715=PLANE('',#17157);
#14716=PLANE('',#17161);
#14717=PLANE('',#17162);
#14718=PLANE('',#17163);
#14719=PLANE('',#17166);
#14720=PLANE('',#17167);
#14721=PLANE('',#17168);
#14722=PLANE('',#17169);
#14723=PLANE('',#17176);
#14724=PLANE('',#17177);
#15523=ADVANCED_FACE('',(#3167),#1559,.T.);
#15524=ADVANCED_FACE('',(#3168),#1560,.T.);
#15525=ADVANCED_FACE('',(#3169),#1561,.T.);
#15526=ADVANCED_FACE('',(#3170),#1562,.T.);
#15527=ADVANCED_FACE('',(#3171),#1563,.T.);
#15528=ADVANCED_FACE('',(#3172),#1564,.T.);
#15529=ADVANCED_FACE('',(#3173),#1565,.T.);
#15530=ADVANCED_FACE('',(#3174),#1566,.T.);
#15531=ADVANCED_FACE('',(#3175),#1567,.T.);
#15532=ADVANCED_FACE('',(#3176),#1568,.T.);
#15533=ADVANCED_FACE('',(#3177),#1569,.T.);
#15534=ADVANCED_FACE('',(#3178),#1570,.T.);
#15535=ADVANCED_FACE('',(#3179),#1571,.T.);
#15536=ADVANCED_FACE('',(#3180),#1572,.T.);
#15537=ADVANCED_FACE('',(#3181),#1573,.T.);
#15538=ADVANCED_FACE('',(#3182),#1574,.T.);
#15539=ADVANCED_FACE('',(#3183),#1575,.T.);
#15540=ADVANCED_FACE('',(#3184),#1576,.T.);
#15541=ADVANCED_FACE('',(#3185),#1577,.T.);
#15542=ADVANCED_FACE('',(#3186),#1578,.T.);
#15543=ADVANCED_FACE('',(#3187),#1579,.T.);
#15544=ADVANCED_FACE('',(#3188),#14713,.F.);
#15545=ADVANCED_FACE('',(#3189),#256,.F.);
#15546=ADVANCED_FACE('',(#3190),#14714,.T.);
#15547=ADVANCED_FACE('',(#3191),#257,.F.);
#15548=ADVANCED_FACE('',(#3192),#157,.F.);
#15549=ADVANCED_FACE('',(#3193,#1746),#14715,.T.);
#15550=ADVANCED_FACE('',(#3194),#1340,.F.);
#15551=ADVANCED_FACE('',(#3195),#14716,.F.);
#15552=ADVANCED_FACE('',(#3196),#14717,.F.);
#15553=ADVANCED_FACE('',(#3197),#14718,.F.);
#15554=ADVANCED_FACE('',(#3198),#1341,.F.);
#15555=ADVANCED_FACE('',(#3199),#14719,.F.);
#15556=ADVANCED_FACE('',(#3200),#14720,.F.);
#15557=ADVANCED_FACE('',(#3201),#14721,.F.);
#15558=ADVANCED_FACE('',(#3202,#1747),#14722,.F.);
#15559=ADVANCED_FACE('',(#3203),#158,.T.);
#15560=ADVANCED_FACE('',(#3204),#1580,.T.);
#15561=ADVANCED_FACE('',(#3205,#1748),#14723,.T.);
#15562=ADVANCED_FACE('',(#3206),#14724,.T.);
#15563=ADVANCED_FACE('',(#3207),#1342,.T.);
#15564=ADVANCED_FACE('',(#3208),#1343,.T.);
#15628=CLOSED_SHELL('',(#15523,#15524,#15525,#15526,#15527,#15528,#15529,
#15530,#15531,#15532,#15533,#15534,#15535,#15536,#15537,#15538,#15539,#15540,
#15541,#15542,#15543,#15544,#15545,#15546,#15547,#15548,#15549,#15550,#15551,
#15552,#15553,#15554,#15555,#15556,#15557,#15558,#15559,#15560,#15561,#15562,
#15563,#15564));
#17121=AXIS2_PLACEMENT_3D('',#66630,#20654,#20655);
#17122=AXIS2_PLACEMENT_3D('',#66631,#20656,#20657);
#17123=AXIS2_PLACEMENT_3D('',#66713,#20659,#20660);
#17124=AXIS2_PLACEMENT_3D('',#66763,#20661,#20662);
#17125=AXIS2_PLACEMENT_3D('',#67163,#20664,#20665);
#17126=AXIS2_PLACEMENT_3D('',#67593,#20667,#20668);
#17127=AXIS2_PLACEMENT_3D('',#68109,#20670,#20671);
#17128=AXIS2_PLACEMENT_3D('',#68545,#20673,#20674);
#17129=AXIS2_PLACEMENT_3D('',#69037,#20676,#20677);
#17130=AXIS2_PLACEMENT_3D('',#69465,#20679,#20680);
#17131=AXIS2_PLACEMENT_3D('',#69973,#20682,#20683);
#17132=AXIS2_PLACEMENT_3D('',#70401,#20685,#20686);
#17133=AXIS2_PLACEMENT_3D('',#70859,#20688,#20689);
#17134=AXIS2_PLACEMENT_3D('',#71289,#20691,#20692);
#17135=AXIS2_PLACEMENT_3D('',#71562,#20694,#20695);
#17136=AXIS2_PLACEMENT_3D('',#71883,#20697,#20698);
#17137=AXIS2_PLACEMENT_3D('',#71991,#20700,#20701);
#17138=AXIS2_PLACEMENT_3D('',#72352,#20703,#20704);
#17139=AXIS2_PLACEMENT_3D('',#72774,#20706,#20707);
#17140=AXIS2_PLACEMENT_3D('',#72902,#20709,#20710);
#17141=AXIS2_PLACEMENT_3D('',#73167,#20712,#20713);
#17142=AXIS2_PLACEMENT_3D('',#73580,#20715,#20716);
#17143=AXIS2_PLACEMENT_3D('',#73624,#20717,#20718);
#17144=AXIS2_PLACEMENT_3D('',#74816,#20719,#20720);
#17145=AXIS2_PLACEMENT_3D('',#74818,#20721,#20722);
#17146=AXIS2_PLACEMENT_3D('',#74820,#20723,#20724);
#17147=AXIS2_PLACEMENT_3D('',#75774,#20725,#20726);
#17148=AXIS2_PLACEMENT_3D('',#76009,#20727,#20728);
#17149=AXIS2_PLACEMENT_3D('',#76104,#20729,#20730);
#17150=AXIS2_PLACEMENT_3D('',#76106,#20731,#20732);
#17151=AXIS2_PLACEMENT_3D('',#76791,#20733,#20734);
#17152=AXIS2_PLACEMENT_3D('',#76793,#20735,#20736);
#17153=AXIS2_PLACEMENT_3D('',#76795,#20737,#20738);
#17154=AXIS2_PLACEMENT_3D('',#77359,#20739,#20740);
#17155=AXIS2_PLACEMENT_3D('',#77361,#20741,#20742);
#17156=AXIS2_PLACEMENT_3D('',#77362,#20743,#20744);
#17157=AXIS2_PLACEMENT_3D('',#77363,#20745,#20746);
#17158=AXIS2_PLACEMENT_3D('',#77365,#20747,#20748);
#17159=AXIS2_PLACEMENT_3D('',#77366,#20749,#20750);
#17160=AXIS2_PLACEMENT_3D('',#77397,#20752,#20753);
#17161=AXIS2_PLACEMENT_3D('',#77398,#20754,#20755);
#17162=AXIS2_PLACEMENT_3D('',#77404,#20759,#20760);
#17163=AXIS2_PLACEMENT_3D('',#77408,#20763,#20764);
#17164=AXIS2_PLACEMENT_3D('',#77412,#20767,#20768);
#17165=AXIS2_PLACEMENT_3D('',#77416,#20770,#20771);
#17166=AXIS2_PLACEMENT_3D('',#77417,#20772,#20773);
#17167=AXIS2_PLACEMENT_3D('',#77421,#20776,#20777);
#17168=AXIS2_PLACEMENT_3D('',#77425,#20780,#20781);
#17169=AXIS2_PLACEMENT_3D('',#77427,#20783,#20784);
#17170=AXIS2_PLACEMENT_3D('',#77428,#20785,#20786);
#17171=AXIS2_PLACEMENT_3D('',#77430,#20787,#20788);
#17172=AXIS2_PLACEMENT_3D('',#77432,#20789,#20790);
#17173=AXIS2_PLACEMENT_3D('',#77433,#20791,#20792);
#17174=AXIS2_PLACEMENT_3D('',#77434,#20793,#20794);
#17175=AXIS2_PLACEMENT_3D('',#77437,#20796,#20797);
#17176=AXIS2_PLACEMENT_3D('',#77438,#20798,#20799);
#17177=AXIS2_PLACEMENT_3D('',#77439,#20800,#20801);
#17178=AXIS2_PLACEMENT_3D('',#77441,#20802,#20803);
#17179=AXIS2_PLACEMENT_3D('',#77442,#20804,#20805);
#17180=AXIS2_PLACEMENT_3D('',#77444,#20807,#20808);
#20654=DIRECTION('axis',(0.,0.,1.));
#20655=DIRECTION('refdir',(1.,0.,0.));
#20656=DIRECTION('center_axis',(0.,0.,1.));
#20657=DIRECTION('ref_axis',(0.176828393097112,-0.984241697650883,0.));
#20658=DIRECTION('',(0.,0.,-1.));
#20659=DIRECTION('center_axis',(0.,0.,-1.));
#20660=DIRECTION('ref_axis',(1.,9.72557910080329E-14,0.));
#20661=DIRECTION('center_axis',(0.,0.,1.));
#20662=DIRECTION('ref_axis',(0.176828393097112,-0.984241697650883,0.));
#20663=DIRECTION('',(0.,0.,-1.));
#20664=DIRECTION('center_axis',(0.,0.,1.));
#20665=DIRECTION('ref_axis',(0.176828393097112,-0.984241697650883,0.));
#20666=DIRECTION('',(0.,0.,-1.));
#20667=DIRECTION('center_axis',(0.,0.,1.));
#20668=DIRECTION('ref_axis',(0.176828393097112,-0.984241697650883,0.));
#20669=DIRECTION('',(0.,0.,-1.));
#20670=DIRECTION('center_axis',(0.,0.,1.));
#20671=DIRECTION('ref_axis',(0.176828393097112,-0.984241697650883,0.));
#20672=DIRECTION('',(0.,0.,-1.));
#20673=DIRECTION('center_axis',(0.,0.,1.));
#20674=DIRECTION('ref_axis',(0.176828393097112,-0.984241697650883,0.));
#20675=DIRECTION('',(0.,0.,-1.));
#20676=DIRECTION('center_axis',(0.,0.,1.));
#20677=DIRECTION('ref_axis',(0.176828393097112,-0.984241697650883,0.));
#20678=DIRECTION('',(0.,0.,-1.));
#20679=DIRECTION('center_axis',(0.,0.,1.));
#20680=DIRECTION('ref_axis',(0.176828393097112,-0.984241697650883,0.));
#20681=DIRECTION('',(0.,0.,-1.));
#20682=DIRECTION('center_axis',(0.,0.,1.));
#20683=DIRECTION('ref_axis',(0.176828393097112,-0.984241697650883,0.));
#20684=DIRECTION('',(0.,0.,-1.));
#20685=DIRECTION('center_axis',(0.,0.,1.));
#20686=DIRECTION('ref_axis',(0.176828393097112,-0.984241697650883,0.));
#20687=DIRECTION('',(0.,0.,-1.));
#20688=DIRECTION('center_axis',(0.,0.,1.));
#20689=DIRECTION('ref_axis',(0.176828393097112,-0.984241697650883,0.));
#20690=DIRECTION('',(0.,0.,-1.));
#20691=DIRECTION('center_axis',(0.,0.,1.));
#20692=DIRECTION('ref_axis',(0.176828393097112,-0.984241697650883,0.));
#20693=DIRECTION('',(0.,0.,-1.));
#20694=DIRECTION('center_axis',(0.,0.,1.));
#20695=DIRECTION('ref_axis',(0.176828393097112,-0.984241697650883,0.));
#20696=DIRECTION('',(0.,0.,-1.));
#20697=DIRECTION('center_axis',(0.,0.,1.));
#20698=DIRECTION('ref_axis',(0.176828393097112,-0.984241697650883,0.));
#20699=DIRECTION('',(0.,0.,-1.));
#20700=DIRECTION('center_axis',(0.,0.,1.));
#20701=DIRECTION('ref_axis',(0.176828393097112,-0.984241697650883,0.));
#20702=DIRECTION('',(0.,0.,-1.));
#20703=DIRECTION('center_axis',(0.,0.,1.));
#20704=DIRECTION('ref_axis',(0.176828393097112,-0.984241697650883,0.));
#20705=DIRECTION('',(0.,0.,-1.));
#20706=DIRECTION('center_axis',(0.,0.,1.));
#20707=DIRECTION('ref_axis',(0.176828393097112,-0.984241697650883,0.));
#20708=DIRECTION('',(0.,0.,-1.));
#20709=DIRECTION('center_axis',(0.,0.,1.));
#20710=DIRECTION('ref_axis',(0.176828393097112,-0.984241697650883,0.));
#20711=DIRECTION('',(0.,0.,-1.));
#20712=DIRECTION('center_axis',(0.,0.,1.));
#20713=DIRECTION('ref_axis',(0.176828393097112,-0.984241697650883,0.));
#20714=DIRECTION('',(0.,0.,-1.));
#20715=DIRECTION('center_axis',(0.,0.,1.));
#20716=DIRECTION('ref_axis',(1.,0.,0.));
#20717=DIRECTION('center_axis',(0.,0.,1.));
#20718=DIRECTION('ref_axis',(1.,0.,0.));
#20719=DIRECTION('center_axis',(-0.0068787995302466,0.0538364315100811,
0.998526074150937));
#20720=DIRECTION('ref_axis',(-0.982073479159668,-0.188467899125696,0.00339595794621756));
#20721=DIRECTION('center_axis',(0.,0.,1.));
#20722=DIRECTION('ref_axis',(1.,0.,0.));
#20723=DIRECTION('center_axis',(0.,0.,1.));
#20724=DIRECTION('ref_axis',(1.,0.,0.));
#20725=DIRECTION('center_axis',(0.,0.,1.));
#20726=DIRECTION('ref_axis',(-0.501423668270377,-0.86520188678613,0.));
#20727=DIRECTION('center_axis',(0.,0.,1.));
#20728=DIRECTION('ref_axis',(1.,9.72557910080329E-14,0.));
#20729=DIRECTION('center_axis',(0.,0.,1.));
#20730=DIRECTION('ref_axis',(1.,0.,0.));
#20731=DIRECTION('center_axis',(0.,0.,1.));
#20732=DIRECTION('ref_axis',(1.,0.,0.));
#20733=DIRECTION('center_axis',(0.,0.,1.));
#20734=DIRECTION('ref_axis',(1.,0.,0.));
#20735=DIRECTION('center_axis',(0.,0.,1.));
#20736=DIRECTION('ref_axis',(1.,0.,0.));
#20737=DIRECTION('center_axis',(0.,0.,1.));
#20738=DIRECTION('ref_axis',(1.,0.,0.));
#20739=DIRECTION('center_axis',(0.,0.,1.));
#20740=DIRECTION('ref_axis',(1.,0.,0.));
#20741=DIRECTION('center_axis',(0.,0.,-1.));
#20742=DIRECTION('ref_axis',(1.,0.,0.));
#20743=DIRECTION('center_axis',(-1.22464679914735E-16,1.,0.));
#20744=DIRECTION('ref_axis',(-1.,-1.22464679914735E-16,0.));
#20745=DIRECTION('center_axis',(0.,0.,-1.));
#20746=DIRECTION('ref_axis',(-1.,0.,0.));
#20747=DIRECTION('center_axis',(0.,0.,1.));
#20748=DIRECTION('ref_axis',(1.,0.,0.));
#20749=DIRECTION('center_axis',(0.,0.,1.));
#20750=DIRECTION('ref_axis',(1.,0.,0.));
#20751=DIRECTION('',(-0.86602540378444,-1.06057523872491E-16,0.499999999999998));
#20752=DIRECTION('center_axis',(0.,0.,-1.));
#20753=DIRECTION('ref_axis',(1.,0.,0.));
#20754=DIRECTION('center_axis',(-0.5,-0.866025403784439,0.));
#20755=DIRECTION('ref_axis',(-0.866025403784439,0.5,0.));
#20756=DIRECTION('',(0.,0.,-1.));
#20757=DIRECTION('',(-0.866025403784439,0.5,0.));
#20758=DIRECTION('',(0.,0.,-1.));
#20759=DIRECTION('center_axis',(0.5,-0.866025403784439,0.));
#20760=DIRECTION('ref_axis',(-0.866025403784439,-0.5,0.));
#20761=DIRECTION('',(0.,0.,-1.));
#20762=DIRECTION('',(-0.866025403784439,-0.5,0.));
#20763=DIRECTION('center_axis',(1.,-3.84592537276713E-16,0.));
#20764=DIRECTION('ref_axis',(-3.84592537276713E-16,-1.,0.));
#20765=DIRECTION('',(0.,0.,-1.));
#20766=DIRECTION('',(-3.84592537276713E-16,-1.,0.));
#20767=DIRECTION('center_axis',(0.,0.,1.));
#20768=DIRECTION('ref_axis',(1.,0.,0.));
#20769=DIRECTION('',(-0.855621686410732,-1.04783435954396E-16,0.517601709564076));
#20770=DIRECTION('center_axis',(0.,0.,-1.));
#20771=DIRECTION('ref_axis',(1.,0.,0.));
#20772=DIRECTION('center_axis',(0.5,0.866025403784439,0.));
#20773=DIRECTION('ref_axis',(0.866025403784439,-0.5,0.));
#20774=DIRECTION('',(0.,0.,-1.));
#20775=DIRECTION('',(0.866025403784439,-0.5,0.));
#20776=DIRECTION('center_axis',(-0.5,0.866025403784439,0.));
#20777=DIRECTION('ref_axis',(0.866025403784439,0.5,0.));
#20778=DIRECTION('',(0.,0.,-1.));
#20779=DIRECTION('',(0.866025403784439,0.5,0.));
#20780=DIRECTION('center_axis',(-1.,-1.92296268638356E-16,0.));
#20781=DIRECTION('ref_axis',(-1.92296268638356E-16,1.,0.));
#20782=DIRECTION('',(-1.92296268638356E-16,1.,0.));
#20783=DIRECTION('center_axis',(0.,0.,-1.));
#20784=DIRECTION('ref_axis',(-1.,0.,0.));
#20785=DIRECTION('center_axis',(0.,0.,1.));
#20786=DIRECTION('ref_axis',(1.,0.,0.));
#20787=DIRECTION('center_axis',(0.,0.,-1.));
#20788=DIRECTION('ref_axis',(-1.,1.22464679914735E-16,0.));
#20789=DIRECTION('center_axis',(1.22464679914735E-16,-1.,0.));
#20790=DIRECTION('ref_axis',(-1.,-1.22464679914735E-16,0.));
#20791=DIRECTION('center_axis',(0.,0.,1.));
#20792=DIRECTION('ref_axis',(-1.,1.22464679914735E-16,0.));
#20793=DIRECTION('center_axis',(0.,0.,1.));
#20794=DIRECTION('ref_axis',(1.,0.,0.));
#20795=DIRECTION('',(0.,0.,-1.));
#20796=DIRECTION('center_axis',(0.,0.,1.));
#20797=DIRECTION('ref_axis',(1.,0.,0.));
#20798=DIRECTION('center_axis',(0.,0.,1.));
#20799=DIRECTION('ref_axis',(1.,0.,0.));
#20800=DIRECTION('center_axis',(0.,0.,-1.));
#20801=DIRECTION('ref_axis',(-1.,0.,0.));
#20802=DIRECTION('center_axis',(0.,0.,1.));
#20803=DIRECTION('ref_axis',(1.,0.,0.));
#20804=DIRECTION('center_axis',(0.,0.,1.));
#20805=DIRECTION('ref_axis',(1.,0.,0.));
#20806=DIRECTION('',(0.707106781186548,8.65956056235494E-17,-0.707106781186547));
#20807=DIRECTION('center_axis',(0.,0.,1.));
#20808=DIRECTION('ref_axis',(1.,0.,0.));
#20809=DIRECTION('',(0.707106781186548,8.65956056235494E-17,-0.707106781186547));
#66630=CARTESIAN_POINT('',(0.,0.,0.));
#66631=CARTESIAN_POINT('Origin',(0.,0.,-2.1456589891905));
#66632=CARTESIAN_POINT('',(-0.0419392741328075,0.233437524640348,-1.89811014643447));
#66633=CARTESIAN_POINT('',(-0.0419392741328074,0.233437524640348,-1.91783866303197));
#66634=CARTESIAN_POINT('',(-0.0419392741328076,0.233437524640348,-2.1456589891905));
#66635=CARTESIAN_POINT('',(-0.137697683872004,-0.193109628142373,-1.9607937088529));
#66636=CARTESIAN_POINT('Ctrl Pts',(-0.137697683872004,-0.193109628142373,
-1.9607937088529));
#66637=CARTESIAN_POINT('Ctrl Pts',(-0.12637047603803,-0.201186544340074,
-1.95985501417045));
#66638=CARTESIAN_POINT('Ctrl Pts',(-0.114289949077831,-0.208291945347675,
-1.95891631948801));
#66639=CARTESIAN_POINT('Ctrl Pts',(-0.101649101270924,-0.214288219078449,
-1.95797762480556));
#66640=CARTESIAN_POINT('Ctrl Pts',(-0.0890324468673995,-0.220273016500722,
-1.95704072669716));
#66641=CARTESIAN_POINT('Ctrl Pts',(-0.075858331601906,-0.22515247421464,
-1.95610382858876));
#66642=CARTESIAN_POINT('Ctrl Pts',(-0.0623457780960344,-0.228833967274529,
-1.95516693048035));
#66643=CARTESIAN_POINT('Ctrl Pts',(-0.0488341882992543,-0.232515197772028,
-1.9542300991911));
#66644=CARTESIAN_POINT('Ctrl Pts',(-0.0349850177357809,-0.234998368896974,
-1.95329326790184));
#66645=CARTESIAN_POINT('Ctrl Pts',(-0.0210329134916387,-0.236240549387808,
-1.95235643661258));
#66646=CARTESIAN_POINT('Ctrl Pts',(-0.00708055823376012,-0.237482752226838,
-1.95141958846869));
#66647=CARTESIAN_POINT('Ctrl Pts',(0.00697388352572853,-0.237483875340244,
-1.9504827403248));
#66648=CARTESIAN_POINT('Ctrl Pts',(0.0208925910903226,-0.23625300053657,
-1.94954589218092));
#66649=CARTESIAN_POINT('Ctrl Pts',(0.0348412441386924,-0.235019477560191,
-1.94860702844968));
#66650=CARTESIAN_POINT('Ctrl Pts',(0.0486527402342993,-0.232548812747818,
-1.94766816471844));
#66651=CARTESIAN_POINT('Ctrl Pts',(0.0620972961073801,-0.228901521273128,
-1.9467293009872));
#66652=CARTESIAN_POINT('Ctrl Pts',(0.0652366861336961,-0.228049855320991,
-1.94651007028433));
#66653=CARTESIAN_POINT('Ctrl Pts',(0.068356140207546,-0.227134246202191,
-1.94629083958145));
#66654=CARTESIAN_POINT('Ctrl Pts',(0.0714528817785064,-0.226155845183243,
-1.94607160887858));
#66655=CARTESIAN_POINT('Ctrl Pts',(0.0848650768915338,-0.221918324852849,
-1.94512210602392));
#66656=CARTESIAN_POINT('Ctrl Pts',(0.0979424730591469,-0.216469828743788,
-1.94417260316927));
#66657=CARTESIAN_POINT('Ctrl Pts',(0.11045530094533,-0.209884747225892,
-1.94322310031462));
#66658=CARTESIAN_POINT('Ctrl Pts',(0.122943524780795,-0.203312613994437,
-1.9422754644733));
#66659=CARTESIAN_POINT('Ctrl Pts',(0.134868624317464,-0.195608655287244,
-1.94132782863197));
#66660=CARTESIAN_POINT('Ctrl Pts',(0.146021360452479,-0.186895005060615,
-1.94038019279065));
#66661=CARTESIAN_POINT('Ctrl Pts',(0.157172938080486,-0.178182259977326,
-1.9394326553864));
#66662=CARTESIAN_POINT('Ctrl Pts',(0.167551628355181,-0.168460504828884,
-1.93848511798215));
#66663=CARTESIAN_POINT('Ctrl Pts',(0.176978438280712,-0.157894309614755,
-1.9375375805779));
#66664=CARTESIAN_POINT('Ctrl Pts',(0.186403995536247,-0.14732951847643,
-1.93659016908599));
#66665=CARTESIAN_POINT('Ctrl Pts',(0.194877384600008,-0.135921143690584,
-1.93564275759408));
#66666=CARTESIAN_POINT('Ctrl Pts',(0.202259088856076,-0.123867839248571,
-1.93469534610217));
#66667=CARTESIAN_POINT('Ctrl Pts',(0.209658159563989,-0.111786177787108,
-1.93374570569734));
#66668=CARTESIAN_POINT('Ctrl Pts',(0.215960021336509,-0.0990572914205307,
-1.9327960652925));
#66669=CARTESIAN_POINT('Ctrl Pts',(0.221070752954074,-0.0859051966607303,
-1.93184642488766));
#66670=CARTESIAN_POINT('Ctrl Pts',(0.224046407741954,-0.0782475662721294,
-1.93129350952664));
#66671=CARTESIAN_POINT('Ctrl Pts',(0.226619178308375,-0.0704468605388091,
-1.93074059416561));
#66672=CARTESIAN_POINT('Ctrl Pts',(0.228778383837622,-0.0625494341592766,
-1.93018767880459));
#66673=CARTESIAN_POINT('Ctrl Pts',(0.232474781461577,-0.0490296336079843,
-1.92924112925243));
#66674=CARTESIAN_POINT('Ctrl Pts',(0.234981370144682,-0.0351342032452116,
-1.92829457970026));
#66675=CARTESIAN_POINT('Ctrl Pts',(0.236235029515445,-0.0210948205689673,
-1.9273480301481));
#66676=CARTESIAN_POINT('Ctrl Pts',(0.237486110216362,-0.00708431569924813,
-1.92640342756722));
#66677=CARTESIAN_POINT('Ctrl Pts',(0.237489230340424,0.00706873551438706,
-1.92545882498633));
#66678=CARTESIAN_POINT('Ctrl Pts',(0.236232450820277,0.0211236787621226,
-1.92451422240545));
#66679=CARTESIAN_POINT('Ctrl Pts',(0.234975900744799,0.0351760560611391,
-1.92356979227647));
#66680=CARTESIAN_POINT('Ctrl Pts',(0.232459931015672,0.0491295242772827,
-1.92262536214749));
#66681=CARTESIAN_POINT('Ctrl Pts',(0.228724667077634,0.0627455759016155,
-1.92168093201852));
#66682=CARTESIAN_POINT('Ctrl Pts',(0.224990083796739,0.0763591463457809,
-1.92073667398798));
#66683=CARTESIAN_POINT('Ctrl Pts',(0.220036886274952,0.0896346191670999,
-1.91979241595745));
#66684=CARTESIAN_POINT('Ctrl Pts',(0.213955295967831,0.102347994373695,
-1.91884815792692));
#66685=CARTESIAN_POINT('Ctrl Pts',(0.207859417454863,0.115091238629796,
-1.91790168143832));
#66686=CARTESIAN_POINT('Ctrl Pts',(0.200630255929949,0.127269011044877,
-1.91695520494971));
#66687=CARTESIAN_POINT('Ctrl Pts',(0.192404128186777,0.138681765498159,
-1.91600872846111));
#66688=CARTESIAN_POINT('Ctrl Pts',(0.187464621419128,0.145534731999475,
-1.91544040188427));
#66689=CARTESIAN_POINT('Ctrl Pts',(0.182166502845806,0.152112423109991,
-1.91487207530744));
#66690=CARTESIAN_POINT('Ctrl Pts',(0.176546005423108,0.158377677070173,
-1.9143037487306));
#66691=CARTESIAN_POINT('Ctrl Pts',(0.167169653179186,0.168829639523006,
-1.9133556422245));
#66692=CARTESIAN_POINT('Ctrl Pts',(0.156830382561657,0.17848120087317,-1.9124075357184));
#66693=CARTESIAN_POINT('Ctrl Pts',(0.145689671968511,0.187153680451942,
-1.9114594292123));
#66694=CARTESIAN_POINT('Ctrl Pts',(0.13457150480671,0.195808611109904,-1.91051324121702));
#66695=CARTESIAN_POINT('Ctrl Pts',(0.12265572453643,0.203487829808672,-1.90956705322175));
#66696=CARTESIAN_POINT('Ctrl Pts',(0.110138977720994,0.210050913379529,
-1.90862086522648));
#66697=CARTESIAN_POINT('Ctrl Pts',(0.097624262151212,0.216612931878512,
-1.90767483078071));
#66698=CARTESIAN_POINT('Ctrl Pts',(0.0845094877785817,0.222058744272142,
-1.90672879633494));
#66699=CARTESIAN_POINT('Ctrl Pts',(0.0710176130865216,0.226292905890779,
-1.90578276188917));
#66700=CARTESIAN_POINT('Ctrl Pts',(0.0575280064598183,0.230526355721359,
-1.90483688647749));
#66701=CARTESIAN_POINT('Ctrl Pts',(0.0436622270574184,0.233548326720256,
-1.90389101106581));
#66702=CARTESIAN_POINT('Ctrl Pts',(0.0296581196528709,0.235313358234623,
-1.90294513565413));
#66703=CARTESIAN_POINT('Ctrl Pts',(0.0156213338132154,0.237082508431184,
-1.90199705305227));
#66704=CARTESIAN_POINT('Ctrl Pts',(0.00144641050224148,0.237588802978478,
-1.90104897045041));
#66705=CARTESIAN_POINT('Ctrl Pts',(-0.0126244187202315,0.236838773592873,
-1.90010088784855));
#66706=CARTESIAN_POINT('Ctrl Pts',(-0.0209408662058052,0.236395474914494,
-1.89954053145124));
#66707=CARTESIAN_POINT('Ctrl Pts',(-0.0292209623871544,0.235514308440667,
-1.89898017505393));
#66708=CARTESIAN_POINT('Ctrl Pts',(-0.0374160476123589,0.234205081085082,
-1.89841981865661));
#66709=CARTESIAN_POINT('Ctrl Pts',(-0.0389256762846854,0.233963906393145,
-1.89831659458256));
#66710=CARTESIAN_POINT('Ctrl Pts',(-0.0404335213778545,0.233708047460805,
-1.89821337050852));
#66711=CARTESIAN_POINT('Ctrl Pts',(-0.0419392741328075,0.233437524640348,
-1.89811014643447));
#66712=CARTESIAN_POINT('',(0.137702479013104,-0.193106208855763,-1.9608));
#66713=CARTESIAN_POINT('Origin',(0.,0.,-1.9608));
#66714=CARTESIAN_POINT('Ctrl Pts',(0.137702479013104,-0.193106208855763,
-1.9608));
#66715=CARTESIAN_POINT('Ctrl Pts',(0.149477310386104,-0.184709671636007,
-1.95982953787546));
#66716=CARTESIAN_POINT('Ctrl Pts',(0.160496540954779,-0.175221999758771,
-1.95885907575091));
#66717=CARTESIAN_POINT('Ctrl Pts',(0.170563783261087,-0.164802841191118,
-1.95788861362637));
#66718=CARTESIAN_POINT('Ctrl Pts',(0.180623617019241,-0.154391350149052,
-1.95691886567112));
#66719=CARTESIAN_POINT('Ctrl Pts',(0.189732304539067,-0.143050282060555,
-1.95594911771588));
#66720=CARTESIAN_POINT('Ctrl Pts',(0.197730174513417,-0.130976176123346,
-1.95497936976064));
#66721=CARTESIAN_POINT('Ctrl Pts',(0.205737403722816,-0.118887940874727,
-1.95400848699086));
#66722=CARTESIAN_POINT('Ctrl Pts',(0.212630784608857,-0.106065601707679,
-1.95303760422109));
#66723=CARTESIAN_POINT('Ctrl Pts',(0.21829392961994,-0.0927347880575818,
-1.95206672145131));
#66724=CARTESIAN_POINT('Ctrl Pts',(0.223960335744276,-0.0793962978791635,
-1.95109527960021));
#66725=CARTESIAN_POINT('Ctrl Pts',(0.22839483161772,-0.0655494838953948,
-1.9501238377491));
#66726=CARTESIAN_POINT('Ctrl Pts',(0.231529867604011,-0.0514383226035734,
-1.94915239589799));
#66727=CARTESIAN_POINT('Ctrl Pts',(0.23467367162705,-0.0372876953594267,
-1.9481782371282));
#66728=CARTESIAN_POINT('Ctrl Pts',(0.23651064375352,-0.0228720170116576,
-1.94720407835841));
#66729=CARTESIAN_POINT('Ctrl Pts',(0.237024640569509,-0.00844395570185955,
-1.94622991958861));
#66730=CARTESIAN_POINT('Ctrl Pts',(0.23725571670898,-0.00195757173252825,
-1.94579196970108));
#66731=CARTESIAN_POINT('Ctrl Pts',(0.237220110839713,0.00453129736859094,
-1.94535401981354));
#66732=CARTESIAN_POINT('Ctrl Pts',(0.236919781413861,0.0109998999908311,
-1.94491606992601));
#66733=CARTESIAN_POINT('Ctrl Pts',(0.236276456812775,0.0248560554099354,
-1.94397795360293));
#66734=CARTESIAN_POINT('Ctrl Pts',(0.23441062882172,0.0387123928421089,
-1.94303983727984));
#66735=CARTESIAN_POINT('Ctrl Pts',(0.231329315697138,0.0523328608437726,
-1.94210172095676));
#66736=CARTESIAN_POINT('Ctrl Pts',(0.228255014392539,0.0659223341799007,
-1.94116573940626));
#66737=CARTESIAN_POINT('Ctrl Pts',(0.223970815010453,0.0792761621068477,
-1.94022975785576));
#66738=CARTESIAN_POINT('Ctrl Pts',(0.218535299951983,0.0921645447007527,
-1.93929377630527));
#66739=CARTESIAN_POINT('Ctrl Pts',(0.213101728896389,0.105048317786161,
-1.938358129507));
#66740=CARTESIAN_POINT('Ctrl Pts',(0.206517933627718,0.117466167693581,
-1.93742248270874));
#66741=CARTESIAN_POINT('Ctrl Pts',(0.198891613031466,0.129205676697045,
-1.93648683591048));
#66742=CARTESIAN_POINT('Ctrl Pts',(0.191267587961356,0.140941652102693,
-1.93555147074235));
#66743=CARTESIAN_POINT('Ctrl Pts',(0.18260213724279,0.151998982507965,-1.93461610557422));
#66744=CARTESIAN_POINT('Ctrl Pts',(0.173046444657011,0.162194046181011,
-1.9336807404061));
#66745=CARTESIAN_POINT('Ctrl Pts',(0.163468116365151,0.172413260114513,
-1.93274315952719));
#66746=CARTESIAN_POINT('Ctrl Pts',(0.152995954040751,0.181765534824852,
-1.93180557864829));
#66747=CARTESIAN_POINT('Ctrl Pts',(0.141817720437167,0.190104483889796,
-1.93086799776939));
#66748=CARTESIAN_POINT('Ctrl Pts',(0.134521763674017,0.195547259017382,
-1.93025604513027));
#66749=CARTESIAN_POINT('Ctrl Pts',(0.126925728673847,0.20055917307947,-1.92964409249114));
#66750=CARTESIAN_POINT('Ctrl Pts',(0.119087822964908,0.205109899923136,
-1.92903213985202));
#66751=CARTESIAN_POINT('Ctrl Pts',(0.106929239153337,0.212169233855818,
-1.92808284577682));
#66752=CARTESIAN_POINT('Ctrl Pts',(0.0941004426223774,0.218167136659545,
-1.92713355170162));
#66753=CARTESIAN_POINT('Ctrl Pts',(0.0808107590087802,0.222983411610426,
-1.92618425762642));
#66754=CARTESIAN_POINT('Ctrl Pts',(0.0675474741095219,0.227790119481285,
-1.92523684923517));
#66755=CARTESIAN_POINT('Ctrl Pts',(0.0538258694776703,0.231419511629482,
-1.92428944084392));
#66756=CARTESIAN_POINT('Ctrl Pts',(0.0398769046725999,0.233798659317654,
-1.92334203245268));
#66757=CARTESIAN_POINT('Ctrl Pts',(0.0259288860147947,0.236177645630117,
-1.92239468832339));
#66758=CARTESIAN_POINT('Ctrl Pts',(0.0117543479097061,0.237306364567924,
-1.9214473441941));
#66759=CARTESIAN_POINT('Ctrl Pts',(-0.0024045406954071,0.237162810763079,
-1.92050000006482));
#66760=CARTESIAN_POINT('Ctrl Pts',(-0.0156632124648629,0.237028384055392,
-1.91961288772054));
#66761=CARTESIAN_POINT('Ctrl Pts',(-0.0289075058911183,0.235778805895645,
-1.91872577537625));
#66762=CARTESIAN_POINT('Ctrl Pts',(-0.0419392741328073,0.233437524640348,
-1.91783866303197));
#66763=CARTESIAN_POINT('Origin',(0.,0.,-2.1456589891905));
#66764=CARTESIAN_POINT('',(-0.0419392500630468,0.233437528964709,-1.79799080372057));
#66765=CARTESIAN_POINT('',(-0.0419392741328097,0.233437524640348,-1.81760526556689));
#66766=CARTESIAN_POINT('',(-0.0419392741328076,0.233437524640348,-2.1456589891905));
#66767=CARTESIAN_POINT('',(-0.237174975484837,0.000107836760217876,-1.87594101081465));
#66768=CARTESIAN_POINT('Ctrl Pts',(-0.0419392500630493,0.233437528964708,
-1.79799080372057));
#66769=CARTESIAN_POINT('Ctrl Pts',(-0.0282675868112729,0.235893771996568,
-1.79898926705185));
#66770=CARTESIAN_POINT('Ctrl Pts',(-0.014401555316779,0.237145080218823,
-1.80001249030746));
#66771=CARTESIAN_POINT('Ctrl Pts',(0.00391717657812939,0.237183812422573,
-1.80134089095945));
#66772=CARTESIAN_POINT('Ctrl Pts',(0.00833543515462887,0.237069671857752,
-1.80165929127765));
#66773=CARTESIAN_POINT('Ctrl Pts',(0.017186016719489,0.236593265928485,
-1.80229025128174));
#66774=CARTESIAN_POINT('Ctrl Pts',(0.0216166837631987,0.236229671704668,
-1.80260265014077));
#66775=CARTESIAN_POINT('Ctrl Pts',(0.0272637718400154,0.235606018732023,
-1.80299429325227));
#66776=CARTESIAN_POINT('Ctrl Pts',(0.0284916570249254,0.235460686664155,
-1.80307905398002));
#66777=CARTESIAN_POINT('Ctrl Pts',(0.0304442378653119,0.235214081797173,
-1.80321314895662));
#66778=CARTESIAN_POINT('Ctrl Pts',(0.031169677629494,0.235119048841648,
-1.80326281685126));
#66779=CARTESIAN_POINT('Ctrl Pts',(0.0325548229261261,0.23493107062727,
-1.80335734618238));
#66780=CARTESIAN_POINT('Ctrl Pts',(0.0332145861601052,0.234838701492014,
-1.80340223711278));
#66781=CARTESIAN_POINT('Ctrl Pts',(0.0347872034170434,0.234611769703897,
-1.80350893326721));
#66782=CARTESIAN_POINT('Ctrl Pts',(0.0356996890314834,0.2344746559423,-1.80357059645435));
#66783=CARTESIAN_POINT('Ctrl Pts',(0.0388065076444369,0.233989255823198,
-1.80377978085021));
#66784=CARTESIAN_POINT('Ctrl Pts',(0.0409968157775473,0.233615450798555,
-1.80392595243139));
#66785=CARTESIAN_POINT('Ctrl Pts',(0.046352149475674,0.232623850032356,
-1.80428086177076));
#66786=CARTESIAN_POINT('Ctrl Pts',(0.0495105184518829,0.231972170865867,
-1.80448803692743));
#66787=CARTESIAN_POINT('Ctrl Pts',(0.0626142015597526,0.228988591234596,
-1.80534233722432));
#66788=CARTESIAN_POINT('Ctrl Pts',(0.0724175237677254,0.226079736434471,
-1.80596911731119));
#66789=CARTESIAN_POINT('Ctrl Pts',(0.0978266212221733,0.216717103424094,
-1.80762908603495));
#66790=CARTESIAN_POINT('Ctrl Pts',(0.112981015399952,0.209216532809259,
-1.80865976223155));
#66791=CARTESIAN_POINT('Ctrl Pts',(0.129881573591196,0.19847611239877,-1.80995397728956));
#66792=CARTESIAN_POINT('Ctrl Pts',(0.13251746723751,0.196725976137932,-1.8101602426783));
#66793=CARTESIAN_POINT('Ctrl Pts',(0.136355666874198,0.194065407908069,
-1.81046763045958));
#66794=CARTESIAN_POINT('Ctrl Pts',(0.137585635139072,0.193195350002201,
-1.81056722944285));
#66795=CARTESIAN_POINT('Ctrl Pts',(0.139758736546854,0.191626859475513,
-1.8107452077354));
#66796=CARTESIAN_POINT('Ctrl Pts',(0.140705140555662,0.190933027656012,
-1.81082340805523));
#66797=CARTESIAN_POINT('Ctrl Pts',(0.142690710160618,0.189454578399914,
-1.81098895762521));
#66798=CARTESIAN_POINT('Ctrl Pts',(0.143728638087296,0.188668371803563,
-1.81107636729729));
#66799=CARTESIAN_POINT('Ctrl Pts',(0.146474537996454,0.186552606848993,
-1.81130998054245));
#66800=CARTESIAN_POINT('Ctrl Pts',(0.148170838271243,0.185208173543935,
-1.8114567689564));
#66801=CARTESIAN_POINT('Ctrl Pts',(0.156680807594783,0.178271704161976,
-1.81220606159333));
#66802=CARTESIAN_POINT('Ctrl Pts',(0.163196550835474,0.172326804781988,
-1.81282275249359));
#66803=CARTESIAN_POINT('Ctrl Pts',(0.17716749081423,0.158075495315829,-1.81424668472668));
#66804=CARTESIAN_POINT('Ctrl Pts',(0.184398047034072,0.149577761665817,
-1.81505977316738));
#66805=CARTESIAN_POINT('Ctrl Pts',(0.19821885125347,0.130802849606491,-1.81676238936714));
#66806=CARTESIAN_POINT('Ctrl Pts',(0.204669421318344,0.120459891476853,
-1.81764961698169));
#66807=CARTESIAN_POINT('Ctrl Pts',(0.211255574220567,0.107830200586463,
-1.81864318672013));
#66808=CARTESIAN_POINT('Ctrl Pts',(0.212189139154548,0.105981317936876,
-1.81878648036838));
#66809=CARTESIAN_POINT('Ctrl Pts',(0.213464135592412,0.103371840901509,
-1.81898547749613));
#66810=CARTESIAN_POINT('Ctrl Pts',(0.213825927605133,0.102621378922579,
-1.81904233525338));
#66811=CARTESIAN_POINT('Ctrl Pts',(0.214472400358779,0.101262143515778,
-1.81914462488984));
#66812=CARTESIAN_POINT('Ctrl Pts',(0.214758461757127,0.100654038017529,
-1.81919013972173));
#66813=CARTESIAN_POINT('Ctrl Pts',(0.215339168592224,0.0994058328464185,
-1.81928304445913));
#66814=CARTESIAN_POINT('Ctrl Pts',(0.215633552271421,0.0987656230764895,
-1.81933041843311));
#66815=CARTESIAN_POINT('Ctrl Pts',(0.216386146042179,0.0971095174691044,
-1.81945227614837));
#66816=CARTESIAN_POINT('Ctrl Pts',(0.216840063503095,0.096091672710009,
-1.81952650281159));
#66817=CARTESIAN_POINT('Ctrl Pts',(0.218755428779171,0.0917140479537584,
-1.81984304986639));
#66818=CARTESIAN_POINT('Ctrl Pts',(0.22014618113985,0.0883236476538218,
-1.82008144570525));
#66819=CARTESIAN_POINT('Ctrl Pts',(0.223800386771826,0.0787920562297992,
-1.82073665232227));
#66820=CARTESIAN_POINT('Ctrl Pts',(0.225889170826399,0.0725871625319044,
-1.82114619480944));
#66821=CARTESIAN_POINT('Ctrl Pts',(0.228782327710164,0.0626506272602354,
-1.82178690085556));
#66822=CARTESIAN_POINT('Ctrl Pts',(0.229757858455704,0.0589727228294529,
-1.82202084874544));
#66823=CARTESIAN_POINT('Ctrl Pts',(0.234889673513442,0.0375585172278741,
-1.82337208320385));
#66824=CARTESIAN_POINT('Ctrl Pts',(0.237079574940827,0.0194162524769529,
-1.82447973176487));
#66825=CARTESIAN_POINT('Ctrl Pts',(0.237187590033331,-0.00188090725826167,
-1.82585714436869));
#66826=CARTESIAN_POINT('Ctrl Pts',(0.237143083508221,-0.0049645937470575,
-1.82605829387516));
#66827=CARTESIAN_POINT('Ctrl Pts',(0.236987875577185,-0.00953684228642896,
-1.8263594853224));
#66828=CARTESIAN_POINT('Ctrl Pts',(0.236923227625293,-0.0110267208193047,
-1.82645809244125));
#66829=CARTESIAN_POINT('Ctrl Pts',(0.236782711563533,-0.0136857833778987,
-1.82663495366969));
#66830=CARTESIAN_POINT('Ctrl Pts',(0.236712221404468,-0.0148552117198704,
-1.82671303692317));
#66831=CARTESIAN_POINT('Ctrl Pts',(0.236544547503257,-0.0173313138987364,
-1.8268790285168));
#66832=CARTESIAN_POINT('Ctrl Pts',(0.236445194116183,-0.0186377964005856,
-1.82696700240654));
#66833=CARTESIAN_POINT('Ctrl Pts',(0.23614979072489,-0.0221384174290009,
-1.82720380306762));
#66834=CARTESIAN_POINT('Ctrl Pts',(0.235933992795775,-0.0243307142868619,
-1.82735324346547));
#66835=CARTESIAN_POINT('Ctrl Pts',(0.234635697439217,-0.0358690467146313,
-1.82814602460467));
#66836=CARTESIAN_POINT('Ctrl Pts',(0.233028462332726,-0.0451463579057098,
-1.82880564188899));
#66837=CARTESIAN_POINT('Ctrl Pts',(0.228443559405747,-0.0646396449436121,
-1.83023822411047));
#66838=CARTESIAN_POINT('Ctrl Pts',(0.225320948591251,-0.0748009698632225,
-1.83101339990323));
#66839=CARTESIAN_POINT('Ctrl Pts',(0.217236987229194,-0.0959396106555246,
-1.83266618307894));
#66840=CARTESIAN_POINT('Ctrl Pts',(0.212098743571396,-0.106819933349215,
-1.83354162760002));
#66841=CARTESIAN_POINT('Ctrl Pts',(0.205128663422169,-0.119073685059738,
-1.83452510304342));
#66842=CARTESIAN_POINT('Ctrl Pts',(0.204075981014947,-0.120868961040342,
-1.83466909723506));
#66843=CARTESIAN_POINT('Ctrl Pts',(0.202568099176248,-0.123364673191028,
-1.83486889655289));
#66844=CARTESIAN_POINT('Ctrl Pts',(0.20213265977402,-0.124076852397924,
-1.83492586804764));
#66845=CARTESIAN_POINT('Ctrl Pts',(0.201339694745126,-0.125358526016224,
-1.83502829738034));
#66846=CARTESIAN_POINT('Ctrl Pts',(0.200983490731757,-0.125928826003704,
-1.83507383892603));
#66847=CARTESIAN_POINT('Ctrl Pts',(0.200249392987781,-0.127093102923555,
-1.83516672708757));
#66848=CARTESIAN_POINT('Ctrl Pts',(0.199871272496017,-0.127686924414544,
-1.83521405827665));
#66849=CARTESIAN_POINT('Ctrl Pts',(0.198889442970073,-0.129213796104573,
-1.83533566706376));
#66850=CARTESIAN_POINT('Ctrl Pts',(0.198281801578081,-0.13014431571462,
-1.83540968962578));
#66851=CARTESIAN_POINT('Ctrl Pts',(0.195659140593141,-0.134099553284646,
-1.83572410174785));
#66852=CARTESIAN_POINT('Ctrl Pts',(0.193581160970091,-0.137082191109466,
-1.83596063247336));
#66853=CARTESIAN_POINT('Ctrl Pts',(0.187619430405574,-0.145233295922761,
-1.83660899642791));
#66854=CARTESIAN_POINT('Ctrl Pts',(0.183591580251059,-0.150292729834986,
-1.83701374402225));
#66855=CARTESIAN_POINT('Ctrl Pts',(0.176474595520834,-0.158518672669928,
-1.83768743028312));
#66856=CARTESIAN_POINT('Ctrl Pts',(0.173494785823795,-0.161774575345168,
-1.83795855102901));
#66857=CARTESIAN_POINT('Ctrl Pts',(0.15814076627188,-0.177638732782072,
-1.83931257757304));
#66858=CARTESIAN_POINT('Ctrl Pts',(0.144477710736296,-0.188918308839718,
-1.84038893672197));
#66859=CARTESIAN_POINT('Ctrl Pts',(0.12707407283701,-0.200284601411832,
-1.84173284868373));
#66860=CARTESIAN_POINT('Ctrl Pts',(0.124424882131842,-0.201941052712327,
-1.84193658444565));
#66861=CARTESIAN_POINT('Ctrl Pts',(0.120457309818049,-0.204314131750754,
-1.84224091372841));
#66862=CARTESIAN_POINT('Ctrl Pts',(0.119163535633641,-0.205071401037203,
-1.84234002803086));
#66863=CARTESIAN_POINT('Ctrl Pts',(0.116845143993157,-0.206399050165758,
-1.84251746349776));
#66864=CARTESIAN_POINT('Ctrl Pts',(0.115823302486003,-0.206974196702347,
-1.84259560968766));
#66865=CARTESIAN_POINT('Ctrl Pts',(0.113654308927228,-0.208173928917217,
-1.84276138275939));
#66866=CARTESIAN_POINT('Ctrl Pts',(0.112506181740366,-0.208796660821598,
-1.84284907257368));
#66867=CARTESIAN_POINT('Ctrl Pts',(0.109425319930819,-0.210434898677635,
-1.84308425139582));
#66868=CARTESIAN_POINT('Ctrl Pts',(0.107483647613497,-0.211433233345502,
-1.84323233919946));
#66869=CARTESIAN_POINT('Ctrl Pts',(0.0973816543078754,-0.216452185349494,
-1.84400235335656));
#66870=CARTESIAN_POINT('Ctrl Pts',(0.0890097058776161,-0.220027202977841,
-1.84463943972918));
#66871=CARTESIAN_POINT('Ctrl Pts',(0.0702608810731703,-0.226788008117977,
-1.84606328788048));
#66872=CARTESIAN_POINT('Ctrl Pts',(0.0598284575954476,-0.229760562478916,
-1.84685395122733));
#66873=CARTESIAN_POINT('Ctrl Pts',(0.0373393350305363,-0.234532544069527,
-1.84853290704963));
#66874=CARTESIAN_POINT('Ctrl Pts',(0.0252708436418725,-0.236138060286027,
-1.84941900940058));
#66875=CARTESIAN_POINT('Ctrl Pts',(0.0110630306850422,-0.236925898578749,
-1.85041158955824));
#66876=CARTESIAN_POINT('Ctrl Pts',(0.00899312594283196,-0.237013494300426,
-1.85055492101486));
#66877=CARTESIAN_POINT('Ctrl Pts',(0.00608929338007281,-0.237098282458763,
-1.85075397032715));
#66878=CARTESIAN_POINT('Ctrl Pts',(0.00525619520105101,-0.237118214195767,
-1.85081084286576));
#66879=CARTESIAN_POINT('Ctrl Pts',(0.00375093002656609,-0.237146290242015,
-1.85091315855521));
#66880=CARTESIAN_POINT('Ctrl Pts',(0.00307880167948047,-0.237155968664331,
-1.85095868468695));
#66881=CARTESIAN_POINT('Ctrl Pts',(0.00170144037645741,-0.237169945529206,
-1.85105164023833));
#66882=CARTESIAN_POINT('Ctrl Pts',(0.000996215548390938,-0.237173956304892,
-1.85109905356954));
#66883=CARTESIAN_POINT('Ctrl Pts',(-0.000824408665852629,-0.237176189889346,
-1.85122101396435));
#66884=CARTESIAN_POINT('Ctrl Pts',(-0.00193981217147089,-0.237169690203402,
-1.85129530372941));
#66885=CARTESIAN_POINT('Ctrl Pts',(-0.00672236624312382,-0.237108078906661,
-1.85161215793729));
#66886=CARTESIAN_POINT('Ctrl Pts',(-0.0103882357251234,-0.236975778189748,
-1.85185079362262));
#66887=CARTESIAN_POINT('Ctrl Pts',(-0.0205911832038786,-0.236370311544264,
-1.85250682793523));
#66888=CARTESIAN_POINT('Ctrl Pts',(-0.0271141607436452,-0.235711170147424,
-1.8529169462639));
#66889=CARTESIAN_POINT('Ctrl Pts',(-0.0358713947009013,-0.234457842276661,
-1.85346464732926));
#66890=CARTESIAN_POINT('Ctrl Pts',(-0.0381360953048283,-0.234100139367924,
-1.85360601918351));
#66891=CARTESIAN_POINT('Ctrl Pts',(-0.0601113142505172,-0.23030185762165,
-1.85497798506941));
#66892=CARTESIAN_POINT('Ctrl Pts',(-0.0793146302337192,-0.224413514151641,
-1.85618678514247));
#66893=CARTESIAN_POINT('Ctrl Pts',(-0.100149646615677,-0.215012000629097,
-1.85766774619856));
#66894=CARTESIAN_POINT('Ctrl Pts',(-0.102727400341699,-0.213792404480238,
-1.85785396715669));
#66895=CARTESIAN_POINT('Ctrl Pts',(-0.106595565747967,-0.211876174690437,
-1.85813830122538));
#66896=CARTESIAN_POINT('Ctrl Pts',(-0.107902597174045,-0.21121353507617,
-1.85823523629233));
#66897=CARTESIAN_POINT('Ctrl Pts',(-0.110189865027876,-0.210027163087761,
-1.85840643094883));
#66898=CARTESIAN_POINT('Ctrl Pts',(-0.111172727103218,-0.209508568478321,
-1.85848050799205));
#66899=CARTESIAN_POINT('Ctrl Pts',(-0.113277237293965,-0.208379171833997,
-1.85864024789927));
#66900=CARTESIAN_POINT('Ctrl Pts',(-0.11439766445566,-0.207766181077483,
-1.85872598681694));
#66901=CARTESIAN_POINT('Ctrl Pts',(-0.11668704510527,-0.206489517742784,
-1.85890263332605));
#66902=CARTESIAN_POINT('Ctrl Pts',(-0.117855414556305,-0.205824897820943,
-1.85899357264267));
#66903=CARTESIAN_POINT('Ctrl Pts',(-0.120749661278421,-0.204145799884859,
-1.85922084518851));
#66904=CARTESIAN_POINT('Ctrl Pts',(-0.122468435365179,-0.203119349697744,
-1.85935760513207));
#66905=CARTESIAN_POINT('Ctrl Pts',(-0.127288183597471,-0.200157586826751,
-1.85974627769366));
#66906=CARTESIAN_POINT('Ctrl Pts',(-0.130357590998437,-0.19817224126737,
-1.85999995924093));
#66907=CARTESIAN_POINT('Ctrl Pts',(-0.140760178193324,-0.191097405309512,
-1.86088137071236));
#66908=CARTESIAN_POINT('Ctrl Pts',(-0.147850636320891,-0.185665846099503,
-1.86152059901013));
#66909=CARTESIAN_POINT('Ctrl Pts',(-0.164280923778104,-0.171540538330984,
-1.86309183401066));
#66910=CARTESIAN_POINT('Ctrl Pts',(-0.173258822725673,-0.162467707772275,
-1.86403027489312));
#66911=CARTESIAN_POINT('Ctrl Pts',(-0.185812852589775,-0.147550574914649,
-1.86543548560185));
#66912=CARTESIAN_POINT('Ctrl Pts',(-0.189939139180032,-0.142199614228725,
-1.86591569649194));
#66913=CARTESIAN_POINT('Ctrl Pts',(-0.194628602336177,-0.135549252179181,
-1.86647809355813));
#66914=CARTESIAN_POINT('Ctrl Pts',(-0.195415578686871,-0.134412218379724,
-1.86657308458988));
#66915=CARTESIAN_POINT('Ctrl Pts',(-0.196626335087387,-0.132629788697261,
-1.86672011072611));
#66916=CARTESIAN_POINT('Ctrl Pts',(-0.197056969034579,-0.131989118860632,
-1.86677258290071));
#66917=CARTESIAN_POINT('Ctrl Pts',(-0.197848065857735,-0.13079967320799,
-1.86686929356309));
#66918=CARTESIAN_POINT('Ctrl Pts',(-0.198209378410447,-0.130251502882987,
-1.86691358632051));
#66919=CARTESIAN_POINT('Ctrl Pts',(-0.199032960629449,-0.128990630623477,
-1.86701483834222));
#66920=CARTESIAN_POINT('Ctrl Pts',(-0.199493681761564,-0.128276939466522,
-1.86707169515392));
#66921=CARTESIAN_POINT('Ctrl Pts',(-0.200924291641534,-0.126034469097009,
-1.86724897566372));
#66922=CARTESIAN_POINT('Ctrl Pts',(-0.201880544132622,-0.12449700705014,
-1.86736854389031));
#66923=CARTESIAN_POINT('Ctrl Pts',(-0.204095344717588,-0.12084341839375,
-1.86764842615613));
#66924=CARTESIAN_POINT('Ctrl Pts',(-0.205338755149752,-0.118718314401139,
-1.86780790769662));
#66925=CARTESIAN_POINT('Ctrl Pts',(-0.209759972332458,-0.110884694427224,
-1.86838525710799));
#66926=CARTESIAN_POINT('Ctrl Pts',(-0.212734835616159,-0.105064568502138,
-1.86879412521511));
#66927=CARTESIAN_POINT('Ctrl Pts',(-0.222835441311536,-0.0831099172756618,
-1.87029018363164));
#66928=CARTESIAN_POINT('Ctrl Pts',(-0.22839559577176,-0.0663199965379573,
-1.87134930950847));
#66929=CARTESIAN_POINT('Ctrl Pts',(-0.233342763019596,-0.0429251512636557,
-1.87286049976554));
#66930=CARTESIAN_POINT('Ctrl Pts',(-0.234397330451919,-0.0367327425098595,
-1.87326317853471));
#66931=CARTESIAN_POINT('Ctrl Pts',(-0.235463468218853,-0.0285127411615625,
-1.87380497609718));
#66932=CARTESIAN_POINT('Ctrl Pts',(-0.235696658365334,-0.0265161478848097,
-1.87393712798372));
#66933=CARTESIAN_POINT('Ctrl Pts',(-0.236035478295466,-0.023255981006669,
-1.87415392337934));
#66934=CARTESIAN_POINT('Ctrl Pts',(-0.236156406592251,-0.0219940716077888,
-1.87423808373788));
#66935=CARTESIAN_POINT('Ctrl Pts',(-0.236365238049562,-0.0196140911963583,
-1.87439730092783));
#66936=CARTESIAN_POINT('Ctrl Pts',(-0.2364553387219,-0.0184962441299297,
-1.87447228634766));
#66937=CARTESIAN_POINT('Ctrl Pts',(-0.236621627272399,-0.0162328136701359,
-1.87462454586558));
#66938=CARTESIAN_POINT('Ctrl Pts',(-0.236697431439527,-0.0150872330738839,
-1.87470182994859));
#66939=CARTESIAN_POINT('Ctrl Pts',(-0.236885405409102,-0.0118948426179452,
-1.87491783635867));
#66940=CARTESIAN_POINT('Ctrl Pts',(-0.236979359191677,-0.00984710277714088,
-1.87505712398689));
#66941=CARTESIAN_POINT('Ctrl Pts',(-0.237133582672749,-0.00515922991764161,
-1.87537774355154));
#66942=CARTESIAN_POINT('Ctrl Pts',(-0.237176322468442,-0.00251884913445103,
-1.87555959789399));
#66943=CARTESIAN_POINT('Ctrl Pts',(-0.237174968833357,0.000121589045928318,
-1.87574276215633));
#66944=CARTESIAN_POINT('Ctrl Pts',(-0.0419392741328075,0.233437524640348,
-1.89811014643447));
#66945=CARTESIAN_POINT('Ctrl Pts',(-0.0557647178783972,0.230953652023264,
-1.89716236890311));
#66946=CARTESIAN_POINT('Ctrl Pts',(-0.0694132968284817,0.227229285998194,
-1.89621459137175));
#66947=CARTESIAN_POINT('Ctrl Pts',(-0.0826482297992921,0.222308908359614,
-1.89526681384039));
#66948=CARTESIAN_POINT('Ctrl Pts',(-0.0958578704916535,0.217397933682242,
-1.89432084753492));
#66949=CARTESIAN_POINT('Ctrl Pts',(-0.108654636960885,0.211295710624007,
-1.89337488122945));
#66950=CARTESIAN_POINT('Ctrl Pts',(-0.120816083667543,0.204096679424819,
-1.89242891492398));
#66951=CARTESIAN_POINT('Ctrl Pts',(-0.132976886900327,0.196898029133314,
-1.8914829986705));
#66952=CARTESIAN_POINT('Ctrl Pts',(-0.14450169745988,0.188603071532895,
-1.89053708241702));
#66953=CARTESIAN_POINT('Ctrl Pts',(-0.155192756435186,0.179352136800901,
-1.88959116616354));
#66954=CARTESIAN_POINT('Ctrl Pts',(-0.165883101262724,0.170101820018392,
-1.88864531309594));
#66955=CARTESIAN_POINT('Ctrl Pts',(-0.175739189356455,0.159896216519811,
-1.88769946002834));
#66956=CARTESIAN_POINT('Ctrl Pts',(-0.184598172414416,0.148914389386176,
-1.88675360696074));
#66957=CARTESIAN_POINT('Ctrl Pts',(-0.193477638346253,0.137907171146288,
-1.88580556698422));
#66958=CARTESIAN_POINT('Ctrl Pts',(-0.201354913365268,0.126120829148612,
-1.8848575270077));
#66959=CARTESIAN_POINT('Ctrl Pts',(-0.208109274133015,0.113765155670924,
-1.88390948703118));
#66960=CARTESIAN_POINT('Ctrl Pts',(-0.211371365641569,0.107797849671148,
-1.88345162088166));
#66961=CARTESIAN_POINT('Ctrl Pts',(-0.214372225391734,0.101698120202883,
-1.88299375473214));
#66962=CARTESIAN_POINT('Ctrl Pts',(-0.217102271967589,0.0954912777771402,
-1.88253588858262));
#66963=CARTESIAN_POINT('Ctrl Pts',(-0.223316722733585,0.0813625383599422,
-1.88149364019435));
#66964=CARTESIAN_POINT('Ctrl Pts',(-0.228161089732516,0.0665956597385658,
-1.88045139180608));
#66965=CARTESIAN_POINT('Ctrl Pts',(-0.231525608196456,0.0514574909440909,
-1.87940914341781));
#66966=CARTESIAN_POINT('Ctrl Pts',(-0.234866127370754,0.0364273035149854,
-1.87837432944287));
#66967=CARTESIAN_POINT('Ctrl Pts',(-0.236747587829712,0.0210316072282276,
-1.87733951546794));
#66968=CARTESIAN_POINT('Ctrl Pts',(-0.237110022140893,0.00555139850354441,
-1.87630470149301));
#66969=CARTESIAN_POINT('Ctrl Pts',(-0.237152481940009,0.00373786558891791,
-1.87618347126689));
#66970=CARTESIAN_POINT('Ctrl Pts',(-0.23717415009495,0.00192319013249233,
-1.87606224104077));
#66971=CARTESIAN_POINT('Ctrl Pts',(-0.237174975484837,0.000107836760217876,
-1.87594101081465));
#66972=CARTESIAN_POINT('',(-0.237174951380842,0.000151863410009322,-1.8956589891905));
#66973=CARTESIAN_POINT('Ctrl Pts',(-0.0419392741328073,0.233437524640348,
-1.91783866303197));
#66974=CARTESIAN_POINT('Ctrl Pts',(-0.0558822279275878,0.230932540223977,
-1.91688952349866));
#66975=CARTESIAN_POINT('Ctrl Pts',(-0.0695810299052555,0.22717752105336,
-1.91594038396535));
#66976=CARTESIAN_POINT('Ctrl Pts',(-0.0828055599448024,0.222250354031726,
-1.91499124443204));
#66977=CARTESIAN_POINT('Ctrl Pts',(-0.0913653365601734,0.219061170830079,
-1.91437689954737));
#66978=CARTESIAN_POINT('Ctrl Pts',(-0.0997267139021598,0.215381955367923,
-1.91376255466271));
#66979=CARTESIAN_POINT('Ctrl Pts',(-0.107832458568548,0.211244269754383,
-1.91314820977804));
#66980=CARTESIAN_POINT('Ctrl Pts',(-0.120360313440485,0.204849258931122,
-1.91219870743455));
#66981=CARTESIAN_POINT('Ctrl Pts',(-0.132357915464483,0.197315221878836,
-1.91124920509106));
#66982=CARTESIAN_POINT('Ctrl Pts',(-0.143610941870615,0.188753484736136,
-1.91029970274757));
#66983=CARTESIAN_POINT('Ctrl Pts',(-0.154841841101612,0.18020858280295,
-1.90935206744002));
#66984=CARTESIAN_POINT('Ctrl Pts',(-0.16533037523629,0.170640436808729,
-1.90840443213246));
#66985=CARTESIAN_POINT('Ctrl Pts',(-0.174890356906369,0.160204068881421,
-1.9074567968249));
#66986=CARTESIAN_POINT('Ctrl Pts',(-0.184449345255448,0.14976878533521,
-1.90650925998051));
#66987=CARTESIAN_POINT('Ctrl Pts',(-0.193079377014223,0.138466038552127,
-1.90556172313612));
#66988=CARTESIAN_POINT('Ctrl Pts',(-0.200631105799812,0.126487706954251,
-1.90461418629173));
#66989=CARTESIAN_POINT('Ctrl Pts',(-0.208181830959439,0.114510967278559,
-1.90366677537514));
#66990=CARTESIAN_POINT('Ctrl Pts',(-0.214654110773553,0.101859535013325,
-1.90271936445854));
#66991=CARTESIAN_POINT('Ctrl Pts',(-0.219943163533292,0.0887523827283964,
-1.90177195354195));
#66992=CARTESIAN_POINT('Ctrl Pts',(-0.225244659434385,0.0756143942699501,
-1.90082231372569));
#66993=CARTESIAN_POINT('Ctrl Pts',(-0.229357100911607,0.0620193346874439,
-1.89987267390942));
#66994=CARTESIAN_POINT('Ctrl Pts',(-0.232224865083146,0.0482036581818705,
-1.89892303409316));
#66995=CARTESIAN_POINT('Ctrl Pts',(-0.233894591620518,0.0401596209761488,
-1.89837011596345));
#66996=CARTESIAN_POINT('Ctrl Pts',(-0.235143329028863,0.0320410305536099,
-1.89781719783375));
#66997=CARTESIAN_POINT('Ctrl Pts',(-0.235968201078832,0.0238953699410578,
-1.89726427970405));
#66998=CARTESIAN_POINT('Ctrl Pts',(-0.236766486397861,0.0160122548797073,
-1.8967291828662));
#66999=CARTESIAN_POINT('Ctrl Pts',(-0.237169869832119,0.00808804811135685,
-1.89619408602835));
#67000=CARTESIAN_POINT('Ctrl Pts',(-0.237174951380842,0.000151863410009322,
-1.8956589891905));
#67001=CARTESIAN_POINT('Ctrl Pts',(-0.237174944447511,0.000162330896843699,
-1.89549312073154));
#67002=CARTESIAN_POINT('Ctrl Pts',(-0.237184634811181,-0.0139958577776726,
-1.89459963185786));
#67003=CARTESIAN_POINT('Ctrl Pts',(-0.235926558959752,-0.0281278877879236,
-1.89374477756997));
#67004=CARTESIAN_POINT('Ctrl Pts',(-0.231083450137942,-0.0550021575796279,
-1.89206500264375));
#67005=CARTESIAN_POINT('Ctrl Pts',(-0.227680677881489,-0.0677217709568628,
-1.89124514588661));
#67006=CARTESIAN_POINT('Ctrl Pts',(-0.222445439750269,-0.0823138738571256,
-1.89023594839191));
#67007=CARTESIAN_POINT('Ctrl Pts',(-0.221615602453172,-0.0845226099006235,
-1.89008131918506));
#67008=CARTESIAN_POINT('Ctrl Pts',(-0.220263814763681,-0.0879637560919081,
-1.88983728224874));
#67009=CARTESIAN_POINT('Ctrl Pts',(-0.219764135091431,-0.0892047940555895,
-1.88974862573526));
#67010=CARTESIAN_POINT('Ctrl Pts',(-0.218812432448759,-0.0915119712257564,
-1.889582566415));
#67011=CARTESIAN_POINT('Ctrl Pts',(-0.218363047202494,-0.0925791607530103,
-1.8895052554225));
#67012=CARTESIAN_POINT('Ctrl Pts',(-0.217343636753233,-0.0949513137335354,
-1.88933226837249));
#67013=CARTESIAN_POINT('Ctrl Pts',(-0.216769641181143,-0.0962545111880764,
-1.88923645823292));
#67014=CARTESIAN_POINT('Ctrl Pts',(-0.215286426228996,-0.0995414334624076,
-1.88899279559419));
#67015=CARTESIAN_POINT('Ctrl Pts',(-0.214361517129657,-0.101517888615515,
-1.88884440631225));
#67016=CARTESIAN_POINT('Ctrl Pts',(-0.207030084992107,-0.116637510019767,
-1.88769442986415));
#67017=CARTESIAN_POINT('Ctrl Pts',(-0.199448979523235,-0.129173240309845,
-1.88665102448432));
#67018=CARTESIAN_POINT('Ctrl Pts',(-0.183174348102441,-0.151202777242698,
-1.88465772615423));
#67019=CARTESIAN_POINT('Ctrl Pts',(-0.174767310243425,-0.160846262397933,
-1.88371656013858));
#67020=CARTESIAN_POINT('Ctrl Pts',(-0.162872252175924,-0.172451138215211,
-1.88252447175839));
#67021=CARTESIAN_POINT('Ctrl Pts',(-0.160054919331403,-0.175069105875549,
-1.88225118622152));
#67022=CARTESIAN_POINT('Ctrl Pts',(-0.155882235161675,-0.178761543374882,
-1.88186074051206));
#67023=CARTESIAN_POINT('Ctrl Pts',(-0.154576957411494,-0.179891426335815,
-1.88174055174873));
#67024=CARTESIAN_POINT('Ctrl Pts',(-0.152240612567697,-0.181869619765219,
-1.88152902085354));
#67025=CARTESIAN_POINT('Ctrl Pts',(-0.151214514026267,-0.182723653819556,
-1.88143732053154));
#67026=CARTESIAN_POINT('Ctrl Pts',(-0.149595250030316,-0.184048403933412,
-1.88129455392657));
#67027=CARTESIAN_POINT('Ctrl Pts',(-0.149006967933456,-0.184525004728834,
-1.88124308264791));
#67028=CARTESIAN_POINT('Ctrl Pts',(-0.147939873196809,-0.185381087970523,
-1.88115044673451));
#67029=CARTESIAN_POINT('Ctrl Pts',(-0.147461877763405,-0.185761536589055,
-1.8811092144553));
#67030=CARTESIAN_POINT('Ctrl Pts',(-0.146341403284033,-0.186646300199484,
-1.88101316627766));
#67031=CARTESIAN_POINT('Ctrl Pts',(-0.145697783590055,-0.187149148008554,
-1.88095845441033));
#67032=CARTESIAN_POINT('Ctrl Pts',(-0.144035796094616,-0.188433856768741,
-1.88081831502408));
#67033=CARTESIAN_POINT('Ctrl Pts',(-0.143013638585458,-0.189210803845375,
-1.88073321748207));
#67034=CARTESIAN_POINT('Ctrl Pts',(-0.13624011529885,-0.194273141411539,
-1.88017607107161));
#67035=CARTESIAN_POINT('Ctrl Pts',(-0.130302591288763,-0.198304511268763,
-1.87971952406197));
#67036=CARTESIAN_POINT('Ctrl Pts',(-0.111330316063401,-0.209965267756706,
-1.8783263351731));
#67037=CARTESIAN_POINT('Ctrl Pts',(-0.0977441774117247,-0.2166240225215,
-1.87741762174244));
#67038=CARTESIAN_POINT('Ctrl Pts',(-0.0735408108175652,-0.225742475739598,
-1.87581509773933));
#67039=CARTESIAN_POINT('Ctrl Pts',(-0.0632192353012449,-0.22884754835643,
-1.87513677632853));
#67040=CARTESIAN_POINT('Ctrl Pts',(-0.0504987335144055,-0.231747846824982,
-1.87428643717059));
#67041=CARTESIAN_POINT('Ctrl Pts',(-0.0482670265010115,-0.232222910483537,
-1.87413676407644));
#67042=CARTESIAN_POINT('Ctrl Pts',(-0.0447247916369375,-0.232923680269989,
-1.87389826712956));
#67043=CARTESIAN_POINT('Ctrl Pts',(-0.043418585282702,-0.233170697446638,
-1.87381012212225));
#67044=CARTESIAN_POINT('Ctrl Pts',(-0.0409570690840748,-0.233614795274303,
-1.87364360984173));
#67045=CARTESIAN_POINT('Ctrl Pts',(-0.0398022364022077,-0.233814319432332,
-1.87356532275594));
#67046=CARTESIAN_POINT('Ctrl Pts',(-0.0371961175448163,-0.234244720174029,
-1.87338825345078));
#67047=CARTESIAN_POINT('Ctrl Pts',(-0.035744080114253,-0.234470681872684,
-1.87328931905078));
#67048=CARTESIAN_POINT('Ctrl Pts',(-0.0314564437638208,-0.235097157778114,
-1.87299631617937));
#67049=CARTESIAN_POINT('Ctrl Pts',(-0.0286156702447432,-0.235459813170809,
-1.87280107089615));
#67050=CARTESIAN_POINT('Ctrl Pts',(-0.00607571946853295,-0.23792336944405,
-1.87124246550739));
#67051=CARTESIAN_POINT('Ctrl Pts',(0.0138062545315421,-0.237599495419691,
-1.86980086325133));
#67052=CARTESIAN_POINT('Ctrl Pts',(0.0356711915459823,-0.234488285018245,
-1.86819004997522));
#67053=CARTESIAN_POINT('Ctrl Pts',(0.0379260362484901,-0.234134161698333,
-1.86802375445623));
#67054=CARTESIAN_POINT('Ctrl Pts',(0.0466792913279063,-0.232629693084337,
-1.86737813726479));
#67055=CARTESIAN_POINT('Ctrl Pts',(0.0531341105863897,-0.231240801438476,
-1.86690183691386));
#67056=CARTESIAN_POINT('Ctrl Pts',(0.0630905107760069,-0.228659464811337,
-1.86617415332546));
#67057=CARTESIAN_POINT('Ctrl Pts',(0.0666362464695275,-0.227651439141091,
-1.86591644081523));
#67058=CARTESIAN_POINT('Ctrl Pts',(0.0712267750376253,-0.226229928730689,
-1.8655858998817));
#67059=CARTESIAN_POINT('Ctrl Pts',(0.0722939425948105,-0.225891168761478,
-1.8655092805891));
#67060=CARTESIAN_POINT('Ctrl Pts',(0.0740317263022084,-0.225325952815515,
-1.86538492139253));
#67061=CARTESIAN_POINT('Ctrl Pts',(0.0747037832309765,-0.225104034428257,
-1.86533692786114));
#67062=CARTESIAN_POINT('Ctrl Pts',(0.0760130376177374,-0.2246651993077,
-1.86524363968965));
#67063=CARTESIAN_POINT('Ctrl Pts',(0.0766503173732511,-0.224448574351676,
-1.86519833018889));
#67064=CARTESIAN_POINT('Ctrl Pts',(0.0780755269895758,-0.223957337300892,
-1.86509720405988));
#67065=CARTESIAN_POINT('Ctrl Pts',(0.0788629556942779,-0.223681271270112,
-1.86504147165853));
#67066=CARTESIAN_POINT('Ctrl Pts',(0.0816026596227852,-0.222704487702123,
-1.86484799564965));
#67067=CARTESIAN_POINT('Ctrl Pts',(0.083547253596568,-0.221982296669889,
-1.86471144037634));
#67068=CARTESIAN_POINT('Ctrl Pts',(0.0967670071953243,-0.216874355296772,
-1.86378676723038));
#67069=CARTESIAN_POINT('Ctrl Pts',(0.107703178028697,-0.211656420477618,
-1.86303960269599));
#67070=CARTESIAN_POINT('Ctrl Pts',(0.127520715768036,-0.200265232626141,
-1.86163625154334));
#67071=CARTESIAN_POINT('Ctrl Pts',(0.136471278748143,-0.194276290790153,
-1.86098072229129));
#67072=CARTESIAN_POINT('Ctrl Pts',(0.152261756939972,-0.182079382547959,
-1.85973699341377));
#67073=CARTESIAN_POINT('Ctrl Pts',(0.159205505579167,-0.176040112756565,
-1.85915400034019));
#67074=CARTESIAN_POINT('Ctrl Pts',(0.167346648273412,-0.168082940673496,
-1.85841132850765));
#67075=CARTESIAN_POINT('Ctrl Pts',(0.16889131157139,-0.166530777883194,
-1.85826757948975));
#67076=CARTESIAN_POINT('Ctrl Pts',(0.171323703491092,-0.164017923394397,
-1.85803647922126));
#67077=CARTESIAN_POINT('Ctrl Pts',(0.172225384605834,-0.163070866048064,
-1.85794973829414));
#67078=CARTESIAN_POINT('Ctrl Pts',(0.173920588187102,-0.161260609887282,
-1.85778457888987));
#67079=CARTESIAN_POINT('Ctrl Pts',(0.174715633705693,-0.160398885751305,
-1.85770622916352));
#67080=CARTESIAN_POINT('Ctrl Pts',(0.176511105732669,-0.158423643698509,
-1.857527223829));
#67081=CARTESIAN_POINT('Ctrl Pts',(0.177507436745531,-0.157306487631131,
-1.8574263999426));
#67082=CARTESIAN_POINT('Ctrl Pts',(0.180542366063355,-0.153837964311554,
-1.85711458647974));
#67083=CARTESIAN_POINT('Ctrl Pts',(0.182545242289507,-0.151455927980086,
-1.85690214316056));
#67084=CARTESIAN_POINT('Ctrl Pts',(0.195749072900072,-0.135110035056083,
-1.85545492185889));
#67085=CARTESIAN_POINT('Ctrl Pts',(0.2053828610913,-0.119958606548223,-1.85415803876152));
#67086=CARTESIAN_POINT('Ctrl Pts',(0.215038755403543,-0.100137732087421,
-1.85254753678398));
#67087=CARTESIAN_POINT('Ctrl Pts',(0.216759393908215,-0.0963566170039159,
-1.85224419311605));
#67088=CARTESIAN_POINT('Ctrl Pts',(0.220922478150781,-0.086531567122758,
-1.85146825662011));
#67089=CARTESIAN_POINT('Ctrl Pts',(0.22321685612571,-0.0804282293298775,
-1.85099784207076));
#67090=CARTESIAN_POINT('Ctrl Pts',(0.226400825825719,-0.0707672208891036,
-1.85027812974325));
#67091=CARTESIAN_POINT('Ctrl Pts',(0.227464328460476,-0.067270471932179,
-1.85002259891089));
#67092=CARTESIAN_POINT('Ctrl Pts',(0.22874586359911,-0.0626781427933214,
-1.84969463707151));
#67093=CARTESIAN_POINT('Ctrl Pts',(0.229037519483508,-0.061603851257538,
-1.84961845584768));
#67094=CARTESIAN_POINT('Ctrl Pts',(0.229501311461506,-0.0598466749729449,
-1.8494947725221));
#67095=CARTESIAN_POINT('Ctrl Pts',(0.229677984765912,-0.0591650218863398,
-1.84944701851049));
#67096=CARTESIAN_POINT('Ctrl Pts',(0.230017147733215,-0.0578320239696665,
-1.8493540880373));
#67097=CARTESIAN_POINT('Ctrl Pts',(0.230179911544511,-0.0571807623722538,
-1.84930889720696));
#67098=CARTESIAN_POINT('Ctrl Pts',(0.23053828631472,-0.0557204802656415,
-1.84920802582521));
#67099=CARTESIAN_POINT('Ctrl Pts',(0.230732410112268,-0.0549110949968989,
-1.84915242945969));
#67100=CARTESIAN_POINT('Ctrl Pts',(0.231394376746947,-0.052085570196356,
-1.84895938205504));
#67101=CARTESIAN_POINT('Ctrl Pts',(0.231840103265428,-0.050064273154927,
-1.84882311791282));
#67102=CARTESIAN_POINT('Ctrl Pts',(0.234724276832261,-0.0361193597687741,
-1.84789399314954));
#67103=CARTESIAN_POINT('Ctrl Pts',(0.236268574193361,-0.0240277295893806,
-1.84714273569856));
#67104=CARTESIAN_POINT('Ctrl Pts',(0.237422862085469,-0.000992052638308131,
-1.84572718424032));
#67105=CARTESIAN_POINT('Ctrl Pts',(0.237218004461241,0.009909990692749,
-1.84506365284641));
#67106=CARTESIAN_POINT('Ctrl Pts',(0.235473282860477,0.0297672532661437,
-1.84382050702397));
#67107=CARTESIAN_POINT('Ctrl Pts',(0.234167329857106,0.0387219479702918,
-1.84324691795644));
#67108=CARTESIAN_POINT('Ctrl Pts',(0.231916639982723,0.0497131348529717,
-1.84251496396376));
#67109=CARTESIAN_POINT('Ctrl Pts',(0.231450387475106,0.0518405371871796,
-1.84237199337972));
#67110=CARTESIAN_POINT('Ctrl Pts',(0.230658276485097,0.0552307891212038,
-1.84214193388744));
#67111=CARTESIAN_POINT('Ctrl Pts',(0.230351176628517,0.0564979281788567,
-1.8420554479519));
#67112=CARTESIAN_POINT('Ctrl Pts',(0.229748447653327,0.058898240960359,
-1.84189064052908));
#67113=CARTESIAN_POINT('Ctrl Pts',(0.229454841969792,0.0600318865189183,
-1.84181238655193));
#67114=CARTESIAN_POINT('Ctrl Pts',(0.228766587479204,0.0626104834683579,
-1.84163341499536));
#67115=CARTESIAN_POINT('Ctrl Pts',(0.228366624731581,0.0640539516055271,
-1.8415325276798));
#67116=CARTESIAN_POINT('Ctrl Pts',(0.22709032540394,0.0684961674646237,
-1.84121982902522));
#67117=CARTESIAN_POINT('Ctrl Pts',(0.226168421029031,0.0714813580847788,
-1.8410065478741));
#67118=CARTESIAN_POINT('Ctrl Pts',(0.219645360881962,0.0912122683677192,
-1.83957513821474));
#67119=CARTESIAN_POINT('Ctrl Pts',(0.212249019757952,0.107302797973203,
-1.83829672182847));
#67120=CARTESIAN_POINT('Ctrl Pts',(0.200866988495921,0.126189525921918,
-1.83668599610456));
#67121=CARTESIAN_POINT('Ctrl Pts',(0.198491235353379,0.129894472106342,
-1.83636456098707));
#67122=CARTESIAN_POINT('Ctrl Pts',(0.192361876016848,0.138891909783512,
-1.83557298816622));
#67123=CARTESIAN_POINT('Ctrl Pts',(0.188491356638195,0.14410091527999,-1.835104860218));
#67124=CARTESIAN_POINT('Ctrl Pts',(0.182121738318622,0.151976697045788,
-1.83438826168345));
#67125=CARTESIAN_POINT('Ctrl Pts',(0.179766493735932,0.154755469500671,
-1.83413361014865));
#67126=CARTESIAN_POINT('Ctrl Pts',(0.176610224117248,0.158309962085933,
-1.83380664145114));
#67127=CARTESIAN_POINT('Ctrl Pts',(0.175866572383603,0.159135678586182,
-1.83373059695881));
#67128=CARTESIAN_POINT('Ctrl Pts',(0.174642791121286,0.160475452311941,
-1.83360710818035));
#67129=CARTESIAN_POINT('Ctrl Pts',(0.1741661401743,0.160992642487537,-1.83355941285533));
#67130=CARTESIAN_POINT('Ctrl Pts',(0.173229561643626,0.161999849436406,
-1.83346649219864));
#67131=CARTESIAN_POINT('Ctrl Pts',(0.172769841476089,0.162490043202691,
-1.83342125293572));
#67132=CARTESIAN_POINT('Ctrl Pts',(0.171735111891281,0.163584006296584,
-1.83332023867585));
#67133=CARTESIAN_POINT('Ctrl Pts',(0.171158984147169,0.164186716789967,
-1.83326454831863));
#67134=CARTESIAN_POINT('Ctrl Pts',(0.169137266316699,0.166279510882546,
-1.83307098918828));
#67135=CARTESIAN_POINT('Ctrl Pts',(0.167675250491103,0.167753693522431,
-1.83293431354991));
#67136=CARTESIAN_POINT('Ctrl Pts',(0.157576201511409,0.177672822352053,
-1.83201076196862));
#67137=CARTESIAN_POINT('Ctrl Pts',(0.148323189318488,0.185467511110483,
-1.83126476813234));
#67138=CARTESIAN_POINT('Ctrl Pts',(0.129812952595336,0.198785092292248,
-1.82986496964348));
#67139=CARTESIAN_POINT('Ctrl Pts',(0.120696104130112,0.204448910574454,
-1.82921178507571));
#67140=CARTESIAN_POINT('Ctrl Pts',(0.103041103751826,0.213823357649805,
-1.82796624768861));
#67141=CARTESIAN_POINT('Ctrl Pts',(0.0946075770403748,0.217686180527965,
-1.827378813469));
#67142=CARTESIAN_POINT('Ctrl Pts',(0.0839251200256205,0.221840867631301,
-1.82663111859779));
#67143=CARTESIAN_POINT('Ctrl Pts',(0.0818690070886439,0.222607864799082,
-1.82648706987633));
#67144=CARTESIAN_POINT('Ctrl Pts',(0.0785702775611092,0.223786515705193,
-1.82625560572852));
#67145=CARTESIAN_POINT('Ctrl Pts',(0.0773343509236932,0.224216616641623,
-1.82616880435029));
#67146=CARTESIAN_POINT('Ctrl Pts',(0.0749847268885639,0.225012544963826,
-1.82600360571782));
#67147=CARTESIAN_POINT('Ctrl Pts',(0.0738717495269176,0.225380387776795,
-1.82592527785344));
#67148=CARTESIAN_POINT('Ctrl Pts',(0.0713332086653112,0.226198560836576,
-1.82574642806855));
#67149=CARTESIAN_POINT('Ctrl Pts',(0.0699060341096111,0.226643689080322,
-1.82564573887647));
#67150=CARTESIAN_POINT('Ctrl Pts',(0.0655046212560836,0.227970939430144,
-1.82533473324368));
#67151=CARTESIAN_POINT('Ctrl Pts',(0.0625173104459858,0.228808192458946,
-1.82512297401412));
#67152=CARTESIAN_POINT('Ctrl Pts',(0.0421326182723946,0.234092412119568,
-1.82367276592415));
#67153=CARTESIAN_POINT('Ctrl Pts',(0.024298328226178,0.236608897301523,
-1.82237178865636));
#67154=CARTESIAN_POINT('Ctrl Pts',(-0.00715941131273107,0.237452081302828,
-1.82007360149346));
#67155=CARTESIAN_POINT('Ctrl Pts',(-0.0206814933532748,0.236658204907083,
-1.81908679755903));
#67156=CARTESIAN_POINT('Ctrl Pts',(-0.0355525043970215,0.234500029678021,
-1.81804667772843));
#67157=CARTESIAN_POINT('Ctrl Pts',(-0.037039478066328,0.234269762977691,
-1.81794320048208));
#67158=CARTESIAN_POINT('Ctrl Pts',(-0.0393031790927103,0.233897122639109,
-1.81778657560314));
#67159=CARTESIAN_POINT('Ctrl Pts',(-0.0400815204268637,0.233765000869813,
-1.81773288588515));
#67160=CARTESIAN_POINT('Ctrl Pts',(-0.0412193742211361,0.233566002461466,
-1.81765465084603));
#67161=CARTESIAN_POINT('Ctrl Pts',(-0.0415793972373618,0.233502179951423,
-1.8176299341645));
#67162=CARTESIAN_POINT('Ctrl Pts',(-0.0419392741328096,0.233437524640348,
-1.81760526556689));
#67163=CARTESIAN_POINT('Origin',(0.,0.,-2.1456589891905));
#67164=CARTESIAN_POINT('',(-0.0419392692346775,0.233437525520344,-1.69793969278784));
#67165=CARTESIAN_POINT('',(-0.0419393124730349,0.233437517752158,-1.71790170279738));
#67166=CARTESIAN_POINT('',(-0.0419392741328076,0.233437524640348,-2.1456589891905));
#67167=CARTESIAN_POINT('Ctrl Pts',(-0.0419392692346775,0.233437525520344,
-1.69793969278784));
#67168=CARTESIAN_POINT('Ctrl Pts',(-0.0371287966350787,0.234301772624793,
-1.6982501843674));
#67169=CARTESIAN_POINT('Ctrl Pts',(-0.032292004561194,0.235017255155577,
-1.69856447585913));
#67170=CARTESIAN_POINT('Ctrl Pts',(-0.0252667305782954,0.235835411594207,
-1.69902590010247));
#67171=CARTESIAN_POINT('Ctrl Pts',(-0.0230943975890999,0.236058038017637,
-1.69916925119909));
#67172=CARTESIAN_POINT('Ctrl Pts',(-0.0196182458083198,0.236365841914204,
-1.69939985294673));
#67173=CARTESIAN_POINT('Ctrl Pts',(-0.0183162262750079,0.236470299470237,
-1.69948649738776));
#67174=CARTESIAN_POINT('Ctrl Pts',(-0.0158439214709464,0.236648105014684,
-1.69965156354595));
#67175=CARTESIAN_POINT('Ctrl Pts',(-0.014673821697801,0.23672353986501,
-1.69972991725923));
#67176=CARTESIAN_POINT('Ctrl Pts',(-0.0120067902043739,0.236875630287251,
-1.6999090584211));
#67177=CARTESIAN_POINT('Ctrl Pts',(-0.0105096072730364,0.236946777168043,
-1.70001001535038));
#67178=CARTESIAN_POINT('Ctrl Pts',(-0.00589094467926848,0.237122398173867,
-1.70032272188493));
#67179=CARTESIAN_POINT('Ctrl Pts',(-0.00276810692013724,0.237179406583153,
-1.70053593808214));
#67180=CARTESIAN_POINT('Ctrl Pts',(0.0180267418323495,0.237148296859321,
-1.70196826815008));
#67181=CARTESIAN_POINT('Ctrl Pts',(0.035637175020166,0.235146856451655,
-1.70324771751406));
#67182=CARTESIAN_POINT('Ctrl Pts',(0.0571333906288445,0.23023246264618,
-1.70485824146629));
#67183=CARTESIAN_POINT('Ctrl Pts',(0.061380482877471,0.229136746020173,
-1.70517853501963));
#67184=CARTESIAN_POINT('Ctrl Pts',(0.0718174415717139,0.226133067267341,
-1.70596810384619));
#67185=CARTESIAN_POINT('Ctrl Pts',(0.0779645775605586,0.224088029518718,
-1.70643536910158));
#67186=CARTESIAN_POINT('Ctrl Pts',(0.0874233130926202,0.220504839799236,
-1.70715089509841));
#67187=CARTESIAN_POINT('Ctrl Pts',(0.0907960691438752,0.219137622188636,
-1.70740530474828));
#67188=CARTESIAN_POINT('Ctrl Pts',(0.0951567347037798,0.217251956489909,
-1.70773208625057));
#67189=CARTESIAN_POINT('Ctrl Pts',(0.09617413444592,0.216803488773754,-1.70780817314177));
#67190=CARTESIAN_POINT('Ctrl Pts',(0.0978306600255841,0.216059339937072,
-1.70793175863884));
#67191=CARTESIAN_POINT('Ctrl Pts',(0.0984716748848465,0.215767944082327,
-1.70797950809556));
#67192=CARTESIAN_POINT('Ctrl Pts',(0.0997222949091607,0.21519269663022,
-1.7080725095042));
#67193=CARTESIAN_POINT('Ctrl Pts',(0.100332004183731,0.214909101107828,
-1.7081177753938));
#67194=CARTESIAN_POINT('Ctrl Pts',(0.101695781294438,0.21426769544878,-1.70821887467106));
#67195=CARTESIAN_POINT('Ctrl Pts',(0.102449190781078,0.213908486523314,
-1.70827462313361));
#67196=CARTESIAN_POINT('Ctrl Pts',(0.105073535010709,0.212640211518016,
-1.70846850461914));
#67197=CARTESIAN_POINT('Ctrl Pts',(0.106934458587307,0.211710485347377,
-1.70860543946312));
#67198=CARTESIAN_POINT('Ctrl Pts',(0.119464876992314,0.205242844945281,
-1.70952538823911));
#67199=CARTESIAN_POINT('Ctrl Pts',(0.1297135827923,0.198924465120284,-1.71026794446004));
#67200=CARTESIAN_POINT('Ctrl Pts',(0.1480384393526,0.18560600323059,-1.71165864432544));
#67201=CARTESIAN_POINT('Ctrl Pts',(0.156206923877903,0.17878578375222,-1.71230624536357));
#67202=CARTESIAN_POINT('Ctrl Pts',(0.170679347399284,0.164950769374471,
-1.71355311850542));
#67203=CARTESIAN_POINT('Ctrl Pts',(0.177076286558787,0.158063762872574,
-1.71414805101863));
#67204=CARTESIAN_POINT('Ctrl Pts',(0.184447904541046,0.149116733369563,
-1.7149042019278));
#67205=CARTESIAN_POINT('Ctrl Pts',(0.185824381896733,0.147397856893892,
-1.71504873788519));
#67206=CARTESIAN_POINT('Ctrl Pts',(0.187981341245023,0.144626113075517,
-1.71528079573552));
#67207=CARTESIAN_POINT('Ctrl Pts',(0.188777397481656,0.143585484373308,
-1.71536769763333));
#67208=CARTESIAN_POINT('Ctrl Pts',(0.190268987078782,0.141601787438656,
-1.71553296631488));
#67209=CARTESIAN_POINT('Ctrl Pts',(0.190966235412761,0.140660052954229,
-1.71561126267076));
#67210=CARTESIAN_POINT('Ctrl Pts',(0.192535305053894,0.138507626897638,
-1.71578987119754));
#67211=CARTESIAN_POINT('Ctrl Pts',(0.193402731252858,0.137293808191824,
-1.71589034910425));
#67212=CARTESIAN_POINT('Ctrl Pts',(0.196029412680728,0.133543911999489,
-1.71620006514583));
#67213=CARTESIAN_POINT('Ctrl Pts',(0.197750601279868,0.13098169794209,-1.71641072955723));
#67214=CARTESIAN_POINT('Ctrl Pts',(0.209265050054842,0.113096472569572,
-1.71787540546711));
#67215=CARTESIAN_POINT('Ctrl Pts',(0.217315911428638,0.0967275721864568,
-1.71919380376489));
#67216=CARTESIAN_POINT('Ctrl Pts',(0.224703613739888,0.0759931480312389,
-1.72080140268741));
#67217=CARTESIAN_POINT('Ctrl Pts',(0.225902395432838,0.0723517861603751,
-1.72108123755319));
#67218=CARTESIAN_POINT('Ctrl Pts',(0.22890707679145,0.062420644573984,-1.72183571978181));
#67219=CARTESIAN_POINT('Ctrl Pts',(0.230541939000404,0.0560821948155643,
-1.722308000844));
#67220=CARTESIAN_POINT('Ctrl Pts',(0.232680118736906,0.0461016705786794,
-1.72303019545722));
#67221=CARTESIAN_POINT('Ctrl Pts',(0.233364503638271,0.0425019267676532,
-1.72328638315693));
#67222=CARTESIAN_POINT('Ctrl Pts',(0.234147987313098,0.0377881297580144,
-1.7236150763283));
#67223=CARTESIAN_POINT('Ctrl Pts',(0.234322973746065,0.0366874203474679,
-1.72369134931222));
#67224=CARTESIAN_POINT('Ctrl Pts',(0.234595933156294,0.0348887573497782,
-1.7238151602851));
#67225=CARTESIAN_POINT('Ctrl Pts',(0.234698563262774,0.0341915439605781,
-1.72386295081084));
#67226=CARTESIAN_POINT('Ctrl Pts',(0.234892989785021,0.0328285789570707,
-1.72395596701296));
#67227=CARTESIAN_POINT('Ctrl Pts',(0.234985066351809,0.0321628800839689,
-1.72400120706889));
#67228=CARTESIAN_POINT('Ctrl Pts',(0.2351849536989,0.0306710335112133,-1.72410218147261));
#67229=CARTESIAN_POINT('Ctrl Pts',(0.235291244461667,0.029844682521119,
-1.72415783157489));
#67230=CARTESIAN_POINT('Ctrl Pts',(0.235646596284867,0.0269620562251806,
-1.72435103620877));
#67231=CARTESIAN_POINT('Ctrl Pts',(0.235873082488558,0.0249030217145075,
-1.72448740348092));
#67232=CARTESIAN_POINT('Ctrl Pts',(0.237243400767329,0.0107402556632508,
-1.72541579262485));
#67233=CARTESIAN_POINT('Ctrl Pts',(0.237482216190972,-0.00143444589990504,
-1.72616635489699));
#67234=CARTESIAN_POINT('Ctrl Pts',(0.236165921497674,-0.0243941535462405,
-1.72757792863405));
#67235=CARTESIAN_POINT('Ctrl Pts',(0.234804889310994,-0.0351578066973479,
-1.72823822039477));
#67236=CARTESIAN_POINT('Ctrl Pts',(0.230956442517926,-0.0547161584103204,
-1.72948114300453));
#67237=CARTESIAN_POINT('Ctrl Pts',(0.228688240202105,-0.0635326375192434,
-1.73005806201125));
#67238=CARTESIAN_POINT('Ctrl Pts',(0.225255000034431,-0.0742760535111648,
-1.7307938814289));
#67239=CARTESIAN_POINT('Ctrl Pts',(0.224561753873381,-0.0763463511906751,
-1.7309372049059));
#67240=CARTESIAN_POINT('Ctrl Pts',(0.223408263412331,-0.0796394022090826,
-1.73116777260335));
#67241=CARTESIAN_POINT('Ctrl Pts',(0.222966314661338,-0.0808684670041031,
-1.73125441093155));
#67242=CARTESIAN_POINT('Ctrl Pts',(0.22210838839416,-0.0831938657442761,
-1.73141947213356));
#67243=CARTESIAN_POINT('Ctrl Pts',(0.221694386716202,-0.0842908910017697,
-1.73149782705979));
#67244=CARTESIAN_POINT('Ctrl Pts',(0.220732611810652,-0.0867833036889839,
-1.73167698037627));
#67245=CARTESIAN_POINT('Ctrl Pts',(0.220179714255993,-0.0881766463774786,
-1.73177794833478));
#67246=CARTESIAN_POINT('Ctrl Pts',(0.218433919496877,-0.0924573583499218,
-1.7320907245545));
#67247=CARTESIAN_POINT('Ctrl Pts',(0.217197195243552,-0.0953263712460283,
-1.73230400035997));
#67248=CARTESIAN_POINT('Ctrl Pts',(0.20859527678713,-0.114244476112031,
-1.73373544800115));
#67249=CARTESIAN_POINT('Ctrl Pts',(0.199515363056517,-0.129449543973588,
-1.73501384883128));
#67250=CARTESIAN_POINT('Ctrl Pts',(0.18617075548076,-0.147009596010536,
-1.73662469551224));
#67251=CARTESIAN_POINT('Ctrl Pts',(0.183409241612209,-0.150440760732392,
-1.73694632552688));
#67252=CARTESIAN_POINT('Ctrl Pts',(0.176357577589377,-0.158719446032334,
-1.73773692262608));
#67253=CARTESIAN_POINT('Ctrl Pts',(0.171961217468533,-0.163472348417104,
-1.73820389321613));
#67254=CARTESIAN_POINT('Ctrl Pts',(0.164798755024177,-0.170606505449436,
-1.73891902690364));
#67255=CARTESIAN_POINT('Ctrl Pts',(0.16216294631855,-0.173113811638388,
-1.73917333160133));
#67256=CARTESIAN_POINT('Ctrl Pts',(0.158647475233605,-0.176307104233043,
-1.73950000006214));
#67257=CARTESIAN_POINT('Ctrl Pts',(0.15781935031295,-0.177048776303312,
-1.7395760757885));
#67258=CARTESIAN_POINT('Ctrl Pts',(0.156458242560708,-0.178250651326304,
-1.73969964766496));
#67259=CARTESIAN_POINT('Ctrl Pts',(0.155928382766988,-0.1787143414619,-1.73974739456614));
#67260=CARTESIAN_POINT('Ctrl Pts',(0.154888451314804,-0.179616258897454,
-1.73984039468729));
#67261=CARTESIAN_POINT('Ctrl Pts',(0.154378569645772,-0.180054686311474,
-1.73988566181945));
#67262=CARTESIAN_POINT('Ctrl Pts',(0.153231599626905,-0.181032467417762,
-1.73998676777583));
#67263=CARTESIAN_POINT('Ctrl Pts',(0.152593508203342,-0.181570643800616,
-1.74004252163597));
#67264=CARTESIAN_POINT('Ctrl Pts',(0.150355094085289,-0.183438423116216,
-1.74023644139134));
#67265=CARTESIAN_POINT('Ctrl Pts',(0.148740073448511,-0.184750373934941,
-1.74037340847613));
#67266=CARTESIAN_POINT('Ctrl Pts',(0.137683673381442,-0.193492987199117,
-1.74129297067195));
#67267=CARTESIAN_POINT('Ctrl Pts',(0.12770551808618,-0.200219141713083,
-1.74203515444148));
#67268=CARTESIAN_POINT('Ctrl Pts',(0.108028799506185,-0.211410800821003,
-1.74342484008459));
#67269=CARTESIAN_POINT('Ctrl Pts',(0.0984561547738076,-0.216035009790264,
-1.74407180825317));
#67270=CARTESIAN_POINT('Ctrl Pts',(0.0798805286347172,-0.223516373858651,
-1.7453188648375));
#67271=CARTESIAN_POINT('Ctrl Pts',(0.0709544612949117,-0.226508059428522,
-1.7459146797503));
#67272=CARTESIAN_POINT('Ctrl Pts',(0.0597483949223565,-0.229536408680303,
-1.74667182614111));
#67273=CARTESIAN_POINT('Ctrl Pts',(0.0576138916008783,-0.230081447673283,
-1.74681641980918));
#67274=CARTESIAN_POINT('Ctrl Pts',(0.0541981200994316,-0.230903143159002,
-1.74704854842856));
#67275=CARTESIAN_POINT('Ctrl Pts',(0.0529215809786821,-0.231199056859538,
-1.74713546270623));
#67276=CARTESIAN_POINT('Ctrl Pts',(0.0504990685385622,-0.23173950382593,
-1.747300740945));
#67277=CARTESIAN_POINT('Ctrl Pts',(0.0493536035275094,-0.231986153230337,
-1.74737903436004));
#67278=CARTESIAN_POINT('Ctrl Pts',(0.0467459466916553,-0.232527464728643,
-1.7475576167204));
#67279=CARTESIAN_POINT('Ctrl Pts',(0.0452827204979859,-0.232816838807933,
-1.74765807122044));
#67280=CARTESIAN_POINT('Ctrl Pts',(0.0407852696601377,-0.23366227316649,
-1.74796764248087));
#67281=CARTESIAN_POINT('Ctrl Pts',(0.0377429505312559,-0.234172936618899,
-1.7481781835874));
#67282=CARTESIAN_POINT('Ctrl Pts',(0.0166808833046302,-0.237287186318497,
-1.74964420480863));
#67283=CARTESIAN_POINT('Ctrl Pts',(-0.00157338997851186,-0.237867062825944,
-1.75096424667569));
#67284=CARTESIAN_POINT('Ctrl Pts',(-0.0235085183083695,-0.236037829829799,
-1.75257184277125));
#67285=CARTESIAN_POINT('Ctrl Pts',(-0.0272986087407516,-0.235629569757196,
-1.75285009644845));
#67286=CARTESIAN_POINT('Ctrl Pts',(-0.0375653165665592,-0.234272614653689,
-1.75360314816787));
#67287=CARTESIAN_POINT('Ctrl Pts',(-0.0440155664850886,-0.233146847368946,
-1.75407556739695));
#67288=CARTESIAN_POINT('Ctrl Pts',(-0.0539918152787328,-0.230976818269961,
-1.75479794558265));
#67289=CARTESIAN_POINT('Ctrl Pts',(-0.0575539720588981,-0.23011508131599,
-1.75505418213814));
#67290=CARTESIAN_POINT('Ctrl Pts',(-0.0621719113940535,-0.228883980025758,
-1.75538292788393));
#67291=CARTESIAN_POINT('Ctrl Pts',(-0.06324685253013,-0.22858927937995,
-1.75545920602704));
#67292=CARTESIAN_POINT('Ctrl Pts',(-0.0649980215446012,-0.228095888744375,
-1.7555830232952));
#67293=CARTESIAN_POINT('Ctrl Pts',(-0.0656754966235909,-0.227901747345606,
-1.7556308150032));
#67294=CARTESIAN_POINT('Ctrl Pts',(-0.0669973014848966,-0.227516579265103,
-1.75572383242033));
#67295=CARTESIAN_POINT('Ctrl Pts',(-0.0676416988422023,-0.227325829684345,
-1.75576907251866));
#67296=CARTESIAN_POINT('Ctrl Pts',(-0.0690831201836953,-0.226892479399009,
-1.75587004536072));
#67297=CARTESIAN_POINT('Ctrl Pts',(-0.0698797023615972,-0.22664841043365,
-1.75592569387407));
#67298=CARTESIAN_POINT('Ctrl Pts',(-0.0726520013762823,-0.225782985968168,
-1.75611888487856));
#67299=CARTESIAN_POINT('Ctrl Pts',(-0.07462092007861,-0.225139932174956,
-1.75625524036277));
#67300=CARTESIAN_POINT('Ctrl Pts',(-0.0880914363734373,-0.220544290708814,
-1.75718389130812));
#67301=CARTESIAN_POINT('Ctrl Pts',(-0.0992841077765119,-0.215737404444969,
-1.75793469780409));
#67302=CARTESIAN_POINT('Ctrl Pts',(-0.119664298256086,-0.205060963001253,
-1.75934687839085));
#67303=CARTESIAN_POINT('Ctrl Pts',(-0.128912331858323,-0.199376888551832,
-1.7600075276878));
#67304=CARTESIAN_POINT('Ctrl Pts',(-0.145137197186066,-0.187802469106299,
-1.76125030218137));
#67305=CARTESIAN_POINT('Ctrl Pts',(-0.152225389661359,-0.182104297397841,
-1.76182667453311));
#67306=CARTESIAN_POINT('Ctrl Pts',(-0.160588518911486,-0.174551059218529,
-1.76256187751194));
#67307=CARTESIAN_POINT('Ctrl Pts',(-0.162188020554886,-0.173065854941128,
-1.76270516437074));
#67308=CARTESIAN_POINT('Ctrl Pts',(-0.164711436459337,-0.170657050688398,
-1.76293568778416));
#67309=CARTESIAN_POINT('Ctrl Pts',(-0.165648638202693,-0.169747503062354,
-1.76302231888555));
#67310=CARTESIAN_POINT('Ctrl Pts',(-0.167412958574379,-0.16800671680448,
-1.7631873757744));
#67311=CARTESIAN_POINT('Ctrl Pts',(-0.168241520312579,-0.167176991083608,
-1.76326573369276));
#67312=CARTESIAN_POINT('Ctrl Pts',(-0.170115393927684,-0.165272445428651,
-1.76344490714452));
#67313=CARTESIAN_POINT('Ctrl Pts',(-0.171156726207246,-0.164193798187904,
-1.76354589237277));
#67314=CARTESIAN_POINT('Ctrl Pts',(-0.174337022194409,-0.160836410402298,
-1.7638587726081));
#67315=CARTESIAN_POINT('Ctrl Pts',(-0.176441150621054,-0.158525288080713,
-1.76407213653543));
#67316=CARTESIAN_POINT('Ctrl Pts',(-0.190112922887156,-0.142899085607667,
-1.76550228622493));
#67317=CARTESIAN_POINT('Ctrl Pts',(-0.200207881602859,-0.128373095693726,
-1.7667791435396));
#67318=CARTESIAN_POINT('Ctrl Pts',(-0.215170485425602,-0.100719313762183,
-1.76907557861254));
#67319=CARTESIAN_POINT('Ctrl Pts',(-0.220669930043714,-0.0880203631203799,
-1.77008477857942));
#67320=CARTESIAN_POINT('Ctrl Pts',(-0.225510372989238,-0.0734801681962261,
-1.77114563972998));
#67321=CARTESIAN_POINT('Ctrl Pts',(-0.225973909804841,-0.0720420420888783,
-1.7712495583202));
#67322=CARTESIAN_POINT('Ctrl Pts',(-0.226659024856208,-0.0698447716957313,
-1.77140669931785));
#67323=CARTESIAN_POINT('Ctrl Pts',(-0.226890592173997,-0.069088819000598,
-1.77146046971265));
#67324=CARTESIAN_POINT('Ctrl Pts',(-0.227307210202494,-0.0677040795699109,
-1.77155841286855));
#67325=CARTESIAN_POINT('Ctrl Pts',(-0.227493436001042,-0.0670756796399827,
-1.77160265079527));
#67326=CARTESIAN_POINT('Ctrl Pts',(-0.227908576823507,-0.0656532110891207,
-1.77170232194437));
#67327=CARTESIAN_POINT('Ctrl Pts',(-0.228135948525569,-0.0648587122766279,
-1.77175766585196));
#67328=CARTESIAN_POINT('Ctrl Pts',(-0.228714589309954,-0.0627960883985072,
-1.77190054151389));
#67329=CARTESIAN_POINT('Ctrl Pts',(-0.229059471619472,-0.0615261792727594,
-1.77198772113345));
#67330=CARTESIAN_POINT('Ctrl Pts',(-0.23143881793859,-0.0524676537366121,
-1.77260444783947));
#67331=CARTESIAN_POINT('Ctrl Pts',(-0.23308639318249,-0.0445818818422,-1.77311441502904));
#67332=CARTESIAN_POINT('Ctrl Pts',(-0.23621322905722,-0.0245770790752242,
-1.77437552441747));
#67333=CARTESIAN_POINT('Ctrl Pts',(-0.23716447290241,-0.0123997790984111,
-1.77511444457095));
#67334=CARTESIAN_POINT('Ctrl Pts',(-0.237185568223226,0.0122448055089872,
-1.77663336339897));
#67335=CARTESIAN_POINT('Ctrl Pts',(-0.23621628787675,0.0246725294036408,
-1.77741178370879));
#67336=CARTESIAN_POINT('Ctrl Pts',(-0.233905237174039,0.0393191648082009,
-1.7783768335306));
#67337=CARTESIAN_POINT('Ctrl Pts',(-0.233498484371059,0.04166669918446,
-1.77853294004969));
#67338=CARTESIAN_POINT('Ctrl Pts',(-0.23280351116214,0.0453471507595598,
-1.77878012319147));
#67339=CARTESIAN_POINT('Ctrl Pts',(-0.232539034570062,0.0466844316802177,
-1.77887044559743));
#67340=CARTESIAN_POINT('Ctrl Pts',(-0.232029243591978,0.0491502219033092,
-1.77903796573602));
#67341=CARTESIAN_POINT('Ctrl Pts',(-0.231787185207946,0.0502793684045034,
-1.77911505726072));
#67342=CARTESIAN_POINT('Ctrl Pts',(-0.231230920573847,0.0527847971283286,
-1.77928698041455));
#67343=CARTESIAN_POINT('Ctrl Pts',(-0.230912655210498,0.0541601232552643,
-1.77938193974669));
#67344=CARTESIAN_POINT('Ctrl Pts',(-0.22995441073413,0.0581389474750131,
-1.77965839727738));
#67345=CARTESIAN_POINT('Ctrl Pts',(-0.229282559096718,0.0607344654645677,
-1.77984091131453));
#67346=CARTESIAN_POINT('Ctrl Pts',(-0.224633657572367,0.0775161988928925,
-1.78103560412374));
#67347=CARTESIAN_POINT('Ctrl Pts',(-0.219386770959641,0.0913145314764611,
-1.78208922235472));
#67348=CARTESIAN_POINT('Ctrl Pts',(-0.205729670451209,0.119128510280837,
-1.78434498511081));
#67349=CARTESIAN_POINT('Ctrl Pts',(-0.197082115277084,0.132947378184802,
-1.78554542520255));
#67350=CARTESIAN_POINT('Ctrl Pts',(-0.185714337261873,0.147536989754321,
-1.78683792526994));
#67351=CARTESIAN_POINT('Ctrl Pts',(-0.184315372054303,0.149281020029628,
-1.78699281630458));
#67352=CARTESIAN_POINT('Ctrl Pts',(-0.182344510676915,0.15166805599514,
-1.78720505791824));
#67353=CARTESIAN_POINT('Ctrl Pts',(-0.18179351604347,0.152328058365742,
-1.78726376782028));
#67354=CARTESIAN_POINT('Ctrl Pts',(-0.180840297133733,0.153457321419483,
-1.78736424418783));
#67355=CARTESIAN_POINT('Ctrl Pts',(-0.180439810021333,0.153928027163815,
-1.78740613249747));
#67356=CARTESIAN_POINT('Ctrl Pts',(-0.179593808938075,0.154914521317799,
-1.78749392633291));
#67357=CARTESIAN_POINT('Ctrl Pts',(-0.17914790395882,0.155429963811847,
-1.7875398007564));
#67358=CARTESIAN_POINT('Ctrl Pts',(-0.178038145931827,0.156701665006331,
-1.78765300833025));
#67359=CARTESIAN_POINT('Ctrl Pts',(-0.17737168015547,0.157455645794402,
-1.78772015129858));
#67360=CARTESIAN_POINT('Ctrl Pts',(-0.174849169802852,0.16027305089246,
-1.78797123527754));
#67361=CARTESIAN_POINT('Ctrl Pts',(-0.172961669040362,0.162308181298798,
-1.78815299169916));
#67362=CARTESIAN_POINT('Ctrl Pts',(-0.168011491502528,0.167461082939212,
-1.78861568277769));
#67363=CARTESIAN_POINT('Ctrl Pts',(-0.164897501630042,0.17052827977056,
-1.78889353457784));
#67364=CARTESIAN_POINT('Ctrl Pts',(-0.154703488025146,0.180028573636075,
-1.78976911452611));
#67365=CARTESIAN_POINT('Ctrl Pts',(-0.147318219221917,0.18612044022142,
-1.79035396772996));
#67366=CARTESIAN_POINT('Ctrl Pts',(-0.127006269313363,0.200906581356134,
-1.79189371948727));
#67367=CARTESIAN_POINT('Ctrl Pts',(-0.113558782386345,0.208802232665008,
-1.79284936163473));
#67368=CARTESIAN_POINT('Ctrl Pts',(-0.0965644993398727,0.21665013677787,
-1.79405877030531));
#67369=CARTESIAN_POINT('Ctrl Pts',(-0.0936669139367885,0.217918544403896,
-1.79426489998666));
#67370=CARTESIAN_POINT('Ctrl Pts',(-0.0893479764318352,0.219707091159926,
-1.79457246989879));
#67371=CARTESIAN_POINT('Ctrl Pts',(-0.0879455419069915,0.22027221404261,
-1.794672392306));
#67372=CARTESIAN_POINT('Ctrl Pts',(-0.0854416054859059,0.221253472128248,
-1.79485092986333));
#67373=CARTESIAN_POINT('Ctrl Pts',(-0.0843422179254959,0.2216748904736,
-1.7949293646418));
#67374=CARTESIAN_POINT('Ctrl Pts',(-0.0820354495447255,0.22253947905544,
-1.7950940561207));
#67375=CARTESIAN_POINT('Ctrl Pts',(-0.0808275136238489,0.222981047734035,
-1.79518036328306));
#67376=CARTESIAN_POINT('Ctrl Pts',(-0.0776461585768175,0.224114765305109,
-1.79540787742805));
#67377=CARTESIAN_POINT('Ctrl Pts',(-0.0756671093598199,0.224790662710331,
-1.79554961641383));
#67378=CARTESIAN_POINT('Ctrl Pts',(-0.0662339549736757,0.227873649818092,
-1.79622638152544));
#67379=CARTESIAN_POINT('Ctrl Pts',(-0.0586733271183367,0.229936411793327,
-1.7967724699271));
#67380=CARTESIAN_POINT('Ctrl Pts',(-0.0480073595660445,0.232286081287475,
-1.79754805523746));
#67381=CARTESIAN_POINT('Ctrl Pts',(-0.0449781099096792,0.23289156918018,
-1.7977688709484));
#67382=CARTESIAN_POINT('Ctrl Pts',(-0.0419392500630493,0.233437528964708,
-1.79799080372057));
#67383=CARTESIAN_POINT('Ctrl Pts',(-0.0419392741328096,0.233437524640348,
-1.81760526556689));
#67384=CARTESIAN_POINT('Ctrl Pts',(-0.0422246088831205,0.233386261535449,
-1.81758570663374));
#67385=CARTESIAN_POINT('Ctrl Pts',(-0.0425098517635914,0.2333344748991,
-1.81756617774455));
#67386=CARTESIAN_POINT('Ctrl Pts',(-0.0436093707511774,0.233132771009703,
-1.81749098927691));
#67387=CARTESIAN_POINT('Ctrl Pts',(-0.0444229647295536,0.232979111494353,
-1.81743554172198));
#67388=CARTESIAN_POINT('Ctrl Pts',(-0.0465328294537987,0.232569177508753,
-1.81729220175974));
#67389=CARTESIAN_POINT('Ctrl Pts',(-0.0478278138186597,0.232306321405142,
-1.81720466527269));
#67390=CARTESIAN_POINT('Ctrl Pts',(-0.0571309294967675,0.230336881567906,
-1.81657854849105));
#67391=CARTESIAN_POINT('Ctrl Pts',(-0.065049066315338,0.228227237965445,
-1.81606022297569));
#67392=CARTESIAN_POINT('Ctrl Pts',(-0.0771927254296154,0.224308167962868,
-1.81526595629149));
#67393=CARTESIAN_POINT('Ctrl Pts',(-0.0815010573453379,0.222778928322139,
-1.81498431454518));
#67394=CARTESIAN_POINT('Ctrl Pts',(-0.0950381294844814,0.217528645486334,
-1.81409257352345));
#67395=CARTESIAN_POINT('Ctrl Pts',(-0.104077907003057,0.213351217043882,
-1.81348642716782));
#67396=CARTESIAN_POINT('Ctrl Pts',(-0.121850003482557,0.203739416455373,
-1.81223233037505));
#67397=CARTESIAN_POINT('Ctrl Pts',(-0.130544431266464,0.198280824566761,
-1.81158491863131));
#67398=CARTESIAN_POINT('Ctrl Pts',(-0.14068290626407,0.190959078011664,
-1.81076963332027));
#67399=CARTESIAN_POINT('Ctrl Pts',(-0.142489225026791,0.18961505681025,
-1.81062191479122));
#67400=CARTESIAN_POINT('Ctrl Pts',(-0.145324276518914,0.187442202734499,
-1.81038596330318));
#67401=CARTESIAN_POINT('Ctrl Pts',(-0.146365719574649,0.186630117412527,
-1.81029838810508));
#67402=CARTESIAN_POINT('Ctrl Pts',(-0.148316578219735,0.185082525197438,
-1.81013260170882));
#67403=CARTESIAN_POINT('Ctrl Pts',(-0.149227444295666,0.184348903692869,
-1.81005446738617));
#67404=CARTESIAN_POINT('Ctrl Pts',(-0.151273570910773,0.182675829509065,
-1.80987727330228));
#67405=CARTESIAN_POINT('Ctrl Pts',(-0.152405568141666,0.181732480783426,
-1.80977805751174));
#67406=CARTESIAN_POINT('Ctrl Pts',(-0.155734271168668,0.178905535548853,
-1.80948271973171));
#67407=CARTESIAN_POINT('Ctrl Pts',(-0.157905308812134,0.176992276735527,
-1.80928538607277));
#67408=CARTESIAN_POINT('Ctrl Pts',(-0.174578663431968,0.161747658586013,
-1.80773189184986));
#67409=CARTESIAN_POINT('Ctrl Pts',(-0.187401353991968,0.146698463779471,
-1.80629828075995));
#67410=CARTESIAN_POINT('Ctrl Pts',(-0.204857522272324,0.12013211026744,
-1.80397793463329));
#67411=CARTESIAN_POINT('Ctrl Pts',(-0.210718257825865,0.109527225876218,
-1.80309928727604));
#67412=CARTESIAN_POINT('Ctrl Pts',(-0.216364772566557,0.0971622087771301,
-1.80215852130915));
#67413=CARTESIAN_POINT('Ctrl Pts',(-0.216972126623969,0.0957982576953321,
-1.80205585457936));
#67414=CARTESIAN_POINT('Ctrl Pts',(-0.217879783902641,0.0937069860932872,
-1.80190022303876));
#67415=CARTESIAN_POINT('Ctrl Pts',(-0.218189401797958,0.0929837860302456,
-1.80184672541694));
#67416=CARTESIAN_POINT('Ctrl Pts',(-0.218750332982474,0.0916553428999317,
-1.80174906368497));
#67417=CARTESIAN_POINT('Ctrl Pts',(-0.219002737651016,0.0910505957403779,
-1.80170483656576));
#67418=CARTESIAN_POINT('Ctrl Pts',(-0.219569234752227,0.0896773160588872,
-1.80160492273518));
#67419=CARTESIAN_POINT('Ctrl Pts',(-0.219881800926178,0.0889081747601063,
-1.80154932763591));
#67420=CARTESIAN_POINT('Ctrl Pts',(-0.220684310991653,0.0869032941126098,
-1.80140531633062));
#67421=CARTESIAN_POINT('Ctrl Pts',(-0.221167924145811,0.0856650288820689,
-1.80131726185175));
#67422=CARTESIAN_POINT('Ctrl Pts',(-0.2247401280476,0.0762866627949354,
-1.8006565807432));
#67423=CARTESIAN_POINT('Ctrl Pts',(-0.227389185159766,0.0679851086415468,
-1.80010691500392));
#67424=CARTESIAN_POINT('Ctrl Pts',(-0.230600643256581,0.0556055575569116,
-1.79931263554828));
#67425=CARTESIAN_POINT('Ctrl Pts',(-0.23152328552715,0.0516294916798794,
-1.79906128675766));
#67426=CARTESIAN_POINT('Ctrl Pts',(-0.233924859197877,0.039914800132482,
-1.79832692217921));
#67427=CARTESIAN_POINT('Ctrl Pts',(-0.23512139376539,0.0321241326543517,
-1.79784622100817));
#67428=CARTESIAN_POINT('Ctrl Pts',(-0.236754954501028,0.0162563737886748,
-1.79686202282117));
#67429=CARTESIAN_POINT('Ctrl Pts',(-0.237171079224004,0.00818791057595655,
-1.79635888636619));
#67430=CARTESIAN_POINT('Ctrl Pts',(-0.237177386889776,-0.00489263773771135,
-1.79552559647331));
#67431=CARTESIAN_POINT('Ctrl Pts',(-0.237021247212718,-0.00989815163286558,
-1.79520260220827));
#67432=CARTESIAN_POINT('Ctrl Pts',(-0.236590546774835,-0.0167428478078149,
-1.79475343268494));
#67433=CARTESIAN_POINT('Ctrl Pts',(-0.236452615215791,-0.0185895188412432,
-1.79463150321382));
#67434=CARTESIAN_POINT('Ctrl Pts',(-0.236197354986612,-0.0215412274122031,
-1.7944353358585));
#67435=CARTESIAN_POINT('Ctrl Pts',(-0.236093857948845,-0.0226474093072384,
-1.79436153300627));
#67436=CARTESIAN_POINT('Ctrl Pts',(-0.235863988168266,-0.0249311506058672,
-1.79420855168445));
#67437=CARTESIAN_POINT('Ctrl Pts',(-0.235736559883318,-0.0261085700804269,
-1.7941293420643));
#67438=CARTESIAN_POINT('Ctrl Pts',(-0.235417678729328,-0.028862046031564,
-1.79394329057562));
#67439=CARTESIAN_POINT('Ctrl Pts',(-0.235219210106757,-0.030437216405649,
-1.79383623077473));
#67440=CARTESIAN_POINT('Ctrl Pts',(-0.234516717286978,-0.0355946058332425,
-1.79348357812263));
#67441=CARTESIAN_POINT('Ctrl Pts',(-0.233946572451736,-0.0391671466644057,
-1.79323592371365));
#67442=CARTESIAN_POINT('Ctrl Pts',(-0.230898611526427,-0.0558101549525806,
-1.79206575504119));
#67443=CARTESIAN_POINT('Ctrl Pts',(-0.227406010435155,-0.0686683945522261,
-1.79111202140262));
#67444=CARTESIAN_POINT('Ctrl Pts',(-0.217275742243629,-0.0964833165233793,
-1.78895691567429));
#67445=CARTESIAN_POINT('Ctrl Pts',(-0.210131617289113,-0.111187002642677,
-1.78775308456659));
#67446=CARTESIAN_POINT('Ctrl Pts',(-0.200379833773667,-0.126904314738665,
-1.78646109942568));
#67447=CARTESIAN_POINT('Ctrl Pts',(-0.199198687516331,-0.12875040438966,
-1.78630932166144));
#67448=CARTESIAN_POINT('Ctrl Pts',(-0.197522433954854,-0.131292026948759,
-1.78610060423131));
#67449=CARTESIAN_POINT('Ctrl Pts',(-0.197048948808188,-0.132001591223906,
-1.78604236193242));
#67450=CARTESIAN_POINT('Ctrl Pts',(-0.196226903881339,-0.133219226838685,
-1.7859424838881));
#67451=CARTESIAN_POINT('Ctrl Pts',(-0.19588017767724,-0.13372851686052,
-1.78590072932225));
#67452=CARTESIAN_POINT('Ctrl Pts',(-0.195144865043252,-0.134799587714983,
-1.7858129699912));
#67453=CARTESIAN_POINT('Ctrl Pts',(-0.194755829118427,-0.135361051439229,
-1.78576699771368));
#67454=CARTESIAN_POINT('Ctrl Pts',(-0.193782994837488,-0.136752187116081,
-1.78565315086778));
#67455=CARTESIAN_POINT('Ctrl Pts',(-0.193196280224435,-0.137579821085454,
-1.78558547142583));
#67456=CARTESIAN_POINT('Ctrl Pts',(-0.190949105303398,-0.140707017207383,
-1.78532983774709));
#67457=CARTESIAN_POINT('Ctrl Pts',(-0.189252674920491,-0.142980601124255,
-1.78514417188698));
#67458=CARTESIAN_POINT('Ctrl Pts',(-0.184757083241285,-0.148785414851225,
-1.78466905294354));
#67459=CARTESIAN_POINT('Ctrl Pts',(-0.181897276319982,-0.152268399185218,
-1.78438289534952));
#67460=CARTESIAN_POINT('Ctrl Pts',(-0.164516480140254,-0.172247562214298,
-1.78272089550249));
#67461=CARTESIAN_POINT('Ctrl Pts',(-0.14785921584081,-0.186742164664861,
-1.78141946274587));
#67462=CARTESIAN_POINT('Ctrl Pts',(-0.125040611242471,-0.201604657202883,
-1.77968747851324));
#67463=CARTESIAN_POINT('Ctrl Pts',(-0.120543741007083,-0.204325211901945,
-1.77934891109686));
#67464=CARTESIAN_POINT('Ctrl Pts',(-0.114314767229415,-0.207816442661382,
-1.778881445741));
#67465=CARTESIAN_POINT('Ctrl Pts',(-0.112658138334739,-0.208719149512561,
-1.77875726695489));
#67466=CARTESIAN_POINT('Ctrl Pts',(-0.110003152677722,-0.210125049401805,
-1.77855839635612));
#67467=CARTESIAN_POINT('Ctrl Pts',(-0.109011679168349,-0.210641125417597,
-1.77848416211732));
#67468=CARTESIAN_POINT('Ctrl Pts',(-0.106965108404931,-0.211688075262727,
-1.77833097477434));
#67469=CARTESIAN_POINT('Ctrl Pts',(-0.105909621131383,-0.212218113480382,
-1.77825199499501));
#67470=CARTESIAN_POINT('Ctrl Pts',(-0.103445951142906,-0.213432347235163,
-1.77806767684125));
#67471=CARTESIAN_POINT('Ctrl Pts',(-0.102034878831108,-0.21411052041243,
-1.7779621327569));
#67472=CARTESIAN_POINT('Ctrl Pts',(-0.0974570899010838,-0.216255114275751,
-1.77761974459099));
#67473=CARTESIAN_POINT('Ctrl Pts',(-0.0942648210789319,-0.217665569332193,
-1.77738100229604));
#67474=CARTESIAN_POINT('Ctrl Pts',(-0.0866275748507787,-0.220840454617206,
-1.77680957544679));
#67475=CARTESIAN_POINT('Ctrl Pts',(-0.082158197746704,-0.222541834829099,
-1.77647495527151));
#67476=CARTESIAN_POINT('Ctrl Pts',(-0.0641865043012014,-0.228768038151814,
-1.77512873507427));
#67477=CARTESIAN_POINT('Ctrl Pts',(-0.0503411202545978,-0.232207692042918,
-1.77408777640383));
#67478=CARTESIAN_POINT('Ctrl Pts',(-0.0245155959738507,-0.236204374912188,
-1.7721806180759));
#67479=CARTESIAN_POINT('Ctrl Pts',(-0.0126367752292691,-0.237136880421377,
-1.77131716988441));
#67480=CARTESIAN_POINT('Ctrl Pts',(0.000607927362936147,-0.23717803381994,
-1.77040055003912));
#67481=CARTESIAN_POINT('Ctrl Pts',(0.0019528419942021,-0.237170773745787,
-1.77030801200717));
#67482=CARTESIAN_POINT('Ctrl Pts',(0.00413253994607958,-0.237140464487511,
-1.77015898623531));
#67483=CARTESIAN_POINT('Ctrl Pts',(0.00496736861772641,-0.237124446412701,
-1.77010213506341));
#67484=CARTESIAN_POINT('Ctrl Pts',(0.00645759485272556,-0.237087979471249,
-1.77000107592872));
#67485=CARTESIAN_POINT('Ctrl Pts',(0.00711300879699002,-0.23706922128587,
-1.76995677711602));
#67486=CARTESIAN_POINT('Ctrl Pts',(0.00855102537612164,-0.237022095612318,
-1.76985990877358));
#67487=CARTESIAN_POINT('Ctrl Pts',(0.00933357021466848,-0.236992570252592,
-1.7698074037868));
#67488=CARTESIAN_POINT('Ctrl Pts',(0.0115902197694559,-0.236896232152906,
-1.76965655972279));
#67489=CARTESIAN_POINT('Ctrl Pts',(0.0130638978233652,-0.236819536461065,
-1.76955874996291));
#67490=CARTESIAN_POINT('Ctrl Pts',(0.0253880638188002,-0.236062747086201,
-1.7687458952489));
#67491=CARTESIAN_POINT('Ctrl Pts',(0.0361822176882157,-0.234650987420839,
-1.76806687022452));
#67492=CARTESIAN_POINT('Ctrl Pts',(0.0641677279359495,-0.229012717023274,
-1.76630665030344));
#67493=CARTESIAN_POINT('Ctrl Pts',(0.0810472239583556,-0.223597048615859,
-1.7652412307388));
#67494=CARTESIAN_POINT('Ctrl Pts',(0.101881666506948,-0.21424005826287,
-1.76378779691733));
#67495=CARTESIAN_POINT('Ctrl Pts',(0.106524222243309,-0.211969951554247,
-1.7634547492042));
#67496=CARTESIAN_POINT('Ctrl Pts',(0.112744455486857,-0.208672423662257,
-1.76299378543093));
#67497=CARTESIAN_POINT('Ctrl Pts',(0.114389712856402,-0.207775084883823,
-1.76287041795289));
#67498=CARTESIAN_POINT('Ctrl Pts',(0.116996874383364,-0.206312762406059,
-1.76267252287729));
#67499=CARTESIAN_POINT('Ctrl Pts',(0.117965748248855,-0.205760313750698,
-1.76259844466805));
#67500=CARTESIAN_POINT('Ctrl Pts',(0.11995350227874,-0.204608248893662,
-1.76244533559134));
#67501=CARTESIAN_POINT('Ctrl Pts',(0.12097186595071,-0.204007808147772,
-1.76236627645481));
#67502=CARTESIAN_POINT('Ctrl Pts',(0.123334948920558,-0.202590587948241,
-1.76218135087122));
#67503=CARTESIAN_POINT('Ctrl Pts',(0.124676101048679,-0.201767999370211,
-1.76207527443289));
#67504=CARTESIAN_POINT('Ctrl Pts',(0.129003084550629,-0.199054453395888,
-1.76172930739334));
#67505=CARTESIAN_POINT('Ctrl Pts',(0.131954733542683,-0.197110165117121,
-1.76148746241492));
#67506=CARTESIAN_POINT('Ctrl Pts',(0.138861366757028,-0.192336014437533,
-1.76090717699937));
#67507=CARTESIAN_POINT('Ctrl Pts',(0.142774803680835,-0.189449126110858,
-1.76056671881602));
#67508=CARTESIAN_POINT('Ctrl Pts',(0.158172640118204,-0.177342180987372,
-1.75917937912675));
#67509=CARTESIAN_POINT('Ctrl Pts',(0.168874854955217,-0.167182622849758,
-1.75810107048424));
#67510=CARTESIAN_POINT('Ctrl Pts',(0.185967867689111,-0.14762944651732,
-1.75620694932065));
#67511=CARTESIAN_POINT('Ctrl Pts',(0.192759995940159,-0.138643951505345,
-1.75539243536873));
#67512=CARTESIAN_POINT('Ctrl Pts',(0.199627828742628,-0.128072434747595,
-1.75451983334028));
#67513=CARTESIAN_POINT('Ctrl Pts',(0.200356654481993,-0.126929231341742,
-1.7544265371124));
#67514=CARTESIAN_POINT('Ctrl Pts',(0.201520141280725,-0.125069243823416,
-1.75427654022832));
#67515=CARTESIAN_POINT('Ctrl Pts',(0.201960863228489,-0.124356314157022,
-1.75421946852363));
#67516=CARTESIAN_POINT('Ctrl Pts',(0.202739690084116,-0.123081390927575,
-1.75411817812442));
#67517=CARTESIAN_POINT('Ctrl Pts',(0.203079252506474,-0.122520316537109,
-1.75407386674992));
#67518=CARTESIAN_POINT('Ctrl Pts',(0.20381781772885,-0.121288445122501,
-1.75397715921445));
#67519=CARTESIAN_POINT('Ctrl Pts',(0.204215839445421,-0.120617082984172,
-1.75392482608115));
#67520=CARTESIAN_POINT('Ctrl Pts',(0.205350517866711,-0.11868144931886,
-1.75377497137765));
#67521=CARTESIAN_POINT('Ctrl Pts',(0.206078814572423,-0.117412282372357,
-1.75367796849171));
#67522=CARTESIAN_POINT('Ctrl Pts',(0.211806672943705,-0.107213117844503,
-1.75290774765169));
#67523=CARTESIAN_POINT('Ctrl Pts',(0.216235876158186,-0.0979735709636499,
-1.75226642380738));
#67524=CARTESIAN_POINT('Ctrl Pts',(0.226035850376233,-0.0735992866731304,
-1.75064355638263));
#67525=CARTESIAN_POINT('Ctrl Pts',(0.230492965113802,-0.0581553645011969,
-1.74967685505498));
#67526=CARTESIAN_POINT('Ctrl Pts',(0.234611094090271,-0.0354795756479239,
-1.74822626099026));
#67527=CARTESIAN_POINT('Ctrl Pts',(0.235557477819984,-0.0285276333323937,
-1.74777797783194));
#67528=CARTESIAN_POINT('Ctrl Pts',(0.236384563734877,-0.0194601885439522,
-1.74718336595542));
#67529=CARTESIAN_POINT('Ctrl Pts',(0.236547077462784,-0.0173735601452316,
-1.74704586721124));
#67530=CARTESIAN_POINT('Ctrl Pts',(0.23676484115846,-0.0140016025243686,
-1.74682247478272));
#67531=CARTESIAN_POINT('Ctrl Pts',(0.236837287666206,-0.0127174660279749,
-1.74673712124373));
#67532=CARTESIAN_POINT('Ctrl Pts',(0.236956012128841,-0.0102573793628458,
-1.74657304139895));
#67533=CARTESIAN_POINT('Ctrl Pts',(0.237003989296173,-0.00908154650503912,
-1.74649437083388));
#67534=CARTESIAN_POINT('Ctrl Pts',(0.237094413137359,-0.00637019798465789,
-1.74631237410626));
#67535=CARTESIAN_POINT('Ctrl Pts',(0.237130696359459,-0.00483454382221716,
-1.74620885822027));
#67536=CARTESIAN_POINT('Ctrl Pts',(0.237198310614449,2.64541996312906E-5,
-1.74587974756742));
#67537=CARTESIAN_POINT('Ctrl Pts',(0.237174621684088,0.00335203400002923,
-1.74565245432632));
#67538=CARTESIAN_POINT('Ctrl Pts',(0.2369547064943,0.0111619046549588,-1.74511338737453));
#67539=CARTESIAN_POINT('Ctrl Pts',(0.236701093387147,0.0156431745928053,
-1.74479996061432));
#67540=CARTESIAN_POINT('Ctrl Pts',(0.235250107450525,0.0326906265683364,
-1.74359196553677));
#67541=CARTESIAN_POINT('Ctrl Pts',(0.233177587168043,0.0451601412476616,
-1.74267434928164));
#67542=CARTESIAN_POINT('Ctrl Pts',(0.2269511790872,0.0701207250392759,-1.7407954941748));
#67543=CARTESIAN_POINT('Ctrl Pts',(0.222730122529124,0.0825536918064508,
-1.73983724189428));
#67544=CARTESIAN_POINT('Ctrl Pts',(0.216681234592023,0.0964648610074144,
-1.73877923678251));
#67545=CARTESIAN_POINT('Ctrl Pts',(0.215834915283595,0.0983438706615251,
-1.7386366754137));
#67546=CARTESIAN_POINT('Ctrl Pts',(0.214613000457316,0.100965001189892,
-1.73843853357414));
#67547=CARTESIAN_POINT('Ctrl Pts',(0.214257858322897,0.101716476687329,
-1.73838181106852));
#67548=CARTESIAN_POINT('Ctrl Pts',(0.21360873295855,0.103071531058045,-1.73827970324171));
#67549=CARTESIAN_POINT('Ctrl Pts',(0.213316123924634,0.103675757173621,
-1.73823423574815));
#67550=CARTESIAN_POINT('Ctrl Pts',(0.212710923698674,0.104912062061687,
-1.73814134598709));
#67551=CARTESIAN_POINT('Ctrl Pts',(0.212398073293054,0.105544001824988,
-1.73809394019016));
#67552=CARTESIAN_POINT('Ctrl Pts',(0.211582326536876,0.107173446332444,
-1.73797187517052));
#67553=CARTESIAN_POINT('Ctrl Pts',(0.211075185793868,0.108168824374664,
-1.73789747474233));
#67554=CARTESIAN_POINT('Ctrl Pts',(0.208862697158191,0.112436516503552,
-1.73757903537841));
#67555=CARTESIAN_POINT('Ctrl Pts',(0.207088041319392,0.115672569411573,
-1.73733897914664));
#67556=CARTESIAN_POINT('Ctrl Pts',(0.201922935750103,0.124590825931142,
-1.736677637795));
#67557=CARTESIAN_POINT('Ctrl Pts',(0.198369079184624,0.130174755778603,
-1.73626378564027));
#67558=CARTESIAN_POINT('Ctrl Pts',(0.193033220000682,0.137831541864277,
-1.73568620926313));
#67559=CARTESIAN_POINT('Ctrl Pts',(0.191442108753656,0.140033129471458,
-1.73551890247147));
#67560=CARTESIAN_POINT('Ctrl Pts',(0.178188503943821,0.157723640797833,
-1.73416049422983));
#67561=CARTESIAN_POINT('Ctrl Pts',(0.1647062533374,0.171754641608623,-1.73298659682459));
#67562=CARTESIAN_POINT('Ctrl Pts',(0.147366681848749,0.185859726015681,
-1.73153946368953));
#67563=CARTESIAN_POINT('Ctrl Pts',(0.145031142214995,0.187687887685678,
-1.73134586580446));
#67564=CARTESIAN_POINT('Ctrl Pts',(0.141488995430069,0.190354933909949,
-1.73105383595194));
#67565=CARTESIAN_POINT('Ctrl Pts',(0.14030781839386,0.191227227731517,-1.73095671196292));
#67566=CARTESIAN_POINT('Ctrl Pts',(0.138171812430985,0.192774214007054,
-1.73078149195571));
#67567=CARTESIAN_POINT('Ctrl Pts',(0.137219942716272,0.193452925988174,
-1.73070355451308));
#67568=CARTESIAN_POINT('Ctrl Pts',(0.135179492918029,0.194885192098844,
-1.73053677350147));
#67569=CARTESIAN_POINT('Ctrl Pts',(0.134089546961815,0.195636721187718,
-1.73044785613788));
#67570=CARTESIAN_POINT('Ctrl Pts',(0.131116572785768,0.19765010221744,-1.73020575110217));
#67571=CARTESIAN_POINT('Ctrl Pts',(0.129221695166951,0.198894121183745,
-1.73005190111323));
#67572=CARTESIAN_POINT('Ctrl Pts',(0.118408184374765,0.20577361584526,-1.72917623250012));
#67573=CARTESIAN_POINT('Ctrl Pts',(0.109140421937473,0.210835458194456,
-1.72843370813801));
#67574=CARTESIAN_POINT('Ctrl Pts',(0.0855207006109245,0.221760510941409,
-1.72656335808938));
#67575=CARTESIAN_POINT('Ctrl Pts',(0.0708724869390377,0.226866839570555,
-1.72542037123355));
#67576=CARTESIAN_POINT('Ctrl Pts',(0.0490219580523127,0.232159263702428,
-1.72379822044009));
#67577=CARTESIAN_POINT('Ctrl Pts',(0.0421415614799232,0.233506285169764,
-1.72329939002018));
#67578=CARTESIAN_POINT('Ctrl Pts',(0.0338275761943979,0.234754409094052,
-1.72271820866506));
#67579=CARTESIAN_POINT('Ctrl Pts',(0.0324423417790905,0.234949850388549,
-1.72262209023703));
#67580=CARTESIAN_POINT('Ctrl Pts',(0.0302867495638811,0.235234552274076,
-1.72247371153436));
#67581=CARTESIAN_POINT('Ctrl Pts',(0.0295175741385323,0.235332306841149,
-1.72242100142236));
#67582=CARTESIAN_POINT('Ctrl Pts',(0.0280964304667106,0.235505842786432,
-1.72232406493486));
#67583=CARTESIAN_POINT('Ctrl Pts',(0.0274446264459685,0.235582690129883,
-1.72227978236074));
#67584=CARTESIAN_POINT('Ctrl Pts',(0.0259529424472506,0.235752283864299,
-1.72217883750642));
#67585=CARTESIAN_POINT('Ctrl Pts',(0.0251128787018391,0.235843248678904,
-1.72212227503345));
#67586=CARTESIAN_POINT('Ctrl Pts',(0.0224970179996491,0.236112367103913,
-1.72194698558677));
#67587=CARTESIAN_POINT('Ctrl Pts',(0.0207196346509031,0.236274973133956,
-1.72182908534887));
#67588=CARTESIAN_POINT('Ctrl Pts',(0.0062656107358857,0.237432953073083,
-1.72087881991969));
#67589=CARTESIAN_POINT('Ctrl Pts',(-0.00647229680483934,0.237427598613414,
-1.72009394717104));
#67590=CARTESIAN_POINT('Ctrl Pts',(-0.0267963352841244,0.235781232699088,
-1.71884247966409));
#67591=CARTESIAN_POINT('Ctrl Pts',(-0.0344016266277004,0.234791736067342,
-1.7183744766436));
#67592=CARTESIAN_POINT('Ctrl Pts',(-0.0419393124730365,0.233437517752158,
-1.71790170279738));
#67593=CARTESIAN_POINT('Origin',(0.,0.,-2.1456589891905));
#67594=CARTESIAN_POINT('',(-0.0419392741218017,0.233437524642326,-1.59829545246927));
#67595=CARTESIAN_POINT('',(-0.0419392757399419,0.233437524351611,-1.61803181050061));
#67596=CARTESIAN_POINT('',(-0.0419392741328076,0.233437524640348,-2.1456589891905));
#67597=CARTESIAN_POINT('',(-0.237174999934351,-5.58036924603097E-6,-1.6761644476277));
#67598=CARTESIAN_POINT('Ctrl Pts',(-0.0419392741218017,0.233437524642326,
-1.59829545246927));
#67599=CARTESIAN_POINT('Ctrl Pts',(-0.0413949734322705,0.233535313444096,
-1.59833049339946));
#67600=CARTESIAN_POINT('Ctrl Pts',(-0.0408503180760221,0.233631200819013,
-1.59836547307769));
#67601=CARTESIAN_POINT('Ctrl Pts',(-0.0261237725611548,0.236170756412341,
-1.59930911111679));
#67602=CARTESIAN_POINT('Ctrl Pts',(-0.0117482039028465,0.237320697836993,
-1.6001779974016));
#67603=CARTESIAN_POINT('Ctrl Pts',(0.0155055078283608,0.237016889532454,
-1.60185623824416));
#67604=CARTESIAN_POINT('Ctrl Pts',(0.0283326117277322,0.235827531878034,
-1.60265931191078));
#67605=CARTESIAN_POINT('Ctrl Pts',(0.0433522038510075,0.233191498241831,
-1.60365171553424));
#67606=CARTESIAN_POINT('Ctrl Pts',(0.0456988912846523,0.232742989339567,
-1.60380824990311));
#67607=CARTESIAN_POINT('Ctrl Pts',(0.0493747370613882,0.23198271128988,
-1.60405596363868));
#67608=CARTESIAN_POINT('Ctrl Pts',(0.0507087042723419,0.231694778051929,
-1.60414638338378));
#67609=CARTESIAN_POINT('Ctrl Pts',(0.0531667062711942,0.231141981113734,
-1.6043139969158));
#67610=CARTESIAN_POINT('Ctrl Pts',(0.0542914404429776,0.23088038786852,
-1.60439108366358));
#67611=CARTESIAN_POINT('Ctrl Pts',(0.0567851649177315,0.230281162352141,
-1.60456288717164));
#67612=CARTESIAN_POINT('Ctrl Pts',(0.0581531358986633,0.229939516666364,
-1.60465773071789));
#67613=CARTESIAN_POINT('Ctrl Pts',(0.0621051226769359,0.22891500090963,
-1.60493350641761));
#67614=CARTESIAN_POINT('Ctrl Pts',(0.0646806727077449,0.228200642995041,
-1.60511544666754));
#67615=CARTESIAN_POINT('Ctrl Pts',(0.0797593891788329,0.223742620004651,
-1.60619412201389));
#67616=CARTESIAN_POINT('Ctrl Pts',(0.0919463914150931,0.219016163076366,
-1.60712275880188));
#67617=CARTESIAN_POINT('Ctrl Pts',(0.115478999887907,0.207578063856908,
-1.60902104079597));
#67618=CARTESIAN_POINT('Ctrl Pts',(0.126780616184222,0.200874907416396,
-1.60998749903883));
#67619=CARTESIAN_POINT('Ctrl Pts',(0.142547492591773,0.189660264730919,
-1.61137876604397));
#67620=CARTESIAN_POINT('Ctrl Pts',(0.147481153179584,0.185849746311779,
-1.61182075172669));
#67621=CARTESIAN_POINT('Ctrl Pts',(0.153298359573892,0.180979086231881,
-1.61234488653896));
#67622=CARTESIAN_POINT('Ctrl Pts',(0.154329849179837,0.180100290311074,
-1.6124379422448));
#67623=CARTESIAN_POINT('Ctrl Pts',(0.155932290767049,0.178711184568227,
-1.61258261577368));
#67624=CARTESIAN_POINT('Ctrl Pts',(0.156508379807423,0.178206885067961,
-1.61263464939922));
#67625=CARTESIAN_POINT('Ctrl Pts',(0.157570181228333,0.177268280053452,
-1.61273057893336));
#67626=CARTESIAN_POINT('Ctrl Pts',(0.1580565452793,0.176834763649822,-1.61277452801657));
#67627=CARTESIAN_POINT('Ctrl Pts',(0.159177733372892,0.17582708106696,-1.61287586843687));
#67628=CARTESIAN_POINT('Ctrl Pts',(0.159811241793498,0.175251477288967,
-1.61293315121102));
#67629=CARTESIAN_POINT('Ctrl Pts',(0.16179816855889,0.173426428275415,-1.61311293510964));
#67630=CARTESIAN_POINT('Ctrl Pts',(0.163140195008985,0.172164603393105,
-1.61323454790499));
#67631=CARTESIAN_POINT('Ctrl Pts',(0.166281119511135,0.169141675263853,
-1.61352000616053));
#67632=CARTESIAN_POINT('Ctrl Pts',(0.16806697907303,0.167367286711644,-1.61368297513337));
#67633=CARTESIAN_POINT('Ctrl Pts',(0.174545201819023,0.160722394205297,
-1.61427819753519));
#67634=CARTESIAN_POINT('Ctrl Pts',(0.1790571657802,0.155679993082782,-1.61470086562913));
#67635=CARTESIAN_POINT('Ctrl Pts',(0.193177831506098,0.138471819306723,
-1.61607751793761));
#67636=CARTESIAN_POINT('Ctrl Pts',(0.201810001450371,0.125558124101835,
-1.61701188170121));
#67637=CARTESIAN_POINT('Ctrl Pts',(0.212784142470918,0.105048462862456,
-1.61847031792467));
#67638=CARTESIAN_POINT('Ctrl Pts',(0.216108627861405,0.0980271018759928,
-1.61896505258933));
#67639=CARTESIAN_POINT('Ctrl Pts',(0.219911011325856,0.0888583373384086,
-1.61961276853596));
#67640=CARTESIAN_POINT('Ctrl Pts',(0.220712028667404,0.0868496223938283,
-1.61975475479359));
#67641=CARTESIAN_POINT('Ctrl Pts',(0.221950990051769,0.0836147882397324,
-1.61998367948646));
#67642=CARTESIAN_POINT('Ctrl Pts',(0.222406512295942,0.082395497273673,
-1.62007002743457));
#67643=CARTESIAN_POINT('Ctrl Pts',(0.223253593823615,0.0800699104714561,
-1.62023486571211));
#67644=CARTESIAN_POINT('Ctrl Pts',(0.223647024587239,0.0789643338852406,
-1.62031329085876));
#67645=CARTESIAN_POINT('Ctrl Pts',(0.224526985280065,0.0764322257864434,
-1.62049307136517));
#67646=CARTESIAN_POINT('Ctrl Pts',(0.225008149815646,0.0750038971754316,
-1.6205946006837));
#67647=CARTESIAN_POINT('Ctrl Pts',(0.226458168703679,0.0705599792611813,
-1.62091090327736));
#67648=CARTESIAN_POINT('Ctrl Pts',(0.227380217964405,0.0675296056053373,
-1.62112719237233));
#67649=CARTESIAN_POINT('Ctrl Pts',(0.229386152900982,0.0604293519272302,
-1.62163558522881));
#67650=CARTESIAN_POINT('Ctrl Pts',(0.230422839012534,0.0563473620230462,
-1.62192909662139));
#67651=CARTESIAN_POINT('Ctrl Pts',(0.233833177876745,0.0412443651867521,
-1.62301962732722));
#67652=CARTESIAN_POINT('Ctrl Pts',(0.235528749373441,0.0300867145550502,
-1.6238350251399));
#67653=CARTESIAN_POINT('Ctrl Pts',(0.237624724114097,0.00380089811443625,
-1.62575870348746));
#67654=CARTESIAN_POINT('Ctrl Pts',(0.237384977223515,-0.0113316018646385,
-1.62686903423174));
#67655=CARTESIAN_POINT('Ctrl Pts',(0.235486256780553,-0.0283228907579257,
-1.62806030653738));
#67656=CARTESIAN_POINT('Ctrl Pts',(0.235239595441707,-0.030303410158227,
-1.62819825814928));
#67657=CARTESIAN_POINT('Ctrl Pts',(0.234857787833126,-0.0330825526157371,
-1.62839034852503));
#67658=CARTESIAN_POINT('Ctrl Pts',(0.234743514883374,-0.0338838908928301,
-1.62844556132753));
#67659=CARTESIAN_POINT('Ctrl Pts',(0.234527749747542,-0.035343439573764,
-1.62854578780731));
#67660=CARTESIAN_POINT('Ctrl Pts',(0.234427583449303,-0.0360018372403216,
-1.62859087400398));
#67661=CARTESIAN_POINT('Ctrl Pts',(0.234214139111045,-0.0373661446680005,
-1.62868402845268));
#67662=CARTESIAN_POINT('Ctrl Pts',(0.234100440947087,-0.0380719753836788,
-1.62873207294345));
#67663=CARTESIAN_POINT('Ctrl Pts',(0.233793764919076,-0.0399224693310695,
-1.62885766585968));
#67664=CARTESIAN_POINT('Ctrl Pts',(0.233595569306069,-0.0410662660881281,
-1.62893492673946));
#67665=CARTESIAN_POINT('Ctrl Pts',(0.232655255169041,-0.0462656568579803,
-1.62928464530654));
#67666=CARTESIAN_POINT('Ctrl Pts',(0.231815813809006,-0.0503032028047273,
-1.6295520886842));
#67667=CARTESIAN_POINT('Ctrl Pts',(0.229069316080241,-0.061977022304927,
-1.63031871594378));
#67668=CARTESIAN_POINT('Ctrl Pts',(0.226886923580297,-0.0695431197798385,
-1.63080731984747));
#67669=CARTESIAN_POINT('Ctrl Pts',(0.218115398944938,-0.095102373304124,
-1.63247117722391));
#67670=CARTESIAN_POINT('Ctrl Pts',(0.209728011531457,-0.112396144146593,
-1.63362659751256));
#67671=CARTESIAN_POINT('Ctrl Pts',(0.197362698131944,-0.13158054532031,
-1.63509467646254));
#67672=CARTESIAN_POINT('Ctrl Pts',(0.195301209558607,-0.134621356780313,
-1.63533329059811));
#67673=CARTESIAN_POINT('Ctrl Pts',(0.192312151569573,-0.138817156949249,
-1.63567164988855));
#67674=CARTESIAN_POINT('Ctrl Pts',(0.191443052722284,-0.140013299739052,
-1.63576917818688));
#67675=CARTESIAN_POINT('Ctrl Pts',(0.189911135091101,-0.142080750622941,
-1.63593966554805));
#67676=CARTESIAN_POINT('Ctrl Pts',(0.189253355222977,-0.142955749787963,
-1.63601242797433));
#67677=CARTESIAN_POINT('Ctrl Pts',(0.18786376721004,-0.144777823008143,
-1.63616524394636));
#67678=CARTESIAN_POINT('Ctrl Pts',(0.187130802085842,-0.145723971553174,
-1.63624534168774));
#67679=CARTESIAN_POINT('Ctrl Pts',(0.185364857989815,-0.147968247098068,
-1.63643714665675));
#67680=CARTESIAN_POINT('Ctrl Pts',(0.184325370326003,-0.149261148116954,
-1.63654911142046));
#67681=CARTESIAN_POINT('Ctrl Pts',(0.180703527281388,-0.153670412735909,
-1.63693611973467));
#67682=CARTESIAN_POINT('Ctrl Pts',(0.178055145383202,-0.156731369612234,
-1.63721381912614));
#67683=CARTESIAN_POINT('Ctrl Pts',(0.160653110548373,-0.175833805542629,
-1.639006847277));
#67684=CARTESIAN_POINT('Ctrl Pts',(0.143827426909285,-0.189842733681717,
-1.64061450061909));
#67685=CARTESIAN_POINT('Ctrl Pts',(0.12458568285217,-0.201819625353787,
-1.64225777891425));
#67686=CARTESIAN_POINT('Ctrl Pts',(0.123836716298305,-0.202280056526028,
-1.64232144152219));
#67687=CARTESIAN_POINT('Ctrl Pts',(0.120111675296871,-0.204541602126206,
-1.64263653581542));
#67688=CARTESIAN_POINT('Ctrl Pts',(0.117098670355735,-0.206281324546274,
-1.64288657011153));
#67689=CARTESIAN_POINT('Ctrl Pts',(0.110150669761161,-0.210091818195628,
-1.64345068357491));
#67690=CARTESIAN_POINT('Ctrl Pts',(0.10619332500407,-0.212119603072217,
-1.64376315946186));
#67691=CARTESIAN_POINT('Ctrl Pts',(0.101065179174825,-0.214567795967495,
-1.64415488220214));
#67692=CARTESIAN_POINT('Ctrl Pts',(0.0999451565232579,-0.215091783576791,
-1.64423964836462));
#67693=CARTESIAN_POINT('Ctrl Pts',(0.0981559607496579,-0.215911841441022,
-1.64437374925309));
#67694=CARTESIAN_POINT('Ctrl Pts',(0.0974894460041401,-0.216213607018129,
-1.64442341769012));
#67695=CARTESIAN_POINT('Ctrl Pts',(0.0962134395366314,-0.21678422083649,
-1.64451794301122));
#67696=CARTESIAN_POINT('Ctrl Pts',(0.095604202864094,-0.217053589595494,
-1.64456282941928));
#67697=CARTESIAN_POINT('Ctrl Pts',(0.0941485192184657,-0.217689889603353,
-1.64466951028082));
#67698=CARTESIAN_POINT('Ctrl Pts',(0.0933010406874348,-0.218054460133688,
-1.6447311627555));
#67699=CARTESIAN_POINT('Ctrl Pts',(0.0904060112228617,-0.219279883122465,
-1.64494029382484));
#67700=CARTESIAN_POINT('Ctrl Pts',(0.0883484308578926,-0.220116945397696,
-1.64508642347101));
#67701=CARTESIAN_POINT('Ctrl Pts',(0.083276931842472,-0.222097551381693,
-1.64544121499253));
#67702=CARTESIAN_POINT('Ctrl Pts',(0.0802508133774784,-0.223208823270988,
-1.64564831534385));
#67703=CARTESIAN_POINT('Ctrl Pts',(0.0675510058753456,-0.227580843852173,
-1.64650212849881));
#67704=CARTESIAN_POINT('Ctrl Pts',(0.0576939746507311,-0.230277258892178,
-1.64712851635495));
#67705=CARTESIAN_POINT('Ctrl Pts',(0.0311626151990876,-0.235723668564269,
-1.64878880045725));
#67706=CARTESIAN_POINT('Ctrl Pts',(0.0143191388386974,-0.237342864681485,
-1.64982015376749));
#67707=CARTESIAN_POINT('Ctrl Pts',(-0.00571599421691471,-0.237127213773188,
-1.65111512222287));
#67708=CARTESIAN_POINT('Ctrl Pts',(-0.00887814354972187,-0.237029882352843,
-1.65132136430564));
#67709=CARTESIAN_POINT('Ctrl Pts',(-0.0135418026440606,-0.236792883404537,
-1.65162872000869));
#67710=CARTESIAN_POINT('Ctrl Pts',(-0.0150455296281969,-0.236702095284314,
-1.65172831045588));
#67711=CARTESIAN_POINT('Ctrl Pts',(-0.0177188107137425,-0.236515118462665,
-1.65190627447209));
#67712=CARTESIAN_POINT('Ctrl Pts',(-0.0188887182533277,-0.236424562497925,
-1.65198446907519));
#67713=CARTESIAN_POINT('Ctrl Pts',(-0.0213552248115881,-0.236215220097435,
-1.65215000743558));
#67714=CARTESIAN_POINT('Ctrl Pts',(-0.0226516100724843,-0.236094430845322,
-1.65223741161772));
#67715=CARTESIAN_POINT('Ctrl Pts',(-0.0261001806599078,-0.235744449584559,
-1.65247101203827));
#67716=CARTESIAN_POINT('Ctrl Pts',(-0.0282502914752019,-0.235496465854739,
-1.6526177931089));
#67717=CARTESIAN_POINT('Ctrl Pts',(-0.0391383057254565,-0.234089440979614,
-1.65336706789977));
#67718=CARTESIAN_POINT('Ctrl Pts',(-0.0478091099154606,-0.232473500080804,
-1.65398374875289));
#67719=CARTESIAN_POINT('Ctrl Pts',(-0.0671943387794745,-0.227730333746132,
-1.6554076783253));
#67720=CARTESIAN_POINT('Ctrl Pts',(-0.0778187542503669,-0.224322067731814,
-1.65622077518125));
#67721=CARTESIAN_POINT('Ctrl Pts',(-0.0994633979154409,-0.215655227443034,
-1.65792353899741));
#67722=CARTESIAN_POINT('Ctrl Pts',(-0.110399512114428,-0.210266857668785,
-1.65881090526219));
#67723=CARTESIAN_POINT('Ctrl Pts',(-0.12265490928234,-0.203007478089665,
-1.65980447447126));
#67724=CARTESIAN_POINT('Ctrl Pts',(-0.124421567514111,-0.201929535224735,
-1.65994765152851));
#67725=CARTESIAN_POINT('Ctrl Pts',(-0.126941264798086,-0.200346492504208,
-1.66015154053104));
#67726=CARTESIAN_POINT('Ctrl Pts',(-0.12770581270293,-0.199860019105865,
-1.66021336352036));
#67727=CARTESIAN_POINT('Ctrl Pts',(-0.129018981398303,-0.199013852198732,
-1.66031944990293));
#67728=CARTESIAN_POINT('Ctrl Pts',(-0.129568928424485,-0.198656245203887,
-1.6603638476303));
#67729=CARTESIAN_POINT('Ctrl Pts',(-0.130629593675061,-0.197960261613705,
-1.66044940783192));
#67730=CARTESIAN_POINT('Ctrl Pts',(-0.131140489568088,-0.197622184836077,
-1.66049059050903));
#67731=CARTESIAN_POINT('Ctrl Pts',(-0.132550158912963,-0.19668148594751,
-1.66060415736031));
#67732=CARTESIAN_POINT('Ctrl Pts',(-0.133446141143098,-0.196074677275335,
-1.66067626686307));
#67733=CARTESIAN_POINT('Ctrl Pts',(-0.137117779568356,-0.193551214581425,
-1.66097160074371));
#67734=CARTESIAN_POINT('Ctrl Pts',(-0.139856701605216,-0.191581481382912,
-1.66119152444396));
#67735=CARTESIAN_POINT('Ctrl Pts',(-0.147172934558227,-0.186079352714719,
-1.66178070692516));
#67736=CARTESIAN_POINT('Ctrl Pts',(-0.151664788468511,-0.182436836735152,
-1.66214435185298));
#67737=CARTESIAN_POINT('Ctrl Pts',(-0.169258844545271,-0.167070112726255,
-1.66359678140266));
#67738=CARTESIAN_POINT('Ctrl Pts',(-0.1811716340073,-0.154070887154443,
-1.66465066145245));
#67739=CARTESIAN_POINT('Ctrl Pts',(-0.195797262466384,-0.134043094438326,
-1.6662098858082));
#67740=CARTESIAN_POINT('Ctrl Pts',(-0.199786798348596,-0.128020852332756,
-1.66667102606022));
#67741=CARTESIAN_POINT('Ctrl Pts',(-0.204580115768191,-0.120014240902144,
-1.66728030973783));
#67742=CARTESIAN_POINT('Ctrl Pts',(-0.205640747018169,-0.118187666354509,
-1.6674190492857));
#67743=CARTESIAN_POINT('Ctrl Pts',(-0.207309952707263,-0.115222523554017,
-1.66764398540523));
#67744=CARTESIAN_POINT('Ctrl Pts',(-0.207933889060767,-0.114092699563961,
-1.66772962820959));
#67745=CARTESIAN_POINT('Ctrl Pts',(-0.209108715401395,-0.111923675214683,
-1.6678939484224));
#67746=CARTESIAN_POINT('Ctrl Pts',(-0.20966115893827,-0.110885356458971,
-1.66797256749072));
#67747=CARTESIAN_POINT('Ctrl Pts',(-0.210913680279988,-0.108488414087502,
-1.66815398618416));
#67748=CARTESIAN_POINT('Ctrl Pts',(-0.211608387434762,-0.107127058660382,
-1.66825697118826));
#67749=CARTESIAN_POINT('Ctrl Pts',(-0.213753108207485,-0.102821968548953,
-1.66858253831989));
#67750=CARTESIAN_POINT('Ctrl Pts',(-0.215155161109763,-0.099854911012428,
-1.66880676691892));
#67751=CARTESIAN_POINT('Ctrl Pts',(-0.218296098698196,-0.0928344812107769,
-1.669337227123));
#67752=CARTESIAN_POINT('Ctrl Pts',(-0.219984321796218,-0.0887599091338202,
-1.66964504032935));
#67753=CARTESIAN_POINT('Ctrl Pts',(-0.225920895096946,-0.0732201963942533,
-1.67081877307354));
#67754=CARTESIAN_POINT('Ctrl Pts',(-0.229393855406376,-0.0614804579089014,
-1.67170631270962));
#67755=CARTESIAN_POINT('Ctrl Pts',(-0.234975782045599,-0.0353388640426506,
-1.6736582750488));
#67756=CARTESIAN_POINT('Ctrl Pts',(-0.236697422564825,-0.020901481585207,
-1.67472107080143));
#67757=CARTESIAN_POINT('Ctrl Pts',(-0.237127843845484,-0.00494658693984074,
-1.67582647678214));
#67758=CARTESIAN_POINT('Ctrl Pts',(-0.237153654686387,-0.00349676692401314,
-1.67592628109097));
#67759=CARTESIAN_POINT('Ctrl Pts',(-0.237170415107311,-0.00155466799264505,
-1.67605903166901));
#67760=CARTESIAN_POINT('Ctrl Pts',(-0.237173130369242,-0.0010625612894877,
-1.6760925882354));
#67761=CARTESIAN_POINT('Ctrl Pts',(-0.237174766855387,-0.000382157342303444,
-1.67613886949327));
#67762=CARTESIAN_POINT('Ctrl Pts',(-0.237174995504198,-0.000193869267784506,
-1.67615166469862));
#67763=CARTESIAN_POINT('Ctrl Pts',(-0.237174999934351,-5.58036924603097E-6,
-1.6761644476277));
#67764=CARTESIAN_POINT('Ctrl Pts',(-0.237174999935275,-5.54095249315624E-6,
-1.6761644503037));
#67765=CARTESIAN_POINT('Ctrl Pts',(-0.237175003412458,0.000143296411532458,
-1.67617455486763));
#67766=CARTESIAN_POINT('Ctrl Pts',(-0.237174866787022,0.00029213433142796,
-1.67618465176352));
#67767=CARTESIAN_POINT('Ctrl Pts',(-0.237173764301833,0.000885099671302591,
-1.67622484650095));
#67768=CARTESIAN_POINT('Ctrl Pts',(-0.237171691051888,0.00132922972991396,
-1.67625488299834));
#67769=CARTESIAN_POINT('Ctrl Pts',(-0.237163054307791,0.0024843037420253,
-1.67633281664781));
#67770=CARTESIAN_POINT('Ctrl Pts',(-0.237154541646107,0.00319523146845797,
-1.67638060341992));
#67771=CARTESIAN_POINT('Ctrl Pts',(-0.237124732704956,0.00500494879468164,
-1.676501814298));
#67772=CARTESIAN_POINT('Ctrl Pts',(-0.237098995752081,0.00610366309204758,
-1.67657499664219));
#67773=CARTESIAN_POINT('Ctrl Pts',(-0.236962674218472,0.0105907941415603,
-1.67687235438578));
#67774=CARTESIAN_POINT('Ctrl Pts',(-0.236787076666774,0.0139770201528288,
-1.67709322101093));
#67775=CARTESIAN_POINT('Ctrl Pts',(-0.236333966548885,0.0201514036218907,
-1.67749138378574));
#67776=CARTESIAN_POINT('Ctrl Pts',(-0.236079553186763,0.0229405448033126,
-1.67766953876236));
#67777=CARTESIAN_POINT('Ctrl Pts',(-0.233709624884289,0.0446618178700894,
-1.6790481268826));
#67778=CARTESIAN_POINT('Ctrl Pts',(-0.2293695077312,0.0632818324143625,
-1.68018283632627));
#67779=CARTESIAN_POINT('Ctrl Pts',(-0.220905147427721,0.0865165795628418,
-1.68172833276153));
#67780=CARTESIAN_POINT('Ctrl Pts',(-0.218771413377802,0.0917783445964427,
-1.68208705324888));
#67781=CARTESIAN_POINT('Ctrl Pts',(-0.214828922389161,0.10057962302854,
-1.68270634029631));
#67782=CARTESIAN_POINT('Ctrl Pts',(-0.213116199490399,0.104159536366658,
-1.68296384762949));
#67783=CARTESIAN_POINT('Ctrl Pts',(-0.210567004580605,0.109161475097841,
-1.68333255980468));
#67784=CARTESIAN_POINT('Ctrl Pts',(-0.209804210028063,0.110620451497574,
-1.68344120307412));
#67785=CARTESIAN_POINT('Ctrl Pts',(-0.208461824726874,0.113124158890964,
-1.68362960511825));
#67786=CARTESIAN_POINT('Ctrl Pts',(-0.20788940827443,0.114172682946437,
-1.68370910777592));
#67787=CARTESIAN_POINT('Ctrl Pts',(-0.206776031325403,0.116175977033382,
-1.68386218600479));
#67788=CARTESIAN_POINT('Ctrl Pts',(-0.206236316398129,0.117131406969948,
-1.68393571540357));
#67789=CARTESIAN_POINT('Ctrl Pts',(-0.204948486762792,0.119374689900586,
-1.68410961031858));
#67790=CARTESIAN_POINT('Ctrl Pts',(-0.204194840163119,0.120659296738656,
-1.68421017382159));
#67791=CARTESIAN_POINT('Ctrl Pts',(-0.20150703271411,0.125143413758136,
-1.68456473169383));
#67792=CARTESIAN_POINT('Ctrl Pts',(-0.199509453618836,0.128304066147017,
-1.68482101947851));
#67793=CARTESIAN_POINT('Ctrl Pts',(-0.18339732705697,0.152510759688757,
-1.68683525745198));
#67794=CARTESIAN_POINT('Ctrl Pts',(-0.166067080113734,0.171217097387719,
-1.68872542029754));
#67795=CARTESIAN_POINT('Ctrl Pts',(-0.143196532691493,0.189104367221874,
-1.69080483405225));
#67796=CARTESIAN_POINT('Ctrl Pts',(-0.140224753548115,0.191318400208875,
-1.69106779016169));
#67797=CARTESIAN_POINT('Ctrl Pts',(-0.135193480051496,0.194886550803115,
-1.69149961849899));
#67798=CARTESIAN_POINT('Ctrl Pts',(-0.133162637147586,0.196279795188257,
-1.69167043611682));
#67799=CARTESIAN_POINT('Ctrl Pts',(-0.130492895897082,0.19805083639496,
-1.69189013149301));
#67800=CARTESIAN_POINT('Ctrl Pts',(-0.129873500436236,0.198457561200043,
-1.69194076727626));
#67801=CARTESIAN_POINT('Ctrl Pts',(-0.128664819944472,0.199243156716865,
-1.69203891232782));
#67802=CARTESIAN_POINT('Ctrl Pts',(-0.128075742800216,0.199622332238864,
-1.6920864409107));
#67803=CARTESIAN_POINT('Ctrl Pts',(-0.126943583072925,0.200344003040888,
-1.69217719191584));
#67804=CARTESIAN_POINT('Ctrl Pts',(-0.126400781153951,0.200686908820421,
-1.69222044007238));
#67805=CARTESIAN_POINT('Ctrl Pts',(-0.125088546889456,0.201508454316071,
-1.69232437979053));
#67806=CARTESIAN_POINT('Ctrl Pts',(-0.124317740655207,0.201984903270952,
-1.69238492892121));
#67807=CARTESIAN_POINT('Ctrl Pts',(-0.121777859780622,0.20353480114067,
-1.69258285720489));
#67808=CARTESIAN_POINT('Ctrl Pts',(-0.119997408367916,0.204589552782499,
-1.69271909338105));
#67809=CARTESIAN_POINT('Ctrl Pts',(-0.107663265693049,0.211679962274617,
-1.6936473766617));
#67810=CARTESIAN_POINT('Ctrl Pts',(-0.0966715123753824,0.216920446875706,
-1.69439795221352));
#67811=CARTESIAN_POINT('Ctrl Pts',(-0.0752178915824162,0.22519234343167,
-1.69580926644089));
#67812=CARTESIAN_POINT('Ctrl Pts',(-0.0648557486026952,0.228392304754425,
-1.69646929077252));
#67813=CARTESIAN_POINT('Ctrl Pts',(-0.0502099450086752,0.231837650920918,
-1.69740741540228));
#67814=CARTESIAN_POINT('Ctrl Pts',(-0.0460843784969549,0.232692817260734,
-1.6976721470331));
#67815=CARTESIAN_POINT('Ctrl Pts',(-0.0419392692346775,0.233437525520344,
-1.69793969278784));
#67816=CARTESIAN_POINT('',(-0.237174910032345,-0.000206582064046445,-1.69575651031441));
#67817=CARTESIAN_POINT('Ctrl Pts',(-0.0419393124730366,0.233437517752158,
-1.71790170279738));
#67818=CARTESIAN_POINT('Ctrl Pts',(-0.052470414665017,0.231545503178974,
-1.71724117783118));
#67819=CARTESIAN_POINT('Ctrl Pts',(-0.0628695321719981,0.228941590339487,
-1.71657092986479));
#67820=CARTESIAN_POINT('Ctrl Pts',(-0.0759806226596189,0.22469605505406,
-1.71567946392309));
#67821=CARTESIAN_POINT('Ctrl Pts',(-0.0788774560950214,0.223695591578132,
-1.71547954587856));
#67822=CARTESIAN_POINT('Ctrl Pts',(-0.0831502404666846,0.222126609230186,
-1.71517985700841));
#67823=CARTESIAN_POINT('Ctrl Pts',(-0.0845416118194761,0.221600786819642,
-1.71508149983606));
#67824=CARTESIAN_POINT('Ctrl Pts',(-0.0870192971135828,0.220637697656498,
-1.71490492890357));
#67825=CARTESIAN_POINT('Ctrl Pts',(-0.0881075014422767,0.220205403663207,
-1.71482688398868));
#67826=CARTESIAN_POINT('Ctrl Pts',(-0.0892370120543696,0.219746987733947,
-1.71474534935636));
#67827=CARTESIAN_POINT('Ctrl Pts',(-0.0892815750003084,0.219728885911692,
-1.71474213168723));
#67828=CARTESIAN_POINT('Ctrl Pts',(-0.0893608251426186,0.219696665785716,
-1.71473640790215));
#67829=CARTESIAN_POINT('Ctrl Pts',(-0.0893955145187637,0.219682552815313,
-1.71473390196658));
#67830=CARTESIAN_POINT('Ctrl Pts',(-0.0894572124536817,0.21965743469228,
-1.7147294440264));
#67831=CARTESIAN_POINT('Ctrl Pts',(-0.0894842223347905,0.219646432770289,
-1.71472749213109));
#67832=CARTESIAN_POINT('Ctrl Pts',(-0.0895322678313714,0.219626852087955,
-1.71472401951473));
#67833=CARTESIAN_POINT('Ctrl Pts',(-0.089553304248772,0.219618275285139,
-1.71472249885993));
#67834=CARTESIAN_POINT('Ctrl Pts',(-0.0895907287796458,0.219603010578249,
-1.71471979322012));
#67835=CARTESIAN_POINT('Ctrl Pts',(-0.0896071173802752,0.219596323860614,
-1.71471860827523));
#67836=CARTESIAN_POINT('Ctrl Pts',(-0.0896482411909376,0.219579539552672,
-1.71471563460843));
#67837=CARTESIAN_POINT('Ctrl Pts',(-0.0896729754382398,0.219569439619552,
-1.71471384580728));
#67838=CARTESIAN_POINT('Ctrl Pts',(-0.0897211736445032,0.219549748957708,
-1.71471035955603));
#67839=CARTESIAN_POINT('Ctrl Pts',(-0.0897446377741547,0.219540158646032,
-1.71470866212008));
#67840=CARTESIAN_POINT('Ctrl Pts',(-0.0897903691672221,0.21952145865184,
-1.71470535336562));
#67841=CARTESIAN_POINT('Ctrl Pts',(-0.0898126365837152,0.219512349342124,
-1.71470374205975));
#67842=CARTESIAN_POINT('Ctrl Pts',(-0.0898560433057266,0.219494584507746,
-1.71470060065989));
#67843=CARTESIAN_POINT('Ctrl Pts',(-0.0898771827485931,0.219485929316583,
-1.71469907057719));
#67844=CARTESIAN_POINT('Ctrl Pts',(-0.089918397903792,0.219469047508133,
-1.71469608702622));
#67845=CARTESIAN_POINT('Ctrl Pts',(-0.08993847373847,0.21946082118981,-1.71469463356812));
#67846=CARTESIAN_POINT('Ctrl Pts',(-0.0899776219576175,0.219444773455151,
-1.71469179895807));
#67847=CARTESIAN_POINT('Ctrl Pts',(-0.0899966944527697,0.219436952306363,
-1.71469041781517));
#67848=CARTESIAN_POINT('Ctrl Pts',(-0.0900338924456024,0.219421692683195,
-1.71468772379767));
#67849=CARTESIAN_POINT('Ctrl Pts',(-0.0900520180421404,0.219414254448981,
-1.71468641093122));
#67850=CARTESIAN_POINT('Ctrl Pts',(-0.0900873751137297,0.219399739783615,
-1.71468384968175));
#67851=CARTESIAN_POINT('Ctrl Pts',(-0.0901046066777239,0.219392663567978,
-1.71468260130603));
#67852=CARTESIAN_POINT('Ctrl Pts',(-0.0901382252242824,0.219378853338914,
-1.71468016548946));
#67853=CARTESIAN_POINT('Ctrl Pts',(-0.0901546122869155,0.21937211951904,
-1.71467897805517));
#67854=CARTESIAN_POINT('Ctrl Pts',(-0.0901865882624179,0.219358975669308,
-1.71467666079328));
#67855=CARTESIAN_POINT('Ctrl Pts',(-0.0902021772467975,0.219352565813669,
-1.71467553097162));
#67856=CARTESIAN_POINT('Ctrl Pts',(-0.0902326005956391,0.219340052594271,
-1.71467332581287));
#67857=CARTESIAN_POINT('Ctrl Pts',(-0.0902474350257179,0.219333949386747,
-1.71467225048103));
#67858=CARTESIAN_POINT('Ctrl Pts',(-0.0902763901032299,0.219322033202578,
-1.71467015137112));
#67859=CARTESIAN_POINT('Ctrl Pts',(-0.0902905108069977,0.219316220367748,
-1.71466912759798));
#67860=CARTESIAN_POINT('Ctrl Pts',(-0.0903180767457681,0.219304869643581,
-1.71466712885419));
#67861=CARTESIAN_POINT('Ctrl Pts',(-0.0903315220339558,0.219299331881042,
-1.7146661538878));
#67862=CARTESIAN_POINT('Ctrl Pts',(-0.0903577731167727,0.219288516922832,
-1.71466425017275));
#67863=CARTESIAN_POINT('Ctrl Pts',(-0.0903705789589261,0.219283239841684,
-1.71466332142796));
#67864=CARTESIAN_POINT('Ctrl Pts',(-0.0903955849418993,0.219272932716641,
-1.71466150772691));
#67865=CARTESIAN_POINT('Ctrl Pts',(-0.0904077851254341,0.219267902776166,
-1.71466062277416));
#67866=CARTESIAN_POINT('Ctrl Pts',(-0.0904316115481425,0.219258077196653,
-1.71465889437314));
#67867=CARTESIAN_POINT('Ctrl Pts',(-0.090443237826432,0.219253281650786,
-1.714658050928));
#67868=CARTESIAN_POINT('Ctrl Pts',(-0.0904659463003456,0.219243912865814,
-1.71465640339346));
#67869=CARTESIAN_POINT('Ctrl Pts',(-0.0904770285312157,0.219239339710945,
-1.7146555993069));
#67870=CARTESIAN_POINT('Ctrl Pts',(-0.0918039699081931,0.218691650947072,
-1.71455931480511));
#67871=CARTESIAN_POINT('Ctrl Pts',(-0.0931148873865717,0.218136710981778,
-1.71446343469572));
#67872=CARTESIAN_POINT('Ctrl Pts',(-0.0971582988594385,0.216381957391532,
-1.71416529844162));
#67873=CARTESIAN_POINT('Ctrl Pts',(-0.0998731106176644,0.215142387458849,
-1.71396169759898));
#67874=CARTESIAN_POINT('Ctrl Pts',(-0.106112569344353,0.212149934264756,
-1.71348554241654));
#67875=CARTESIAN_POINT('Ctrl Pts',(-0.109618323557994,0.210359910666094,
-1.71321177768223));
#67876=CARTESIAN_POINT('Ctrl Pts',(-0.121922004639338,0.203686614970498,
-1.71222844444857));
#67877=CARTESIAN_POINT('Ctrl Pts',(-0.130451136622435,0.198332232430276,
-1.71150423927462));
#67878=CARTESIAN_POINT('Ctrl Pts',(-0.151424374476446,0.183226320157479,
-1.70962325668375));
#67879=CARTESIAN_POINT('Ctrl Pts',(-0.163282242033374,0.172743126392853,
-1.70845775976851));
#67880=CARTESIAN_POINT('Ctrl Pts',(-0.175868137659138,0.159153541293116,
-1.70715693223449));
#67881=CARTESIAN_POINT('Ctrl Pts',(-0.177690693889794,0.157116105018937,
-1.70696684935604));
#67882=CARTESIAN_POINT('Ctrl Pts',(-0.180151641990481,0.154267395359076,
-1.70670832070887));
#67883=CARTESIAN_POINT('Ctrl Pts',(-0.180820491580162,0.153482876263535,
-1.70663786019124));
#67884=CARTESIAN_POINT('Ctrl Pts',(-0.181882272751237,0.152220897902633,
-1.70652572413574));
#67885=CARTESIAN_POINT('Ctrl Pts',(-0.182278479926713,0.151746231180519,
-1.70648381634638));
#67886=CARTESIAN_POINT('Ctrl Pts',(-0.183107059982614,0.150745642485521,
-1.70639605052671));
#67887=CARTESIAN_POINT('Ctrl Pts',(-0.18353903194204,0.150219399268201,
-1.70635022317439));
#67888=CARTESIAN_POINT('Ctrl Pts',(-0.184602083130875,0.148912922621912,
-1.70623724713287));
#67889=CARTESIAN_POINT('Ctrl Pts',(-0.185230497398954,0.148130518610366,
-1.70617028704228));
#67890=CARTESIAN_POINT('Ctrl Pts',(-0.187566502593951,0.145183975948144,
-1.70592061279501));
#67891=CARTESIAN_POINT('Ctrl Pts',(-0.189241365110963,0.142994010776344,
-1.70574005207734));
#67892=CARTESIAN_POINT('Ctrl Pts',(-0.20025831147995,0.128056084576701,
-1.70453790643847));
#67893=CARTESIAN_POINT('Ctrl Pts',(-0.208345295510102,0.114429532041464,
-1.7035813684058));
#67894=CARTESIAN_POINT('Ctrl Pts',(-0.218749183721279,0.0920813448084949,
-1.70206876652322));
#67895=CARTESIAN_POINT('Ctrl Pts',(-0.222029858525925,0.0838624278279787,
-1.70152358359472));
#67896=CARTESIAN_POINT('Ctrl Pts',(-0.227007627957384,0.0690343756026345,
-1.7005379259616));
#67897=CARTESIAN_POINT('Ctrl Pts',(-0.228893069435958,0.0624992604882175,
-1.70010291213344));
#67898=CARTESIAN_POINT('Ctrl Pts',(-0.230982545438021,0.0538824885112005,
-1.69952371996331));
#67899=CARTESIAN_POINT('Ctrl Pts',(-0.231443652613897,0.0518661169124639,
-1.69938780314305));
#67900=CARTESIAN_POINT('Ctrl Pts',(-0.232147500154828,0.0485917628194526,
-1.69916635198425));
#67901=CARTESIAN_POINT('Ctrl Pts',(-0.232406529978652,0.0473373632120651,
-1.69908134040437));
#67902=CARTESIAN_POINT('Ctrl Pts',(-0.232884339077109,0.0449249809981179,
-1.69891748942797));
#67903=CARTESIAN_POINT('Ctrl Pts',(-0.233104673812937,0.0437673424494301,
-1.69883870232299));
#67904=CARTESIAN_POINT('Ctrl Pts',(-0.233523128832349,0.0414759391227606,
-1.69868241868451));
#67905=CARTESIAN_POINT('Ctrl Pts',(-0.233721641556557,0.0403422782272066,
-1.69860493702333));
#67906=CARTESIAN_POINT('Ctrl Pts',(-0.234160557063099,0.0377236911775027,
-1.6984255766842));
#67907=CARTESIAN_POINT('Ctrl Pts',(-0.234395097368543,0.0362378463453015,
-1.69832351555668));
#67908=CARTESIAN_POINT('Ctrl Pts',(-0.235197598807343,0.0308197225275599,
-1.69795025213469));
#67909=CARTESIAN_POINT('Ctrl Pts',(-0.23568083538695,0.0268757572059763,
-1.69767643048821));
#67910=CARTESIAN_POINT('Ctrl Pts',(-0.236811228339999,0.0152341338636049,
-1.69686161869962));
#67911=CARTESIAN_POINT('Ctrl Pts',(-0.237181636093005,0.00751554444000314,
-1.69631281396535));
#67912=CARTESIAN_POINT('Ctrl Pts',(-0.237174910032345,-0.000206582064046445,
-1.69575651031441));
#67913=CARTESIAN_POINT('Ctrl Pts',(-0.23717491023877,-0.000206344932647713,
-1.69575652739741));
#67914=CARTESIAN_POINT('Ctrl Pts',(-0.237157180591062,-0.0205849776901013,
-1.69428844669781));
#67915=CARTESIAN_POINT('Ctrl Pts',(-0.234513236349716,-0.0408764697135139,
-1.6927680918941));
#67916=CARTESIAN_POINT('Ctrl Pts',(-0.228894938723376,-0.0621425514459061,
-1.69122992573039));
#67917=CARTESIAN_POINT('Ctrl Pts',(-0.228466403219468,-0.0637000204472546,
-1.69111766083907));
#67918=CARTESIAN_POINT('Ctrl Pts',(-0.227663245470384,-0.0665065965353731,
-1.69091620357677));
#67919=CARTESIAN_POINT('Ctrl Pts',(-0.227294173327026,-0.0677572113261506,
-1.69082673957857));
#67920=CARTESIAN_POINT('Ctrl Pts',(-0.226697674189515,-0.0697187353092507,
-1.69068697001384));
#67921=CARTESIAN_POINT('Ctrl Pts',(-0.226477180202674,-0.0704317004088306,
-1.69063628214129));
#67922=CARTESIAN_POINT('Ctrl Pts',(-0.226054949474159,-0.071774492600173,
-1.69054104962184));
#67923=CARTESIAN_POINT('Ctrl Pts',(-0.225853945042602,-0.0724045129121424,
-1.69049646671612));
#67924=CARTESIAN_POINT('Ctrl Pts',(-0.225380589747264,-0.0738670261675179,
-1.69039319128249));
#67925=CARTESIAN_POINT('Ctrl Pts',(-0.225106259276207,-0.0746988613394432,
-1.690334614762));
#67926=CARTESIAN_POINT('Ctrl Pts',(-0.224188942165128,-0.0774294346738284,
-1.69014281163176));
#67927=CARTESIAN_POINT('Ctrl Pts',(-0.223526470624683,-0.0793216031707172,
-1.69001066550158));
#67928=CARTESIAN_POINT('Ctrl Pts',(-0.217567643406588,-0.0956735741837433,
-1.68887346507427));
#67929=CARTESIAN_POINT('Ctrl Pts',(-0.210897879602875,-0.109596231993451,
-1.68793639908497));
#67930=CARTESIAN_POINT('Ctrl Pts',(-0.197190004059619,-0.13225272925852,
-1.68631330835599));
#67931=CARTESIAN_POINT('Ctrl Pts',(-0.19079927011016,-0.141316295681844,
-1.68563296896661));
#67932=CARTESIAN_POINT('Ctrl Pts',(-0.181164663114807,-0.153129746536141,
-1.68466877165995));
#67933=CARTESIAN_POINT('Ctrl Pts',(-0.178445711399983,-0.156289729225064,
-1.68440254491068));
#67934=CARTESIAN_POINT('Ctrl Pts',(-0.173553953805227,-0.161680824977024,
-1.68393196751487));
#67935=CARTESIAN_POINT('Ctrl Pts',(-0.171417812881863,-0.163943880662194,
-1.68372908224305));
#67936=CARTESIAN_POINT('Ctrl Pts',(-0.168238769456387,-0.167181729418243,
-1.68343045201469));
#67937=CARTESIAN_POINT('Ctrl Pts',(-0.167230555393448,-0.168190235724517,
-1.68333621105053));
#67938=CARTESIAN_POINT('Ctrl Pts',(-0.166198053055606,-0.169204575127073,
-1.6832401477154));
#67939=CARTESIAN_POINT('Ctrl Pts',(-0.16618277781715,-0.169219577591904,
-1.68323872661598));
#67940=CARTESIAN_POINT('Ctrl Pts',(-0.166151114141369,-0.169250667419559,
-1.68323578105735));
#67941=CARTESIAN_POINT('Ctrl Pts',(-0.166134725399423,-0.169266754470103,
-1.68323425658465));
#67942=CARTESIAN_POINT('Ctrl Pts',(-0.166100704825517,-0.169300139077184,
-1.68323109224278));
#67943=CARTESIAN_POINT('Ctrl Pts',(-0.166083072628262,-0.169317436259359,
-1.6832294523574));
#67944=CARTESIAN_POINT('Ctrl Pts',(-0.166046413945018,-0.169353387184813,
-1.68322604318276));
#67945=CARTESIAN_POINT('Ctrl Pts',(-0.166027387017896,-0.169372040475925,
-1.68322427387389));
#67946=CARTESIAN_POINT('Ctrl Pts',(-0.165987761787904,-0.169410874483293,
-1.68322058945122));
#67947=CARTESIAN_POINT('Ctrl Pts',(-0.165967162948092,-0.169431054649117,
-1.68321867431354));
#67948=CARTESIAN_POINT('Ctrl Pts',(-0.165924185100876,-0.169473143608142,
-1.68321467890185));
#67949=CARTESIAN_POINT('Ctrl Pts',(-0.165901805434801,-0.16949505172508,
-1.68321259859854));
#67950=CARTESIAN_POINT('Ctrl Pts',(-0.165855017984594,-0.16954083519938,
-1.68320824990633));
#67951=CARTESIAN_POINT('Ctrl Pts',(-0.165830609384606,-0.169564709718448,
-1.68320598148113));
#67952=CARTESIAN_POINT('Ctrl Pts',(-0.165779467301703,-0.169614711164627,
-1.68320122908784));
#67953=CARTESIAN_POINT('Ctrl Pts',(-0.165752732797996,-0.169640837041939,
-1.68319874507429));
#67954=CARTESIAN_POINT('Ctrl Pts',(-0.165696580682709,-0.169695684875623,
-1.68319352837377));
#67955=CARTESIAN_POINT('Ctrl Pts',(-0.165667161779537,-0.169724405502736,
-1.68319079562923));
#67956=CARTESIAN_POINT('Ctrl Pts',(-0.165605204415702,-0.169784860812962,
-1.68318504111908));
#67957=CARTESIAN_POINT('Ctrl Pts',(-0.165572664301311,-0.169816593791666,
-1.68318201927972));
#67958=CARTESIAN_POINT('Ctrl Pts',(-0.165503927330314,-0.1698835872495,
-1.68317563694354));
#67959=CARTESIAN_POINT('Ctrl Pts',(-0.165467728327327,-0.169918845513685,
-1.68317227635091));
#67960=CARTESIAN_POINT('Ctrl Pts',(-0.165411628792834,-0.169973452207973,
-1.68316706909839));
#67961=CARTESIAN_POINT('Ctrl Pts',(-0.165391736111512,-0.169992808734408,
-1.6831652227896));
#67962=CARTESIAN_POINT('Ctrl Pts',(-0.165334626359688,-0.170048359729382,
-1.68315992270308));
#67963=CARTESIAN_POINT('Ctrl Pts',(-0.165297400820845,-0.170084545453185,
-1.68315646854648));
#67964=CARTESIAN_POINT('Ctrl Pts',(-0.165187064580053,-0.170191729253609,
-1.68314623213565));
#67965=CARTESIAN_POINT('Ctrl Pts',(-0.165113920067816,-0.170262692362983,
-1.68313944836739));
#67966=CARTESIAN_POINT('Ctrl Pts',(-0.164199874793727,-0.171148334960564,
-1.68305470274398));
#67967=CARTESIAN_POINT('Ctrl Pts',(-0.163353011594101,-0.171956811323076,
-1.68297647371683));
#67968=CARTESIAN_POINT('Ctrl Pts',(-0.161417549239935,-0.173777342178364,
-1.68279831126105));
#67969=CARTESIAN_POINT('Ctrl Pts',(-0.160325361474269,-0.174785491818389,
-1.68269821491546));
#67970=CARTESIAN_POINT('Ctrl Pts',(-0.156956597635245,-0.177836904452586,
-1.68239076207132));
#67971=CARTESIAN_POINT('Ctrl Pts',(-0.154649983447817,-0.179846376726283,
-1.68218200896848));
#67972=CARTESIAN_POINT('Ctrl Pts',(-0.138195617390948,-0.193630425809376,
-1.68070434169805));
#67973=CARTESIAN_POINT('Ctrl Pts',(-0.122760571644535,-0.203765451123917,
-1.67936921032285));
#67974=CARTESIAN_POINT('Ctrl Pts',(-0.0945483389667432,-0.217912386417895,
-1.67706425910662));
#67975=CARTESIAN_POINT('Ctrl Pts',(-0.0823114352816662,-0.222823031305432,
-1.67610472197689));
#67976=CARTESIAN_POINT('Ctrl Pts',(-0.0682932819849794,-0.227134904289521,
-1.6750895653239));
#67977=CARTESIAN_POINT('Ctrl Pts',(-0.066853297979091,-0.22756290108941,
-1.67498625766919));
#67978=CARTESIAN_POINT('Ctrl Pts',(-0.0646512577182661,-0.228194691938939,
-1.67482985751953));
#67979=CARTESIAN_POINT('Ctrl Pts',(-0.0638921225311366,-0.22840840456902,
-1.67477622446273));
#67980=CARTESIAN_POINT('Ctrl Pts',(-0.0625002784601605,-0.228792756036485,
-1.67467842857025));
#67981=CARTESIAN_POINT('Ctrl Pts',(-0.0618679247264918,-0.228964560432744,
-1.67463420162206));
#67982=CARTESIAN_POINT('Ctrl Pts',(-0.0604348370734335,-0.229347545897333,
-1.67453442861028));
#67983=CARTESIAN_POINT('Ctrl Pts',(-0.059633703299846,-0.229557155898233,
-1.67447897291913));
#67984=CARTESIAN_POINT('Ctrl Pts',(-0.0575507864926815,-0.230090493699902,
-1.67433558058076));
#67985=CARTESIAN_POINT('Ctrl Pts',(-0.0562673447682712,-0.230407713467742,
-1.67424800044231));
#67986=CARTESIAN_POINT('Ctrl Pts',(-0.0469974130212168,-0.232616822161363,
-1.67362055981486));
#67987=CARTESIAN_POINT('Ctrl Pts',(-0.0389192012064967,-0.234103972247925,
-1.67310105597248));
#67988=CARTESIAN_POINT('Ctrl Pts',(-0.0166862644013108,-0.23701384841901,
-1.67170551773418));
#67989=CARTESIAN_POINT('Ctrl Pts',(-0.00245580051308762,-0.237587850527465,
-1.67084807818523));
#67990=CARTESIAN_POINT('Ctrl Pts',(0.0222530302080953,-0.236363201104281,
-1.66931404003925));
#67991=CARTESIAN_POINT('Ctrl Pts',(0.0327177312100396,-0.235143080853157,
-1.66865037987484));
#67992=CARTESIAN_POINT('Ctrl Pts',(0.0452937888356439,-0.232820930285271,
-1.66781678782396));
#67993=CARTESIAN_POINT('Ctrl Pts',(0.047515504108547,-0.232377686477648,
-1.66766816729781));
#67994=CARTESIAN_POINT('Ctrl Pts',(0.0510246900051521,-0.231625157689122,
-1.66743110925161));
#67995=CARTESIAN_POINT('Ctrl Pts',(0.0523165433744463,-0.231336793082054,
-1.66734334039548));
#67996=CARTESIAN_POINT('Ctrl Pts',(0.0547447295738881,-0.230773399630376,
-1.667177394927));
#67997=CARTESIAN_POINT('Ctrl Pts',(0.0558815784585395,-0.230500751620637,
-1.66709929698662));
#67998=CARTESIAN_POINT('Ctrl Pts',(0.0584420225985232,-0.229866630540486,
-1.66692246664108));
#67999=CARTESIAN_POINT('Ctrl Pts',(0.0598643581327024,-0.229500318731439,
-1.66682358075949));
#68000=CARTESIAN_POINT('Ctrl Pts',(0.0641502633238746,-0.228353963467647,
-1.66652357369212));
#68001=CARTESIAN_POINT('Ctrl Pts',(0.0670025881770273,-0.22753338370541,
-1.66632115274849));
#68002=CARTESIAN_POINT('Ctrl Pts',(0.0883524898015625,-0.220955021774782,
-1.66478444993675));
#68003=CARTESIAN_POINT('Ctrl Pts',(0.106094297452694,-0.213004673118266,
-1.66337569702148));
#68004=CARTESIAN_POINT('Ctrl Pts',(0.12500412500385,-0.201577276900321,
-1.66176266752614));
#68005=CARTESIAN_POINT('Ctrl Pts',(0.127315529573917,-0.200125425793602,
-1.66156359871335));
#68006=CARTESIAN_POINT('Ctrl Pts',(0.135142654857335,-0.195018514124812,
-1.66088385192511));
#68007=CARTESIAN_POINT('Ctrl Pts',(0.140530600564594,-0.191172487870343,
-1.66040607842604));
#68008=CARTESIAN_POINT('Ctrl Pts',(0.14866222216491,-0.184838152202823,
-1.65967661453991));
#68009=CARTESIAN_POINT('Ctrl Pts',(0.151520343984657,-0.182502569553957,
-1.65941851092251));
#68010=CARTESIAN_POINT('Ctrl Pts',(0.155171268528208,-0.179374206590474,
-1.65908777643997));
#68011=CARTESIAN_POINT('Ctrl Pts',(0.156014434164411,-0.178641330669532,
-1.65901132085006));
#68012=CARTESIAN_POINT('Ctrl Pts',(0.157381320787173,-0.177436179228383,
-1.65888729935182));
#68013=CARTESIAN_POINT('Ctrl Pts',(0.157908157341729,-0.176967487720228,
-1.65883947917616));
#68014=CARTESIAN_POINT('Ctrl Pts',(0.158932493392311,-0.176047987415613,
-1.6587464784643));
#68015=CARTESIAN_POINT('Ctrl Pts',(0.159430179906112,-0.175597406247439,
-1.65870128305898));
#68016=CARTESIAN_POINT('Ctrl Pts',(0.160539718285173,-0.174584278428505,
-1.65860048510387));
#68017=CARTESIAN_POINT('Ctrl Pts',(0.161150546110789,-0.174020610737428,
-1.65854496596836));
#68018=CARTESIAN_POINT('Ctrl Pts',(0.163265368615457,-0.172048382646694,
-1.65835259681015));
#68019=CARTESIAN_POINT('Ctrl Pts',(0.164754012049177,-0.170623394586858,
-1.65821692089826));
#68020=CARTESIAN_POINT('Ctrl Pts',(0.175574246991383,-0.159992164364411,
-1.65722705216902));
#68021=CARTESIAN_POINT('Ctrl Pts',(0.184148127779807,-0.150044552570448,
-1.65642130465746));
#68022=CARTESIAN_POINT('Ctrl Pts',(0.199275683101352,-0.129230126706398,
-1.6548434990787));
#68023=CARTESIAN_POINT('Ctrl Pts',(0.205867676875826,-0.118447024207546,
-1.65407350062453));
#68024=CARTESIAN_POINT('Ctrl Pts',(0.213598510709018,-0.103188146454109,
-1.65299460121818));
#68025=CARTESIAN_POINT('Ctrl Pts',(0.215512471342336,-0.09912864528375,
-1.65270867614093));
#68026=CARTESIAN_POINT('Ctrl Pts',(0.218642217894794,-0.0919707475758003,
-1.65220445184955));
#68027=CARTESIAN_POINT('Ctrl Pts',(0.219910104286968,-0.0888964684794111,
-1.65198787499301));
#68028=CARTESIAN_POINT('Ctrl Pts',(0.221668554010249,-0.0843646386891815,
-1.65166808129659));
#68029=CARTESIAN_POINT('Ctrl Pts',(0.222210277724175,-0.0829272716628046,
-1.65156657568996));
#68030=CARTESIAN_POINT('Ctrl Pts',(0.223142306479953,-0.0803795783009577,
-1.65138647677795));
#68031=CARTESIAN_POINT('Ctrl Pts',(0.223538384402725,-0.0792714082253722,
-1.65130807863437));
#68032=CARTESIAN_POINT('Ctrl Pts',(0.224350064659753,-0.0769459777216967,
-1.65114341589405));
#68033=CARTESIAN_POINT('Ctrl Pts',(0.224764043608607,-0.0757281954622659,
-1.65105710051559));
#68034=CARTESIAN_POINT('Ctrl Pts',(0.225825612059335,-0.0725200279909076,
-1.65082945498842));
#68035=CARTESIAN_POINT('Ctrl Pts',(0.226456782289814,-0.0705243701603183,
-1.65068759140964));
#68036=CARTESIAN_POINT('Ctrl Pts',(0.229088059447948,-0.0618049349896727,
-1.65006648413415));
#68037=CARTESIAN_POINT('Ctrl Pts',(0.230815538385571,-0.0550032600622956,
-1.64957855368143));
#68038=CARTESIAN_POINT('Ctrl Pts',(0.235493073283074,-0.0324356463933141,
-1.64794783550951));
#68039=CARTESIAN_POINT('Ctrl Pts',(0.237146429378257,-0.0164474939926009,
-1.64677064021288));
#68040=CARTESIAN_POINT('Ctrl Pts',(0.237192638167339,0.0098164657577528,
-1.6448582902849));
#68041=CARTESIAN_POINT('Ctrl Pts',(0.236548263926154,0.0200419383520721,
-1.64412022645384));
#68042=CARTESIAN_POINT('Ctrl Pts',(0.235058806373024,0.0316461556477715,
-1.64331088365781));
#68043=CARTESIAN_POINT('Ctrl Pts',(0.234859091574168,0.0330957549622613,
-1.64321029781273));
#68044=CARTESIAN_POINT('Ctrl Pts',(0.234532295490491,0.0353156074959141,
-1.64305715307967));
#68045=CARTESIAN_POINT('Ctrl Pts',(0.234414810614051,0.0360872050722019,
-1.64300408655352));
#68046=CARTESIAN_POINT('Ctrl Pts',(0.234191595284752,0.0375060989005817,
-1.64290682352088));
#68047=CARTESIAN_POINT('Ctrl Pts',(0.234086988717764,0.038153538358511,
-1.64286256774081));
#68048=CARTESIAN_POINT('Ctrl Pts',(0.23384257519367,0.0396274294370454,
-1.6427620990309));
#68049=CARTESIAN_POINT('Ctrl Pts',(0.233701071910317,0.0404535805450527,
-1.6427059821209));
#68050=CARTESIAN_POINT('Ctrl Pts',(0.233319226423434,0.0426140504752146,
-1.64255970853903));
#68051=CARTESIAN_POINT('Ctrl Pts',(0.2330718136613,0.0439471114377123,-1.64246993238373));
#68052=CARTESIAN_POINT('Ctrl Pts',(0.230664970819543,0.0563227476213644,
-1.64164031538453));
#68053=CARTESIAN_POINT('Ctrl Pts',(0.227733419951994,0.0672022320847831,
-1.64093908349473));
#68054=CARTESIAN_POINT('Ctrl Pts',(0.22351973073066,0.0793310999483972,
-1.64014824972499));
#68055=CARTESIAN_POINT('Ctrl Pts',(0.222984517748316,0.0808232537580587,
-1.64005080401535));
#68056=CARTESIAN_POINT('Ctrl Pts',(0.218499832212858,0.0929426682953969,
-1.63925733015927));
#68057=CARTESIAN_POINT('Ctrl Pts',(0.213808104613146,0.103279233520729,
-1.63856710653441));
#68058=CARTESIAN_POINT('Ctrl Pts',(0.204152407266693,0.121048513537255,
-1.63730495828086));
#68059=CARTESIAN_POINT('Ctrl Pts',(0.199474550600821,0.128611135922112,
-1.63674091273525));
#68060=CARTESIAN_POINT('Ctrl Pts',(0.193141231733835,0.137670435450131,
-1.63601966279915));
#68061=CARTESIAN_POINT('Ctrl Pts',(0.191874315379319,0.139430738281067,
-1.63587727215916));
#68062=CARTESIAN_POINT('Ctrl Pts',(0.18980807663954,0.142220152053972,-1.63564786941395));
#68063=CARTESIAN_POINT('Ctrl Pts',(0.189024084804779,0.143260506967485,
-1.63556145258007));
#68064=CARTESIAN_POINT('Ctrl Pts',(0.187518083015122,0.145225082312253,
-1.63539659610589));
#68065=CARTESIAN_POINT('Ctrl Pts',(0.186797708245683,0.146150511799278,
-1.63531822254369));
#68066=CARTESIAN_POINT('Ctrl Pts',(0.185137978125632,0.148250366858739,
-1.6351387208456));
#68067=CARTESIAN_POINT('Ctrl Pts',(0.184194264453201,0.149421266824015,
-1.63503742038396));
#68068=CARTESIAN_POINT('Ctrl Pts',(0.181238757845033,0.153017723422935,
-1.63472245000505));
#68069=CARTESIAN_POINT('Ctrl Pts',(0.179189783115478,0.155412132692644,
-1.63450728212836));
#68070=CARTESIAN_POINT('Ctrl Pts',(0.165689458861937,0.170566476123119,
-1.6331090044744));
#68071=CARTESIAN_POINT('Ctrl Pts',(0.152932715529392,0.182091451040202,
-1.63186953869485));
#68072=CARTESIAN_POINT('Ctrl Pts',(0.130932188417867,0.1980129192153,-1.62988622741946));
#68073=CARTESIAN_POINT('Ctrl Pts',(0.122451475954019,0.203366691535162,
-1.62915364894644));
#68074=CARTESIAN_POINT('Ctrl Pts',(0.11085799405431,0.209696583273971,-1.62821189354252));
#68075=CARTESIAN_POINT('Ctrl Pts',(0.10802811031955,0.211168372070908,-1.62798649001198));
#68076=CARTESIAN_POINT('Ctrl Pts',(0.103194277712658,0.213559773586262,
-1.62760995108571));
#68077=CARTESIAN_POINT('Ctrl Pts',(0.101205683322833,0.214509315378902,
-1.62745741719782));
#68078=CARTESIAN_POINT('Ctrl Pts',(0.09836891670005,0.215815620864276,-1.62724345475326));
#68079=CARTESIAN_POINT('Ctrl Pts',(0.0975315296552249,0.216195344019782,
-1.62718073810462));
#68080=CARTESIAN_POINT('Ctrl Pts',(0.0960843096693439,0.216841483276736,
-1.62707313583831));
#68081=CARTESIAN_POINT('Ctrl Pts',(0.0954755308803292,0.217110217363173,
-1.62702811191803));
#68082=CARTESIAN_POINT('Ctrl Pts',(0.0941941761281132,0.21766941560904,
-1.6269338566329));
#68083=CARTESIAN_POINT('Ctrl Pts',(0.0935213780306655,0.217959329224692,
-1.62688465812623));
#68084=CARTESIAN_POINT('Ctrl Pts',(0.0917047824816403,0.218732153369597,
-1.62675257581389));
#68085=CARTESIAN_POINT('Ctrl Pts',(0.0905584994538912,0.219209216026502,
-1.62667003584843));
#68086=CARTESIAN_POINT('Ctrl Pts',(0.0852362816501132,0.221375354896636,
-1.62629027578228));
#68087=CARTESIAN_POINT('Ctrl Pts',(0.0810162119952549,0.22295437014655,
-1.62599900467261));
#68088=CARTESIAN_POINT('Ctrl Pts',(0.0735680116787141,0.225501800381747,
-1.62549769546265));
#68089=CARTESIAN_POINT('Ctrl Pts',(0.0703596525575211,0.226523366075457,
-1.62528579308882));
#68090=CARTESIAN_POINT('Ctrl Pts',(0.0621964622093398,0.228932404337942,
-1.62475429749068));
#68091=CARTESIAN_POINT('Ctrl Pts',(0.0572161794161748,0.23022762190028,
-1.62443704790002));
#68092=CARTESIAN_POINT('Ctrl Pts',(0.0388132782934101,0.234379537614686,
-1.62327816374289));
#68093=CARTESIAN_POINT('Ctrl Pts',(0.0251929274813872,0.236231946603039,
-1.62244461852425));
#68094=CARTESIAN_POINT('Ctrl Pts',(0.00680270278645107,0.237123845681054,
-1.62128531824732));
#68095=CARTESIAN_POINT('Ctrl Pts',(0.0021108001608454,0.237212004935238,
-1.62098680656104));
#68096=CARTESIAN_POINT('Ctrl Pts',(-0.00602025926877484,0.237123535332844,
-1.62046246901015));
#68097=CARTESIAN_POINT('Ctrl Pts',(-0.00945872637578249,0.237011276234417,
-1.62023856695493));
#68098=CARTESIAN_POINT('Ctrl Pts',(-0.0144478135261466,0.236739655900411,
-1.61990997126444));
#68099=CARTESIAN_POINT('Ctrl Pts',(-0.0160013252897077,0.23663972909591,
-1.61980712854234));
#68100=CARTESIAN_POINT('Ctrl Pts',(-0.0187302043561134,0.236437204838378,
-1.61962550385825));
#68101=CARTESIAN_POINT('Ctrl Pts',(-0.0199060119794063,0.236341115737117,
-1.6195469283242));
#68102=CARTESIAN_POINT('Ctrl Pts',(-0.0223528122925231,0.23612277040315,
-1.61938273148388));
#68103=CARTESIAN_POINT('Ctrl Pts',(-0.0236236294669529,0.235999014702225,
-1.6192970655003));
#68104=CARTESIAN_POINT('Ctrl Pts',(-0.0269318279979655,0.235649865024365,
-1.61907302355486));
#68105=CARTESIAN_POINT('Ctrl Pts',(-0.0289673591628409,0.235408313124346,
-1.61893414455652));
#68106=CARTESIAN_POINT('Ctrl Pts',(-0.034659392386036,0.23465791087814,
-1.61854280990291));
#68107=CARTESIAN_POINT('Ctrl Pts',(-0.038306984633953,0.2340901000619,-1.61828856529244));
#68108=CARTESIAN_POINT('Ctrl Pts',(-0.0419392757399419,0.233437524351611,
-1.61803181050061));
#68109=CARTESIAN_POINT('Origin',(0.,0.,-2.1456589891905));
#68110=CARTESIAN_POINT('',(-0.0419392735583895,0.233437524743548,-1.49813919362704));
#68111=CARTESIAN_POINT('',(-0.0419392871413391,0.233437522303241,-1.51768363453027));
#68112=CARTESIAN_POINT('',(-0.0419392741328076,0.233437524640348,-2.1456589891905));
#68113=CARTESIAN_POINT('Ctrl Pts',(-0.0419392735583878,0.233437524743548,
-1.49813919362704));
#68114=CARTESIAN_POINT('Ctrl Pts',(-0.0403526003689305,0.233722585686572,
-1.49825693285339));
#68115=CARTESIAN_POINT('Ctrl Pts',(-0.0387626152701877,0.233991542611384,
-1.49837468919692));
#68116=CARTESIAN_POINT('Ctrl Pts',(-0.0349451157565634,0.234597298026795,
-1.49865674407909));
#68117=CARTESIAN_POINT('Ctrl Pts',(-0.0327157377689241,0.234918568965427,
-1.49882091429307));
#68118=CARTESIAN_POINT('Ctrl Pts',(-0.0239929327900559,0.236049012636772,
-1.49946050857385));
#68119=CARTESIAN_POINT('Ctrl Pts',(-0.01747128207471,0.236621138183647,
-1.49993284946457));
#68120=CARTESIAN_POINT('Ctrl Pts',(-0.00727404522223611,0.237091737755044,
-1.50065512348649));
#68121=CARTESIAN_POINT('Ctrl Pts',(-0.00361049104734264,0.237175824764138,
-1.50091133227188));
#68122=CARTESIAN_POINT('Ctrl Pts',(0.00116829973749349,0.237174741188912,
-1.50124004805536));
#68123=CARTESIAN_POINT('Ctrl Pts',(0.00228283310931947,0.237166632515784,
-1.50131632319342));
#68124=CARTESIAN_POINT('Ctrl Pts',(0.00410194056428352,0.237140572942378,
-1.50144013674687));
#68125=CARTESIAN_POINT('Ctrl Pts',(0.00480654913001082,0.237127337880786,
-1.50148792771894));
#68126=CARTESIAN_POINT('Ctrl Pts',(0.00618294274336731,0.237095346771428,
-1.50158094413403));
#68127=CARTESIAN_POINT('Ctrl Pts',(0.00685472176362094,0.237076875819526,
-1.50162618396144));
#68128=CARTESIAN_POINT('Ctrl Pts',(0.00835912202114733,0.237029111703741,
-1.50172715707174));
#68129=CARTESIAN_POINT('Ctrl Pts',(0.00919169422975093,0.236998285912196,
-1.50178280611683));
#68130=CARTESIAN_POINT('Ctrl Pts',(0.0120934306043169,0.236875535553353,
-1.50197600320352));
#68131=CARTESIAN_POINT('Ctrl Pts',(0.0141616101806051,0.236760891874265,
-1.50211236411089));
#68132=CARTESIAN_POINT('Ctrl Pts',(0.0283593181106992,0.235787167133492,
-1.50304089513483));
#68133=CARTESIAN_POINT('Ctrl Pts',(0.0404102307192574,0.234023350843837,
-1.50379158936632));
#68134=CARTESIAN_POINT('Ctrl Pts',(0.0628473306437485,0.228953483000353,
-1.50520348802103));
#68135=CARTESIAN_POINT('Ctrl Pts',(0.0732442863940249,0.225842310135339,
-1.50586397007022));
#68136=CARTESIAN_POINT('Ctrl Pts',(0.091903459910376,0.218834197757721,
-1.50710682163704));
#68137=CARTESIAN_POINT('Ctrl Pts',(0.100223506659529,0.215150811543088,
-1.50768345774627));
#68138=CARTESIAN_POINT('Ctrl Pts',(0.110253014288989,0.210002425457461,
-1.50841895791524));
#68139=CARTESIAN_POINT('Ctrl Pts',(0.112181125593001,0.208978803699889,
-1.50856226209941));
#68140=CARTESIAN_POINT('Ctrl Pts',(0.115239777492522,0.207300458425837,
-1.50879280621596));
#68141=CARTESIAN_POINT('Ctrl Pts',(0.116379544375256,0.20666273954255,-1.50887944048197));
#68142=CARTESIAN_POINT('Ctrl Pts',(0.118532482574293,0.205434676003937,
-1.5090444987553));
#68143=CARTESIAN_POINT('Ctrl Pts',(0.119546659596171,0.2048461657544,-1.50912285485526));
#68144=CARTESIAN_POINT('Ctrl Pts',(0.121847453205156,0.203488147631162,
-1.50930201760913));
#68145=CARTESIAN_POINT('Ctrl Pts',(0.123131210386247,0.202713918930156,
-1.5094029938949));
#68146=CARTESIAN_POINT('Ctrl Pts',(0.127067824261604,0.20028857249091,-1.5097158215292));
#68147=CARTESIAN_POINT('Ctrl Pts',(0.129695365667227,0.198597217335201,
-1.50992914111335));
#68148=CARTESIAN_POINT('Ctrl Pts',(0.146936313427526,0.187011091402289,
-1.5113599349279));
#68149=CARTESIAN_POINT('Ctrl Pts',(0.16043696772387,0.175565323953528,-1.51263755909178));
#68150=CARTESIAN_POINT('Ctrl Pts',(0.175572283406681,0.159517615244273,
-1.51424869033332));
#68151=CARTESIAN_POINT('Ctrl Pts',(0.178512991741656,0.156219745690236,
-1.51457135617857));
#68152=CARTESIAN_POINT('Ctrl Pts',(0.185527952185885,0.147895884524635,
-1.51536272525409));
#68153=CARTESIAN_POINT('Ctrl Pts',(0.189492239776667,0.142781357474674,
-1.51582944268662));
#68154=CARTESIAN_POINT('Ctrl Pts',(0.195350747418637,0.134548451101161,
-1.51654423959651));
#68155=CARTESIAN_POINT('Ctrl Pts',(0.197390525903791,0.13153776670685,-1.51679845436004));
#68156=CARTESIAN_POINT('Ctrl Pts',(0.199962526085301,0.127546870855848,
-1.51712502622282));
#68157=CARTESIAN_POINT('Ctrl Pts',(0.200558092893519,0.126608323585253,
-1.51720109263065));
#68158=CARTESIAN_POINT('Ctrl Pts',(0.201520094992038,0.125068491788823,
-1.5173246533053));
#68159=CARTESIAN_POINT('Ctrl Pts',(0.201890481526255,0.124469714493431,
-1.51737239823772));
#68160=CARTESIAN_POINT('Ctrl Pts',(0.202609413532483,0.123295816597441,
-1.51746539792279));
#68161=CARTESIAN_POINT('Ctrl Pts',(0.202958187220563,0.122720850307326,
-1.51751066656476));
#68162=CARTESIAN_POINT('Ctrl Pts',(0.203734434947989,0.121428816742796,
-1.51761177938801));
#68163=CARTESIAN_POINT('Ctrl Pts',(0.204160582396517,0.120710952970522,
-1.51766753856944));
#68164=CARTESIAN_POINT('Ctrl Pts',(0.205635769817062,0.118195776179702,
-1.51786149435082));
#68165=CARTESIAN_POINT('Ctrl Pts',(0.206664974130446,0.116386857200065,
-1.51799849156476));
#68166=CARTESIAN_POINT('Ctrl Pts',(0.213470861231888,0.104049878128328,
-1.51891768698643));
#68167=CARTESIAN_POINT('Ctrl Pts',(0.218465283812093,0.0931084284711445,
-1.51965951824881));
#68168=CARTESIAN_POINT('Ctrl Pts',(0.226270439510772,0.0718764945556738,
-1.52104825062062));
#68169=CARTESIAN_POINT('Ctrl Pts',(0.229258777445018,0.0616842518846413,
-1.521694626286));
#68170=CARTESIAN_POINT('Ctrl Pts',(0.233593252141522,0.0421296923970143,
-1.52294183886079));
#68171=CARTESIAN_POINT('Ctrl Pts',(0.23508189421692,0.0328205675152876,
-1.52353846344611));
#68172=CARTESIAN_POINT('Ctrl Pts',(0.236230919693698,0.0212553478775441,
-1.52429652331921));
#68173=CARTESIAN_POINT('Ctrl Pts',(0.236418214008599,0.0190595062975572,
-1.52444117003284));
#68174=CARTESIAN_POINT('Ctrl Pts',(0.236668049534541,0.0155541808922851,
-1.52467336389789));
#68175=CARTESIAN_POINT('Ctrl Pts',(0.236750382950365,0.0142462019333863,
-1.5247602897569));
#68176=CARTESIAN_POINT('Ctrl Pts',(0.236885784910824,0.0117676841364564,
-1.52492557731148));
#68177=CARTESIAN_POINT('Ctrl Pts',(0.236941027771759,0.0105972994782463,
-1.5250038683533));
#68178=CARTESIAN_POINT('Ctrl Pts',(0.237046865842675,0.00793649006466121,
-1.52518242763867));
#68179=CARTESIAN_POINT('Ctrl Pts',(0.237092080224086,0.00644591331735392,
-1.52528286127322));
#68180=CARTESIAN_POINT('Ctrl Pts',(0.23718764657318,0.00187258819260197,
-1.52559230238027));
#68181=CARTESIAN_POINT('Ctrl Pts',(0.2371919453507,-0.0012106913590628,
-1.52580273245632));
#68182=CARTESIAN_POINT('Ctrl Pts',(0.236806234750191,-0.0225162407726303,
-1.527269971454));
#68183=CARTESIAN_POINT('Ctrl Pts',(0.234376900259723,-0.0406373752304413,
-1.52859150064718));
#68184=CARTESIAN_POINT('Ctrl Pts',(0.22896645522489,-0.061973566132968,
-1.53019910913681));
#68185=CARTESIAN_POINT('Ctrl Pts',(0.227946326950483,-0.0656264670646265,
-1.53047594671459));
#68186=CARTESIAN_POINT('Ctrl Pts',(0.224927617249713,-0.075514234110407,
-1.53122771618989));
#68187=CARTESIAN_POINT('Ctrl Pts',(0.222757672168899,-0.0816937182181737,
-1.53170025811718));
#68188=CARTESIAN_POINT('Ctrl Pts',(0.218978401871383,-0.0911804290418259,
-1.53242279915932));
#68189=CARTESIAN_POINT('Ctrl Pts',(0.217543290257257,-0.0945533269945362,
-1.53267907896747));
#68190=CARTESIAN_POINT('Ctrl Pts',(0.215570433643927,-0.0989070834577553,
-1.53300787107483));
#68191=CARTESIAN_POINT('Ctrl Pts',(0.215103218492084,-0.0999191099715619,
-1.5330841536173));
#68192=CARTESIAN_POINT('Ctrl Pts',(0.214328977921189,-0.101565577377538,
-1.53320797614158));
#68193=CARTESIAN_POINT('Ctrl Pts',(0.214026235303011,-0.102201995674903,
-1.53325576874724));
#68194=CARTESIAN_POINT('Ctrl Pts',(0.213429278224202,-0.103442618959504,
-1.53334878576498));
#68195=CARTESIAN_POINT('Ctrl Pts',(0.213135326267643,-0.104046936208847,
-1.53339402457898));
#68196=CARTESIAN_POINT('Ctrl Pts',(0.212471230250406,-0.105397585044266,
-1.53349499276515));
#68197=CARTESIAN_POINT('Ctrl Pts',(0.212099710721139,-0.106143239923163,
-1.53355063792639));
#68198=CARTESIAN_POINT('Ctrl Pts',(0.210791007509068,-0.108735551334171,
-1.53374380830403));
#68199=CARTESIAN_POINT('Ctrl Pts',(0.209833541761557,-0.11057194236618,
-1.53388014681627));
#68200=CARTESIAN_POINT('Ctrl Pts',(0.203085872677736,-0.123110373508932,
-1.53480918671718));
#68201=CARTESIAN_POINT('Ctrl Pts',(0.19650285113427,-0.133366943993421,
-1.53556035353904));
#68202=CARTESIAN_POINT('Ctrl Pts',(0.182590932122008,-0.1517601579827,-1.53697586876211));
#68203=CARTESIAN_POINT('Ctrl Pts',(0.175430635886981,-0.159983361572266,
-1.53763945189577));
#68204=CARTESIAN_POINT('Ctrl Pts',(0.161339378743874,-0.174078463899533,
-1.53888251345984));
#68205=CARTESIAN_POINT('Ctrl Pts',(0.154588207765221,-0.18010042785522,
-1.53945596483905));
#68206=CARTESIAN_POINT('Ctrl Pts',(0.145803708159033,-0.187077549739037,
-1.54018786886537));
#68207=CARTESIAN_POINT('Ctrl Pts',(0.144078460705597,-0.188409467834584,
-1.54033095246942));
#68208=CARTESIAN_POINT('Ctrl Pts',(0.141291031214913,-0.190500732117462,
-1.54056122553606));
#68209=CARTESIAN_POINT('Ctrl Pts',(0.140240483022783,-0.191275432936191,
-1.54064781188387));
#68210=CARTESIAN_POINT('Ctrl Pts',(0.138234060436025,-0.192729604417816,
-1.54081283297547));
#68211=CARTESIAN_POINT('Ctrl Pts',(0.13727943361882,-0.193410736268062,
-1.54089120026589));
#68212=CARTESIAN_POINT('Ctrl Pts',(0.135091941419078,-0.194947170837933,
-1.54107046462445));
#68213=CARTESIAN_POINT('Ctrl Pts',(0.133855942349463,-0.19579790236774,
-1.54117153203704));
#68214=CARTESIAN_POINT('Ctrl Pts',(0.130015561772675,-0.198387856963129,
-1.54148493060846));
#68215=CARTESIAN_POINT('Ctrl Pts',(0.127384832963406,-0.20008720796019,
-1.54169873776807));
#68216=CARTESIAN_POINT('Ctrl Pts',(0.109811136979919,-0.21095208871016,
-1.54312195639264));
#68217=CARTESIAN_POINT('Ctrl Pts',(0.0939276013892588,-0.218487195255883,
-1.54439061142367));
#68218=CARTESIAN_POINT('Ctrl Pts',(0.068147143198341,-0.227382903442695,
-1.54638245531063));
#68219=CARTESIAN_POINT('Ctrl Pts',(0.0587438344862851,-0.229991740195819,
-1.54709473150502));
#68220=CARTESIAN_POINT('Ctrl Pts',(0.0461340717715222,-0.232666049386161,
-1.54801334056481));
#68221=CARTESIAN_POINT('Ctrl Pts',(0.0430491433158123,-0.233256546300021,
-1.54823520428722));
#68222=CARTESIAN_POINT('Ctrl Pts',(0.0378060564099866,-0.234152573755792,
-1.54860647990618));
#68223=CARTESIAN_POINT('Ctrl Pts',(0.0356538164773341,-0.234489939900515,
-1.54875724269302));
#68224=CARTESIAN_POINT('Ctrl Pts',(0.0325908839470168,-0.234926909750811,
-1.5489691880057));
#68225=CARTESIAN_POINT('Ctrl Pts',(0.0316838675929623,-0.235050954573529,
-1.54903162666025));
#68226=CARTESIAN_POINT('Ctrl Pts',(0.0301167676648912,-0.235256037423696,
-1.54913892006547));
#68227=CARTESIAN_POINT('Ctrl Pts',(0.0294570265270114,-0.235339555691331,
-1.54918391079166));
#68228=CARTESIAN_POINT('Ctrl Pts',(0.0280675509064115,-0.235509518174503,
-1.54927827972268));
#68229=CARTESIAN_POINT('Ctrl Pts',(0.0273377581672127,-0.235595347110625,
-1.54932762371291));
#68230=CARTESIAN_POINT('Ctrl Pts',(0.0253645571366234,-0.235818117688735,
-1.54946047020111));
#68231=CARTESIAN_POINT('Ctrl Pts',(0.0241204238724349,-0.235948618795346,
-1.54954362216039));
#68232=CARTESIAN_POINT('Ctrl Pts',(0.01829072215585,-0.23651352109108,-1.54993064505786));
#68233=CARTESIAN_POINT('Ctrl Pts',(0.0136938250253303,-0.236824158474367,
-1.5502282873018));
#68234=CARTESIAN_POINT('Ctrl Pts',(0.00594124313793845,-0.237121518081253,
-1.55072196631789));
#68235=CARTESIAN_POINT('Ctrl Pts',(0.0027898263478255,-0.237179533316197,
-1.55092034567002));
#68236=CARTESIAN_POINT('Ctrl Pts',(-0.0146548208244471,-0.237152913396436,
-1.55201020544053));
#68237=CARTESIAN_POINT('Ctrl Pts',(-0.0289168759591554,-0.235839170098116,
-1.55287223014267));
#68238=CARTESIAN_POINT('Ctrl Pts',(-0.0530798299700456,-0.231387338564605,
-1.55439224574075));
#68239=CARTESIAN_POINT('Ctrl Pts',(-0.0630525803721703,-0.228870933593862,
-1.55503743737435));
#68240=CARTESIAN_POINT('Ctrl Pts',(-0.0755404455863732,-0.22484157278426,
-1.55588788112081));
#68241=CARTESIAN_POINT('Ctrl Pts',(-0.0782347820119654,-0.223918309924308,
-1.55607393214493));
#68242=CARTESIAN_POINT('Ctrl Pts',(-0.0822704737345905,-0.222453678469284,
-1.55635681147324));
#68243=CARTESIAN_POINT('Ctrl Pts',(-0.0836246361951811,-0.221948169576309,
-1.55645245293647));
#68244=CARTESIAN_POINT('Ctrl Pts',(-0.0860641264696326,-0.221012013180196,
-1.55662609951111));
#68245=CARTESIAN_POINT('Ctrl Pts',(-0.087151063484527,-0.220585665637363,
-1.55670395854886));
#68246=CARTESIAN_POINT('Ctrl Pts',(-0.0894790927337202,-0.219652611139689,
-1.55687179493788));
#68247=CARTESIAN_POINT('Ctrl Pts',(-0.090719120556606,-0.219143374652647,
-1.55696185549327));
#68248=CARTESIAN_POINT('Ctrl Pts',(-0.0940580904649978,-0.217738979005214,
-1.557206188833));
#68249=CARTESIAN_POINT('Ctrl Pts',(-0.096148494384201,-0.216824015627731,
-1.55736112852527));
#68250=CARTESIAN_POINT('Ctrl Pts',(-0.10731839960784,-0.211741691327165,
-1.5581999606161));
#68251=CARTESIAN_POINT('Ctrl Pts',(-0.116139746961318,-0.207034521989676,
-1.55890224612895));
#68252=CARTESIAN_POINT('Ctrl Pts',(-0.139098352316603,-0.192853676827186,
-1.56083835176652));
#68253=CARTESIAN_POINT('Ctrl Pts',(-0.152556285958983,-0.182393573845782,
-1.56209687960328));
#68254=CARTESIAN_POINT('Ctrl Pts',(-0.169206965890734,-0.166309540009794,
-1.56376022108362));
#68255=CARTESIAN_POINT('Ctrl Pts',(-0.173465964134562,-0.161862393558947,
-1.56419637674309));
#68256=CARTESIAN_POINT('Ctrl Pts',(-0.178417386678673,-0.156272000504373,
-1.56471180321978));
#68257=CARTESIAN_POINT('Ctrl Pts',(-0.179279153207211,-0.155282605059267,
-1.56480183471092));
#68258=CARTESIAN_POINT('Ctrl Pts',(-0.180619405019962,-0.153717829017834,
-1.56494230011409));
#68259=CARTESIAN_POINT('Ctrl Pts',(-0.181103437612204,-0.153147266877444,
-1.5649931222925));
#68260=CARTESIAN_POINT('Ctrl Pts',(-0.182010081172323,-0.152068234956686,
-1.56508847810162));
#68261=CARTESIAN_POINT('Ctrl Pts',(-0.182433263737258,-0.151560291716579,
-1.56513305107814));
#68262=CARTESIAN_POINT('Ctrl Pts',(-0.183410460061543,-0.150377346263434,
-1.56523614049781));
#68263=CARTESIAN_POINT('Ctrl Pts',(-0.183962876694107,-0.149701046049113,
-1.56529454246618));
#68264=CARTESIAN_POINT('Ctrl Pts',(-0.185760914361094,-0.147474801579748,
-1.56548510269854));
#68265=CARTESIAN_POINT('Ctrl Pts',(-0.186990820523314,-0.145912193070795,
-1.56561619996631));
#68266=CARTESIAN_POINT('Ctrl Pts',(-0.197781627399318,-0.131841793500857,
-1.56677507184123));
#68267=CARTESIAN_POINT('Ctrl Pts',(-0.206096087345197,-0.11842456948595,
-1.56773162403626));
#68268=CARTESIAN_POINT('Ctrl Pts',(-0.219863767401986,-0.0903005080396204,
-1.56965120240518));
#68269=CARTESIAN_POINT('Ctrl Pts',(-0.225313796306159,-0.075682661650732,
-1.57061036730523));
#68270=CARTESIAN_POINT('Ctrl Pts',(-0.229994294282153,-0.0579839484923982,
-1.57179800862275));
#68271=CARTESIAN_POINT('Ctrl Pts',(-0.230649866709464,-0.0553186374757089,
-1.57197743184894));
#68272=CARTESIAN_POINT('Ctrl Pts',(-0.231575232285671,-0.051253508068792,
-1.57225223798412));
#68273=CARTESIAN_POINT('Ctrl Pts',(-0.23187891798976,-0.0498615838088404,
-1.57234653568833));
#68274=CARTESIAN_POINT('Ctrl Pts',(-0.232408381862603,-0.0473253103862923,
-1.57251876537644));
#68275=CARTESIAN_POINT('Ctrl Pts',(-0.232638295266252,-0.0461818628381915,
-1.5725965625038));
#68276=CARTESIAN_POINT('Ctrl Pts',(-0.233117358477165,-0.0437048976327094,
-1.57276543351551));
#68277=CARTESIAN_POINT('Ctrl Pts',(-0.23336351846313,-0.0423708510422573,
-1.57285659970519));
#68278=CARTESIAN_POINT('Ctrl Pts',(-0.234005308331653,-0.0387173421779607,
-1.57310689861532));
#68279=CARTESIAN_POINT('Ctrl Pts',(-0.234377878661777,-0.0363940408689096,
-1.57326675419077));
#68280=CARTESIAN_POINT('Ctrl Pts',(-0.236363365187718,-0.0227138366397453,
-1.57421235800029));
#68281=CARTESIAN_POINT('Ctrl Pts',(-0.237184984577307,-0.0112592180260812,
-1.57502272257575));
#68282=CARTESIAN_POINT('Ctrl Pts',(-0.23716687031361,0.00935657934971425,
-1.57650990145017));
#68283=CARTESIAN_POINT('Ctrl Pts',(-0.236629549187816,0.0184963197536797,
-1.57717907270038));
#68284=CARTESIAN_POINT('Ctrl Pts',(-0.235383558988599,0.0291378701453599,
-1.57796111466374));
#68285=CARTESIAN_POINT('Ctrl Pts',(-0.235185941931456,0.0306921502255948,
-1.57807539920959));
#68286=CARTESIAN_POINT('Ctrl Pts',(-0.233547229905083,0.0426338639009862,
-1.57895353549401));
#68287=CARTESIAN_POINT('Ctrl Pts',(-0.231433839853078,0.0529186618183489,
-1.57971079543511));
#68288=CARTESIAN_POINT('Ctrl Pts',(-0.228286216710733,0.0643367624147382,
-1.58053060395141));
#68289=CARTESIAN_POINT('Ctrl Pts',(-0.227915013344541,0.0656396423157721,
-1.58062382745949));
#68290=CARTESIAN_POINT('Ctrl Pts',(-0.227296148252182,0.0677432197782579,
-1.58077374153251));
#68291=CARTESIAN_POINT('Ctrl Pts',(-0.227055376583825,0.0685458886798055,
-1.58083080232548));
#68292=CARTESIAN_POINT('Ctrl Pts',(-0.226618533964416,0.0699746459128448,
-1.58093209593542));
#68293=CARTESIAN_POINT('Ctrl Pts',(-0.226424114666178,0.070601213440327,
-1.58097642123452));
#68294=CARTESIAN_POINT('Ctrl Pts',(-0.225992505048857,0.0719720671855698,
-1.58107318730141));
#68295=CARTESIAN_POINT('Ctrl Pts',(-0.225754236262176,0.0727159930622962,
-1.58112556477085));
#68296=CARTESIAN_POINT('Ctrl Pts',(-0.225058363969718,0.0748522637399902,
-1.58127562100822));
#68297=CARTESIAN_POINT('Ctrl Pts',(-0.224591514746974,0.0762415920055359,
-1.58137277914787));
#68298=CARTESIAN_POINT('Ctrl Pts',(-0.220730747035128,0.0873878254732538,
-1.5821494529609));
#68299=CARTESIAN_POINT('Ctrl Pts',(-0.216715092128115,0.0969191430188302,
-1.58279647101808));
#68300=CARTESIAN_POINT('Ctrl Pts',(-0.204803838991282,0.120716014100129,
-1.58443989603002));
#68301=CARTESIAN_POINT('Ctrl Pts',(-0.196038712819069,0.134483387828047,
-1.58542126925986));
#68302=CARTESIAN_POINT('Ctrl Pts',(-0.181754083713967,0.152521272843102,
-1.58687176305908));
#68303=CARTESIAN_POINT('Ctrl Pts',(-0.177352977769336,0.157617238544378,
-1.58730254230416));
#68304=CARTESIAN_POINT('Ctrl Pts',(-0.171328868542365,0.164020270325979,
-1.58787687538116));
#68305=CARTESIAN_POINT('Ctrl Pts',(-0.169896817305636,0.165503176106197,
-1.58801234567089));
#68306=CARTESIAN_POINT('Ctrl Pts',(-0.167544802464842,0.167876017632505,
-1.58823326780594));
#68307=CARTESIAN_POINT('Ctrl Pts',(-0.166636625412965,0.168777525432041,
-1.58831820189973));
#68308=CARTESIAN_POINT('Ctrl Pts',(-0.164877514863053,0.170495679148747,
-1.58848203992736));
#68309=CARTESIAN_POINT('Ctrl Pts',(-0.164027695964611,0.17131341566146,
-1.58856089262049));
#68310=CARTESIAN_POINT('Ctrl Pts',(-0.162045594720039,0.173192419394738,
-1.58874414802871));
#68311=CARTESIAN_POINT('Ctrl Pts',(-0.160908935215939,0.174248969214105,
-1.5888487488674));
#68312=CARTESIAN_POINT('Ctrl Pts',(-0.157240902808065,0.177591989205021,
-1.58918480878934));
#68313=CARTESIAN_POINT('Ctrl Pts',(-0.154670638839328,0.179834945207608,
-1.58941806902809));
#68314=CARTESIAN_POINT('Ctrl Pts',(-0.148492258278884,0.184996098578095,
-1.5899739141462));
#68315=CARTESIAN_POINT('Ctrl Pts',(-0.144845210246446,0.187865290446729,
-1.59029829506591));
#68316=CARTESIAN_POINT('Ctrl Pts',(-0.12164429786254,0.205040499020205,
-1.59233907212551));
#68317=CARTESIAN_POINT('Ctrl Pts',(-0.100082369864355,0.216384358933479,
-1.59415771635204));
#68318=CARTESIAN_POINT('Ctrl Pts',(-0.0743544254437696,0.225238369261192,
-1.59607307737764));
#68319=CARTESIAN_POINT('Ctrl Pts',(-0.0715115974071082,0.226157018599424,
-1.59628118595296));
#68320=CARTESIAN_POINT('Ctrl Pts',(-0.0676290671327156,0.227331106576671,
-1.59655995328095));
#68321=CARTESIAN_POINT('Ctrl Pts',(-0.0666040160675047,0.227633538591691,
-1.59663304122716));
#68322=CARTESIAN_POINT('Ctrl Pts',(-0.0649756006170944,0.228102046198254,
-1.59674830317951));
#68323=CARTESIAN_POINT('Ctrl Pts',(-0.0643735785280153,0.228272675907759,
-1.59679073255126));
#68324=CARTESIAN_POINT('Ctrl Pts',(-0.0631210725835327,0.228622321690159,
-1.59687861727664));
#68325=CARTESIAN_POINT('Ctrl Pts',(-0.062470491743581,0.228800947231329,
-1.59692404765882));
#68326=CARTESIAN_POINT('Ctrl Pts',(-0.0608816579816892,0.229229900539494,
-1.59703448174924));
#68327=CARTESIAN_POINT('Ctrl Pts',(-0.0599425989567112,0.229477250490129,
-1.59709931591161));
#68328=CARTESIAN_POINT('Ctrl Pts',(-0.0565513129593959,0.230348283771568,
-1.59733197331986));
#68329=CARTESIAN_POINT('Ctrl Pts',(-0.0540905608930938,0.230938509841191,
-1.59749800523825));
#68330=CARTESIAN_POINT('Ctrl Pts',(-0.0484075384125142,0.232205789651432,
-1.59787606103081));
#68331=CARTESIAN_POINT('Ctrl Pts',(-0.0451796913467915,0.232855352832219,
-1.59808684124396));
#68332=CARTESIAN_POINT('Ctrl Pts',(-0.0419392741218017,0.233437524642326,
-1.59829545246927));
#68333=CARTESIAN_POINT('Ctrl Pts',(-0.0419392757399419,0.233437524351611,
-1.61803181050061));
#68334=CARTESIAN_POINT('Ctrl Pts',(-0.0448253805600994,0.232919008118186,
-1.61782780117959));
#68335=CARTESIAN_POINT('Ctrl Pts',(-0.0477018253624859,0.232346976417747,
-1.61762220998104));
#68336=CARTESIAN_POINT('Ctrl Pts',(-0.0665627472268817,0.228231078868697,
-1.6162592909867));
#68337=CARTESIAN_POINT('Ctrl Pts',(-0.082152447815779,0.223093875629562,
-1.61505775634771));
#68338=CARTESIAN_POINT('Ctrl Pts',(-0.106545044553912,0.21214995997301,
-1.6131106274145));
#68339=CARTESIAN_POINT('Ctrl Pts',(-0.11571631766398,0.207290224297602,
-1.61236257754996));
#68340=CARTESIAN_POINT('Ctrl Pts',(-0.125788627065247,0.201075485959217,
-1.61154380133823));
#68341=CARTESIAN_POINT('Ctrl Pts',(-0.127029118554178,0.200294116399598,
-1.61144302152065));
#68342=CARTESIAN_POINT('Ctrl Pts',(-0.12891931375671,0.199078881886963,
-1.61128964454322));
#68343=CARTESIAN_POINT('Ctrl Pts',(-0.129574225193482,0.198653242819663,
-1.61123653742812));
#68344=CARTESIAN_POINT('Ctrl Pts',(-0.130775130330684,0.197864286774164,
-1.6111392367465));
#68345=CARTESIAN_POINT('Ctrl Pts',(-0.131321721560386,0.19750193963529,
-1.61109498355794));
#68346=CARTESIAN_POINT('Ctrl Pts',(-0.132562871229332,0.196671724079642,
-1.61099456702984));
#68347=CARTESIAN_POINT('Ctrl Pts',(-0.1332564603171,0.196202440654019,-1.61093849929123));
#68348=CARTESIAN_POINT('Ctrl Pts',(-0.135064330725534,0.194965223710152,
-1.61079244056339));
#68349=CARTESIAN_POINT('Ctrl Pts',(-0.136174569437207,0.194191397179468,
-1.61070282827568));
#68350=CARTESIAN_POINT('Ctrl Pts',(-0.145680592230037,0.187444165012068,
-1.60993571367215));
#68351=CARTESIAN_POINT('Ctrl Pts',(-0.153686614280069,0.180938195371603,
-1.60929050051278));
#68352=CARTESIAN_POINT('Ctrl Pts',(-0.16874719762037,0.166976111990685,
-1.60802234707679));
#68353=CARTESIAN_POINT('Ctrl Pts',(-0.175791676964131,0.159542875115537,
-1.60740046339865));
#68354=CARTESIAN_POINT('Ctrl Pts',(-0.18753428391113,0.145426919488356,
-1.60626780584322));
#68355=CARTESIAN_POINT('Ctrl Pts',(-0.192409057189505,0.138913050417115,
-1.60576128509703));
#68356=CARTESIAN_POINT('Ctrl Pts',(-0.198858253472461,0.129302871034174,
-1.60502410889906));
#68357=CARTESIAN_POINT('Ctrl Pts',(-0.200714446697319,0.126402320015458,
-1.60480288118514));
#68358=CARTESIAN_POINT('Ctrl Pts',(-0.203917010455068,0.12114938193312,
-1.60440363483024));
#68359=CARTESIAN_POINT('Ctrl Pts',(-0.205287464014855,0.118812356395178,
-1.60422649127343));
#68360=CARTESIAN_POINT('Ctrl Pts',(-0.207313357874855,0.115217883051229,
-1.60395448549345));
#68361=CARTESIAN_POINT('Ctrl Pts',(-0.207998081739118,0.11397713267939,
-1.60386067466868));
#68362=CARTESIAN_POINT('Ctrl Pts',(-0.209171918164477,0.111804280567195,
-1.60369649279287));
#68363=CARTESIAN_POINT('Ctrl Pts',(-0.209666026095908,0.110874911235665,
-1.60362630179277));
#68364=CARTESIAN_POINT('Ctrl Pts',(-0.2107661005386,0.108772126692896,-1.60346754451242));
#68365=CARTESIAN_POINT('Ctrl Pts',(-0.211368481142887,0.107596885356162,
-1.60337885460028));
#68366=CARTESIAN_POINT('Ctrl Pts',(-0.212971215415024,0.104404555737766,
-1.60313801571861));
#68367=CARTESIAN_POINT('Ctrl Pts',(-0.213952691199311,0.102378196763698,
-1.60298521615846));
#68368=CARTESIAN_POINT('Ctrl Pts',(-0.218720926029562,0.092165557337005,
-1.6022152621633));
#68369=CARTESIAN_POINT('Ctrl Pts',(-0.222066930649408,0.083782906557399,
-1.60158330450425));
#68370=CARTESIAN_POINT('Ctrl Pts',(-0.225095352756358,0.074728465753995,
-1.60090108818646));
#68371=CARTESIAN_POINT('Ctrl Pts',(-0.225261751686517,0.0742253639108846,
-1.60086318421204));
#68372=CARTESIAN_POINT('Ctrl Pts',(-0.230857472539021,0.0571147524739912,
-1.5995741765043));
#68373=CARTESIAN_POINT('Ctrl Pts',(-0.234436308771632,0.0399601541125883,
-1.59827993360627));
#68374=CARTESIAN_POINT('Ctrl Pts',(-0.236690627417089,0.0163772768627074,
-1.59657726251572));
#68375=CARTESIAN_POINT('Ctrl Pts',(-0.237038764327972,0.0101640384228324,
-1.59613634377581));
#68376=CARTESIAN_POINT('Ctrl Pts',(-0.23716408303571,0.00262845668443124,
-1.59561614313132));
#68377=CARTESIAN_POINT('Ctrl Pts',(-0.23717501418411,0.00131297859049132,
-1.59552587121188));
#68378=CARTESIAN_POINT('Ctrl Pts',(-0.237174991904851,-0.000751352849641178,
-1.5953851263894));
#68379=CARTESIAN_POINT('Ctrl Pts',(-0.237171437763164,-0.00150015495153717,
-1.59533426257375));
#68380=CARTESIAN_POINT('Ctrl Pts',(-0.237158072402004,-0.00290961275161045,
-1.59523889401));
#68381=CARTESIAN_POINT('Ctrl Pts',(-0.237149047112992,-0.00357024049217805,
-1.59519434940052));
#68382=CARTESIAN_POINT('Ctrl Pts',(-0.237121444682551,-0.0051173458443599,
-1.5950903844646));
#68383=CARTESIAN_POINT('Ctrl Pts',(-0.237100657091772,-0.00600376772102378,
-1.59503108710061));
#68384=CARTESIAN_POINT('Ctrl Pts',(-0.237016452093551,-0.00890111005079207,
-1.59483809002992));
#68385=CARTESIAN_POINT('Ctrl Pts',(-0.236932416881283,-0.0109114076643369,
-1.59470547402414));
#68386=CARTESIAN_POINT('Ctrl Pts',(-0.236668833765064,-0.0157426928009187,
-1.59438934917823));
#68387=CARTESIAN_POINT('Ctrl Pts',(-0.236464416753113,-0.018562067842114,
-1.59420699295673));
#68388=CARTESIAN_POINT('Ctrl Pts',(-0.235474923760893,-0.0294955531655902,
-1.59350574820215));
#68389=CARTESIAN_POINT('Ctrl Pts',(-0.234322107712655,-0.0375712313196251,
-1.59300039577045));
#68390=CARTESIAN_POINT('Ctrl Pts',(-0.22889712927067,-0.0652788779971918,
-1.59126346106171));
#68391=CARTESIAN_POINT('Ctrl Pts',(-0.222552201560954,-0.0844136581320735,
-1.59005069501236));
#68392=CARTESIAN_POINT('Ctrl Pts',(-0.212643298963519,-0.105085206262819,
-1.5885654089827));
#68393=CARTESIAN_POINT('Ctrl Pts',(-0.211367639957468,-0.107628029890246,
-1.58837962913555));
#68394=CARTESIAN_POINT('Ctrl Pts',(-0.209367015345032,-0.111443146026963,
-1.58809587933566));
#68395=CARTESIAN_POINT('Ctrl Pts',(-0.208675467580815,-0.112732741380211,
-1.58799908163612));
#68396=CARTESIAN_POINT('Ctrl Pts',(-0.207410266440159,-0.115040547801208,
-1.58782421671853));
#68397=CARTESIAN_POINT('Ctrl Pts',(-0.206840932332536,-0.116061082585927,
-1.58774630536856));
#68398=CARTESIAN_POINT('Ctrl Pts',(-0.20560892914254,-0.118231596427108,
-1.58757932528566));
#68399=CARTESIAN_POINT('Ctrl Pts',(-0.204944104820854,-0.119380299512177,
-1.58749018082305));
#68400=CARTESIAN_POINT('Ctrl Pts',(-0.203110067364868,-0.122488728537328,
-1.58724680480496));
#68401=CARTESIAN_POINT('Ctrl Pts',(-0.201922181019589,-0.124437214131901,
-1.58709189903665));
#68402=CARTESIAN_POINT('Ctrl Pts',(-0.194920244012957,-0.135558157436927,
-1.58619386269258));
#68403=CARTESIAN_POINT('Ctrl Pts',(-0.188510613607033,-0.144338498989121,
-1.58542872498265));
#68404=CARTESIAN_POINT('Ctrl Pts',(-0.171594242740078,-0.164454793572754,
-1.58353752637507));
#68405=CARTESIAN_POINT('Ctrl Pts',(-0.160537939460671,-0.175264077918458,
-1.58239798684725));
#68406=CARTESIAN_POINT('Ctrl Pts',(-0.143248817321769,-0.189148893207022,
-1.58079981652409));
#68407=CARTESIAN_POINT('Ctrl Pts',(-0.137808277619231,-0.193148711075333,
-1.58031993437694));
#68408=CARTESIAN_POINT('Ctrl Pts',(-0.131056535695983,-0.197681752515671,
-1.57975789585834));
#68409=CARTESIAN_POINT('Ctrl Pts',(-0.129902318587938,-0.198442129299966,
-1.57966294943602));
#68410=CARTESIAN_POINT('Ctrl Pts',(-0.128093480546965,-0.199611212575235,
-1.57951599193981));
#68411=CARTESIAN_POINT('Ctrl Pts',(-0.12744342321421,-0.200026872861384,
-1.5794635441475));
#68412=CARTESIAN_POINT('Ctrl Pts',(-0.126236318509734,-0.200790447536555,
-1.57936684427133));
#68413=CARTESIAN_POINT('Ctrl Pts',(-0.125679854786443,-0.201139220568089,
-1.57932253826151));
#68414=CARTESIAN_POINT('Ctrl Pts',(-0.124399705473633,-0.201934188927431,
-1.57922122609034));
#68415=CARTESIAN_POINT('Ctrl Pts',(-0.123675063128399,-0.202378808663552,
-1.57916432263383));
#68416=CARTESIAN_POINT('Ctrl Pts',(-0.121398418630204,-0.203758897447544,
-1.57898688478273));
#68417=CARTESIAN_POINT('Ctrl Pts',(-0.11983803264698,-0.204680508985244,
-1.57886720641069));
#68418=CARTESIAN_POINT('Ctrl Pts',(-0.116131029040646,-0.206813050795847,
-1.57858704707638));
#68419=CARTESIAN_POINT('Ctrl Pts',(-0.113975763673021,-0.208008606116302,
-1.57842739937182));
#68420=CARTESIAN_POINT('Ctrl Pts',(-0.106032497992382,-0.212254303865473,
-1.57784928952455));
#68421=CARTESIAN_POINT('Ctrl Pts',(-0.100137269307851,-0.215098395725834,
-1.57743983747774));
#68422=CARTESIAN_POINT('Ctrl Pts',(-0.0906152336394982,-0.21921573080034,
-1.57679757205473));
#68423=CARTESIAN_POINT('Ctrl Pts',(-0.0870624959189503,-0.220650810132163,
-1.57656199791734));
#68424=CARTESIAN_POINT('Ctrl Pts',(-0.0664526318686506,-0.228400563924269,
-1.57521088632839));
#68425=CARTESIAN_POINT('Ctrl Pts',(-0.0487510743039558,-0.232821857679894,
-1.57410482193531));
#68426=CARTESIAN_POINT('Ctrl Pts',(-0.0276591421225758,-0.235576897961391,
-1.57272912428341));
#68427=CARTESIAN_POINT('Ctrl Pts',(-0.0245919141816058,-0.235916805928248,
-1.57252784560778));
#68428=CARTESIAN_POINT('Ctrl Pts',(-0.0200337176549391,-0.23633208684842,
-1.57222650997896));
#68429=CARTESIAN_POINT('Ctrl Pts',(-0.0185471820476079,-0.236453392837338,
-1.57212788994346));
#68430=CARTESIAN_POINT('Ctrl Pts',(-0.0158912994391405,-0.236644922448308,
-1.57195102838453));
#68431=CARTESIAN_POINT('Ctrl Pts',(-0.0147223798344311,-0.236720519106242,
-1.57187295789503));
#68432=CARTESIAN_POINT('Ctrl Pts',(-0.0122454224141728,-0.236862292326132,
-1.57170701771441));
#68433=CARTESIAN_POINT('Ctrl Pts',(-0.0109373047304288,-0.236926298966222,
-1.57161908269013));
#68434=CARTESIAN_POINT('Ctrl Pts',(-0.00742955300061291,-0.237068822926058,
-1.57138244668804));
#68435=CARTESIAN_POINT('Ctrl Pts',(-0.00522928954504909,-0.237127558546657,
-1.57123313346676));
#68436=CARTESIAN_POINT('Ctrl Pts',(0.00635404935427809,-0.237275483284894,
-1.57044220184766));
#68437=CARTESIAN_POINT('Ctrl Pts',(0.0157342978430609,-0.236838383638481,
-1.56978439981627));
#68438=CARTESIAN_POINT('Ctrl Pts',(0.0356405595703932,-0.234722984347898,
-1.56835247685168));
#68439=CARTESIAN_POINT('Ctrl Pts',(0.0461298632089687,-0.232888676800962,
-1.56757600914355));
#68440=CARTESIAN_POINT('Ctrl Pts',(0.0681396971986026,-0.227494122084667,
-1.56592107634686));
#68441=CARTESIAN_POINT('Ctrl Pts',(0.0795860880552203,-0.223746969316612,
-1.56504477648228));
#68442=CARTESIAN_POINT('Ctrl Pts',(0.0926216159837324,-0.218351878931473,
-1.56406058919018));
#68443=CARTESIAN_POINT('Ctrl Pts',(0.0945329973376726,-0.21753119301078,
-1.56391666796137));
#68444=CARTESIAN_POINT('Ctrl Pts',(0.0971957780596239,-0.21634615241026,
-1.56371695962002));
#68445=CARTESIAN_POINT('Ctrl Pts',(0.0979563604836231,-0.216002843566867,
-1.56366000744057));
#68446=CARTESIAN_POINT('Ctrl Pts',(0.0993263524834753,-0.215375737259282,
-1.56355760905645));
#68447=CARTESIAN_POINT('Ctrl Pts',(0.0999363962822983,-0.215093350050745,
-1.56351207923177));
#68448=CARTESIAN_POINT('Ctrl Pts',(0.101182695938329,-0.214509995189509,
-1.56341921294));
#68449=CARTESIAN_POINT('Ctrl Pts',(0.101818825764001,-0.214208783075014,
-1.5633718919076));
#68450=CARTESIAN_POINT('Ctrl Pts',(0.103455764355276,-0.21342474117569,
-1.56325030255618));
#68451=CARTESIAN_POINT('Ctrl Pts',(0.104454551882658,-0.21293769519829,
-1.56317628922051));
#68452=CARTESIAN_POINT('Ctrl Pts',(0.108705700198137,-0.210827567588547,
-1.56286185872002));
#68453=CARTESIAN_POINT('Ctrl Pts',(0.111924134523603,-0.209136759408554,
-1.56262530115006));
#68454=CARTESIAN_POINT('Ctrl Pts',(0.12075580255814,-0.204234720056343,
-1.56197679227005));
#68455=CARTESIAN_POINT('Ctrl Pts',(0.126278718686508,-0.200866826557076,
-1.56157193052418));
#68456=CARTESIAN_POINT('Ctrl Pts',(0.135330607630634,-0.194825841464226,
-1.56089792181914));
#68457=CARTESIAN_POINT('Ctrl Pts',(0.138934652818485,-0.19227232145599,
-1.5606265955807));
#68458=CARTESIAN_POINT('Ctrl Pts',(0.156578725015797,-0.179015944720803,
-1.55927307059438));
#68459=CARTESIAN_POINT('Ctrl Pts',(0.16946248981502,-0.166871163373313,
-1.55819737168683));
#68460=CARTESIAN_POINT('Ctrl Pts',(0.182899899045689,-0.151027702305313,
-1.55685423620292));
#68461=CARTESIAN_POINT('Ctrl Pts',(0.184873215905236,-0.148605627382765,
-1.5566505173462));
#68462=CARTESIAN_POINT('Ctrl Pts',(0.187721544500754,-0.144964990623914,
-1.55634623056634));
#68463=CARTESIAN_POINT('Ctrl Pts',(0.188633814498065,-0.143775904207863,
-1.55624714174698));
#68464=CARTESIAN_POINT('Ctrl Pts',(0.190239387617031,-0.141641554640548,
-1.55606976006927));
#68465=CARTESIAN_POINT('Ctrl Pts',(0.190937073792697,-0.140699638836436,
-1.55599164215179));
#68466=CARTESIAN_POINT('Ctrl Pts',(0.192397013132775,-0.138697780799072,
-1.55582593792496));
#68467=CARTESIAN_POINT('Ctrl Pts',(0.193157551384084,-0.13763664223583,
-1.55573828879223));
#68468=CARTESIAN_POINT('Ctrl Pts',(0.195165666785093,-0.134785399572777,
-1.55550324171146));
#68469=CARTESIAN_POINT('Ctrl Pts',(0.196397341691543,-0.132984303776592,
-1.55535524576509));
#68470=CARTESIAN_POINT('Ctrl Pts',(0.202627891522382,-0.123597904885718,
-1.55458620003902));
#68471=CARTESIAN_POINT('Ctrl Pts',(0.207212204733981,-0.115747870474028,
-1.55395003284956));
#68472=CARTESIAN_POINT('Ctrl Pts',(0.216257954015978,-0.0979904267812124,
-1.55252639588848));
#68473=CARTESIAN_POINT('Ctrl Pts',(0.220512125623393,-0.0879999833909121,
-1.55173494670563));
#68474=CARTESIAN_POINT('Ctrl Pts',(0.228055491319261,-0.0662619916257181,
-1.55005451203028));
#68475=CARTESIAN_POINT('Ctrl Pts',(0.231153824412979,-0.0544786847534756,
-1.54916771819621));
#68476=CARTESIAN_POINT('Ctrl Pts',(0.233705691664736,-0.0404712150169731,
-1.54817455328728));
#68477=CARTESIAN_POINT('Ctrl Pts',(0.234050184699699,-0.0384289127149271,
-1.54803126360847));
#68478=CARTESIAN_POINT('Ctrl Pts',(0.234495665138618,-0.0355592100236386,
-1.54783228232833));
#68479=CARTESIAN_POINT('Ctrl Pts',(0.234619100103016,-0.0347354617892509,
-1.54777543639346));
#68480=CARTESIAN_POINT('Ctrl Pts',(0.234834249724351,-0.0332461592872965,
-1.54767317228876));
#68481=CARTESIAN_POINT('Ctrl Pts',(0.234927480781002,-0.0325808343269141,
-1.54762767117023));
#68482=CARTESIAN_POINT('Ctrl Pts',(0.235112675384859,-0.0312170900386859,
-1.54753479408695));
#68483=CARTESIAN_POINT('Ctrl Pts',(0.23520435644733,-0.0305186431263219,
-1.54748743403413));
#68484=CARTESIAN_POINT('Ctrl Pts',(0.235432975287881,-0.028714726930122,
-1.5473656252953));
#68485=CARTESIAN_POINT('Ctrl Pts',(0.235565241515327,-0.0276086672510516,
-1.54729143334992));
#68486=CARTESIAN_POINT('Ctrl Pts',(0.236098697966602,-0.0228644339758852,
-1.54697515882675));
#68487=CARTESIAN_POINT('Ctrl Pts',(0.23642345782649,-0.0192179523995993,
-1.54673699223175));
#68488=CARTESIAN_POINT('Ctrl Pts',(0.237092526549318,-0.0090449698864053,
-1.54608259769615));
#68489=CARTESIAN_POINT('Ctrl Pts',(0.237251750755394,-0.00250933525563609,
-1.54567361576959));
#68490=CARTESIAN_POINT('Ctrl Pts',(0.237074360950808,0.00794202820876042,
-1.54502644709862));
#68491=CARTESIAN_POINT('Ctrl Pts',(0.236910833666278,0.0118569134303206,
-1.5447855775441));
#68492=CARTESIAN_POINT('Ctrl Pts',(0.235447125741487,0.0338274066397509,
-1.54343455705116));
#68493=CARTESIAN_POINT('Ctrl Pts',(0.232180434876699,0.0516894852950028,
-1.54233338054061));
#68494=CARTESIAN_POINT('Ctrl Pts',(0.226014732182807,0.0719644789403343,
-1.54096289516608));
#68495=CARTESIAN_POINT('Ctrl Pts',(0.225057166030109,0.0749053801037273,
-1.54076117758595));
#68496=CARTESIAN_POINT('Ctrl Pts',(0.223552564501143,0.079236733408524,
-1.54045931095087));
#68497=CARTESIAN_POINT('Ctrl Pts',(0.223049431365746,0.0806421726657788,
-1.54036060635765));
#68498=CARTESIAN_POINT('Ctrl Pts',(0.222127830795571,0.0831419258734293,
-1.54018365116373));
#68499=CARTESIAN_POINT('Ctrl Pts',(0.221714455426029,0.0842380746603786,
-1.54010557230142));
#68500=CARTESIAN_POINT('Ctrl Pts',(0.220822055629857,0.0865523752381976,
-1.53993967557087));
#68501=CARTESIAN_POINT('Ctrl Pts',(0.220341035212367,0.087769710004237,
-1.53985179282678));
#68502=CARTESIAN_POINT('Ctrl Pts',(0.21902550993899,0.091019974198752,-1.53961544748848));
#68503=CARTESIAN_POINT('Ctrl Pts',(0.218172803279667,0.0930453494221007,
-1.53946637526698));
#68504=CARTESIAN_POINT('Ctrl Pts',(0.213553675006278,0.103604108676579,
-1.53867952657932));
#68505=CARTESIAN_POINT('Ctrl Pts',(0.209314887335971,0.111920602462604,
-1.53802576850633));
#68506=CARTESIAN_POINT('Ctrl Pts',(0.199197372849681,0.129175816892105,
-1.53659531412792));
#68507=CARTESIAN_POINT('Ctrl Pts',(0.193181233905292,0.138010747883932,
-1.53581596621799));
#68508=CARTESIAN_POINT('Ctrl Pts',(0.179151971643283,0.155890249861244,
-1.5341562542592));
#68509=CARTESIAN_POINT('Ctrl Pts',(0.171000524460262,0.164791011818302,
-1.53327806041202));
#68510=CARTESIAN_POINT('Ctrl Pts',(0.160691007038307,0.174455435602565,
-1.53229227614546));
#68511=CARTESIAN_POINT('Ctrl Pts',(0.159156288233608,0.175856689966613,
-1.53214849088208));
#68512=CARTESIAN_POINT('Ctrl Pts',(0.156979957509692,0.177791927058622,
-1.53194893903163));
#68513=CARTESIAN_POINT('Ctrl Pts',(0.156353696833787,0.178342922276559,
-1.53189200969239));
#68514=CARTESIAN_POINT('Ctrl Pts',(0.155217574750184,0.17933191815341,-1.53178964018432));
#68515=CARTESIAN_POINT('Ctrl Pts',(0.154708734540378,0.179771076308688,
-1.5317441165398));
#68516=CARTESIAN_POINT('Ctrl Pts',(0.153663151867028,0.180665746427945,
-1.53165124797291));
#68517=CARTESIAN_POINT('Ctrl Pts',(0.153126237508268,0.181121041277761,
-1.5316039185876));
#68518=CARTESIAN_POINT('Ctrl Pts',(0.15173616977246,0.1822891971724,-1.53148228226324));
#68519=CARTESIAN_POINT('Ctrl Pts',(0.150880005006412,0.182998472216423,
-1.53140823068345));
#68520=CARTESIAN_POINT('Ctrl Pts',(0.147199355803761,0.186004251457002,
-1.53109340631247));
#68521=CARTESIAN_POINT('Ctrl Pts',(0.144327022069157,0.188241722628779,
-1.53085650512341));
#68522=CARTESIAN_POINT('Ctrl Pts',(0.136201568036226,0.194275852817154,
-1.5302067416342));
#68523=CARTESIAN_POINT('Ctrl Pts',(0.130842459506234,0.197924826773105,
-1.52980100209372));
#68524=CARTESIAN_POINT('Ctrl Pts',(0.121647353085139,0.203648776817385,
-1.52913022882568));
#68525=CARTESIAN_POINT('Ctrl Pts',(0.117891831130865,0.205845622711681,
-1.52886294117754));
#68526=CARTESIAN_POINT('Ctrl Pts',(0.098557526277699,0.216452717935185,
-1.52751035921817));
#68527=CARTESIAN_POINT('Ctrl Pts',(0.082134568345313,0.223202134276999,
-1.52643183025522));
#68528=CARTESIAN_POINT('Ctrl Pts',(0.0621134700864995,0.228918407631067,
-1.5250856418275));
#68529=CARTESIAN_POINT('Ctrl Pts',(0.0590960108539749,0.229715869147917,
-1.52488212178102));
#68530=CARTESIAN_POINT('Ctrl Pts',(0.0546081342243292,0.230807661679454,
-1.52457807534288));
#68531=CARTESIAN_POINT('Ctrl Pts',(0.0531491686735988,0.231147984437338,
-1.52447902459574));
#68532=CARTESIAN_POINT('Ctrl Pts',(0.0505431752407854,0.231729889920066,
-1.52430168525066));
#68533=CARTESIAN_POINT('Ctrl Pts',(0.0493973861112057,0.231976836357658,
-1.52422357127617));
#68534=CARTESIAN_POINT('Ctrl Pts',(0.0469712672034625,0.232480936817258,
-1.52405784833121));
#68535=CARTESIAN_POINT('Ctrl Pts',(0.0456905538446019,0.232736028790258,
-1.52397017633583));
#68536=CARTESIAN_POINT('Ctrl Pts',(0.0422629836936132,0.233389349151447,
-1.52373500223649));
#68537=CARTESIAN_POINT('Ctrl Pts',(0.0401126681567993,0.233768520945373,
-1.52358690100049));
#68538=CARTESIAN_POINT('Ctrl Pts',(0.0289672507140675,0.235575524796537,
-1.52281614370083));
#68539=CARTESIAN_POINT('Ctrl Pts',(0.0199016736731542,0.236513879936278,
-1.5221782883199));
#68540=CARTESIAN_POINT('Ctrl Pts',(-1.4024014571486E-5,0.237422171039584,
-1.52075395183144));
#68541=CARTESIAN_POINT('Ctrl Pts',(-0.0108539915600171,0.23717387463299,
-1.51996361814138));
#68542=CARTESIAN_POINT('Ctrl Pts',(-0.028443735834832,0.235562387824582,
-1.5186736308643));
#68543=CARTESIAN_POINT('Ctrl Pts',(-0.0352170706831922,0.234645232886711,
-1.51817526932316));
#68544=CARTESIAN_POINT('Ctrl Pts',(-0.0419392871413391,0.233437522303241,
-1.51768363453027));
#68545=CARTESIAN_POINT('Origin',(0.,0.,-2.1456589891905));
#68546=CARTESIAN_POINT('',(-0.0419392741322232,0.233437524640453,-1.39788629978594));
#68547=CARTESIAN_POINT('',(-0.0419392748056672,0.233437524519463,-1.41774927189049));
#68548=CARTESIAN_POINT('',(-0.0419392741328076,0.233437524640348,-2.1456589891905));
#68549=CARTESIAN_POINT('',(-0.237174975146335,-0.000108578706768982,-1.47575156156963));
#68550=CARTESIAN_POINT('Ctrl Pts',(-0.0419392741322232,0.233437524640453,
-1.39788629978594));
#68551=CARTESIAN_POINT('Ctrl Pts',(-0.0417180158744456,0.233477275793321,
-1.39790131808953));
#68552=CARTESIAN_POINT('Ctrl Pts',(-0.0414967013879086,0.233516712322986,
-1.39791634640987));
#68553=CARTESIAN_POINT('Ctrl Pts',(-0.03997497007651,0.233785641439333,
-1.39801972238812));
#68554=CARTESIAN_POINT('Ctrl Pts',(-0.0386727356578481,0.234004580660391,
-1.39810840368024));
#68555=CARTESIAN_POINT('Ctrl Pts',(-0.0351472170219117,0.234567079239536,
-1.39834910766252));
#68556=CARTESIAN_POINT('Ctrl Pts',(-0.0329208096375801,0.23488989167629,
-1.39850177937129));
#68557=CARTESIAN_POINT('Ctrl Pts',(-0.0205616969838143,0.236502708322871,
-1.39935321128919));
#68558=CARTESIAN_POINT('Ctrl Pts',(-0.0103598125379389,0.237168582931925,
-1.40007131630334));
#68559=CARTESIAN_POINT('Ctrl Pts',(0.00983488366610878,0.237181181891399,
-1.40152083381518));
#68560=CARTESIAN_POINT('Ctrl Pts',(0.0198076613864323,0.236557124939314,
-1.4022501113566));
#68561=CARTESIAN_POINT('Ctrl Pts',(0.0341751828074724,0.234743020647505,
-1.4033075762913));
#68562=CARTESIAN_POINT('Ctrl Pts',(0.0386226802781399,0.234052385055344,
-1.40363577598582));
#68563=CARTESIAN_POINT('Ctrl Pts',(0.0511782513117806,0.231735024255397,
-1.40456114737663));
#68564=CARTESIAN_POINT('Ctrl Pts',(0.0592255204948725,0.229810145643756,
-1.40515298587548));
#68565=CARTESIAN_POINT('Ctrl Pts',(0.0684271973005747,0.227093492737877,
-1.40581676211146));
#68566=CARTESIAN_POINT('Ctrl Pts',(0.0696946706410852,0.226707716803832,
-1.4059078976691));
#68567=CARTESIAN_POINT('Ctrl Pts',(0.0717499760047658,0.226063285224635,
-1.40605512569324));
#68568=CARTESIAN_POINT('Ctrl Pts',(0.0725397807810432,0.225811089719167,
-1.40611156779772));
#68569=CARTESIAN_POINT('Ctrl Pts',(0.0739516835641688,0.225352077547534,
-1.40621220635755));
#68570=CARTESIAN_POINT('Ctrl Pts',(0.0745742607516494,0.22514681881604,
-1.40625649022976));
#68571=CARTESIAN_POINT('Ctrl Pts',(0.0759436644003392,0.224689033840108,
-1.40635369094314));
#68572=CARTESIAN_POINT('Ctrl Pts',(0.0766900875522137,0.224435363985013,
-1.40640654024647));
#68573=CARTESIAN_POINT('Ctrl Pts',(0.0788530244302914,0.223688245316555,
-1.40655933775896));
#68574=CARTESIAN_POINT('Ctrl Pts',(0.080266170777264,0.223185063725022,
-1.4066587354356));
#68575=CARTESIAN_POINT('Ctrl Pts',(0.0936881257930744,0.218261909338375,
-1.40759953923139));
#68576=CARTESIAN_POINT('Ctrl Pts',(0.105327294131923,0.212889603563721,
-1.40839094762103));
#68577=CARTESIAN_POINT('Ctrl Pts',(0.13287309346103,0.197360026008351,-1.41033273705339));
#68578=CARTESIAN_POINT('Ctrl Pts',(0.148108278852666,0.18619906552795,-1.41147468771679));
#68579=CARTESIAN_POINT('Ctrl Pts',(0.164076912938587,0.171288981820243,
-1.41288836970618));
#68580=CARTESIAN_POINT('Ctrl Pts',(0.166250179703749,0.169180451128731,
-1.41308594002728));
#68581=CARTESIAN_POINT('Ctrl Pts',(0.169425175322059,0.165979766785024,
-1.4133828055702));
#68582=CARTESIAN_POINT('Ctrl Pts',(0.170458054400523,0.164918842275546,
-1.41348072702198));
#68583=CARTESIAN_POINT('Ctrl Pts',(0.172289593164401,0.163001984611306,
-1.41365684200265));
#68584=CARTESIAN_POINT('Ctrl Pts',(0.173091984094836,0.162149671161329,
-1.4137348704784));
#68585=CARTESIAN_POINT('Ctrl Pts',(0.17478358582726,0.160325958570626,-1.41390126213349));
#68586=CARTESIAN_POINT('Ctrl Pts',(0.175671078058892,0.15935302657418,-1.41398969474534));
#68587=CARTESIAN_POINT('Ctrl Pts',(0.178041482653542,0.156710552792748,
-1.41422901305029));
#68588=CARTESIAN_POINT('Ctrl Pts',(0.179508963501372,0.155027411542843,
-1.41438053502395));
#68589=CARTESIAN_POINT('Ctrl Pts',(0.187361030769182,0.145760421728771,
-1.41521012223092));
#68590=CARTESIAN_POINT('Ctrl Pts',(0.193288262647181,0.137803687082492,
-1.41590635290925));
#68591=CARTESIAN_POINT('Ctrl Pts',(0.204268242513911,0.120956492033935,
-1.41734800311278));
#68592=CARTESIAN_POINT('Ctrl Pts',(0.20927950829322,0.112062712993019,-1.41809280223622));
#68593=CARTESIAN_POINT('Ctrl Pts',(0.214642323710848,0.100922483452259,
-1.41899567148415));
#68594=CARTESIAN_POINT('Ctrl Pts',(0.215555299066054,0.0989575057310869,
-1.41915381260305));
#68595=CARTESIAN_POINT('Ctrl Pts',(0.220801063905372,0.0872499738251653,
-1.42008870073981));
#68596=CARTESIAN_POINT('Ctrl Pts',(0.224500325589006,0.0772355193366812,
-1.42085914020115));
#68597=CARTESIAN_POINT('Ctrl Pts',(0.227896164392543,0.0657050634842037,
-1.42169114483246));
#68598=CARTESIAN_POINT('Ctrl Pts',(0.228267880313989,0.0644018023238318,
-1.42178440382792));
#68599=CARTESIAN_POINT('Ctrl Pts',(0.228851382788145,0.0622874600940939,
-1.42193436350777));
#68600=CARTESIAN_POINT('Ctrl Pts',(0.229070070039358,0.061478338913267,
-1.42199143477438));
#68601=CARTESIAN_POINT('Ctrl Pts',(0.22945228028266,0.06003384122748,-1.42209273955511));
#68602=CARTESIAN_POINT('Ctrl Pts',(0.229617460816204,0.0593989288000395,
-1.42213706563693));
#68603=CARTESIAN_POINT('Ctrl Pts',(0.229973518346591,0.0580066502121284,
-1.42223382471026));
#68604=CARTESIAN_POINT('Ctrl Pts',(0.230163290180798,0.05724902188514,-1.42228619447312));
#68605=CARTESIAN_POINT('Ctrl Pts',(0.230698261311157,0.0550675872870964,
-1.42243620611052));
#68606=CARTESIAN_POINT('Ctrl Pts',(0.231034022972514,0.0536414712569274,
-1.42253332783677));
#68607=CARTESIAN_POINT('Ctrl Pts',(0.233624760573055,0.0421617196478598,
-1.42330819945264));
#68608=CARTESIAN_POINT('Ctrl Pts',(0.2352359390451,0.0319726239218326,-1.42395362207822));
#68609=CARTESIAN_POINT('Ctrl Pts',(0.237663091612336,0.00556783595630032,
-1.42559129702647));
#68610=CARTESIAN_POINT('Ctrl Pts',(0.237488122953125,-0.010683077692122,
-1.42656856752845));
#68611=CARTESIAN_POINT('Ctrl Pts',(0.234888007935024,-0.0335556617833019,
-1.4280191073462));
#68612=CARTESIAN_POINT('Ctrl Pts',(0.233827783020413,-0.040285396487299,
-1.42845480617632));
#68613=CARTESIAN_POINT('Ctrl Pts',(0.23206974185919,-0.0489887789261965,
-1.42903481620551));
#68614=CARTESIAN_POINT('Ctrl Pts',(0.231633354083273,-0.051012296321916,
-1.42917083735685));
#68615=CARTESIAN_POINT('Ctrl Pts',(0.230884016810966,-0.0542788509147047,
-1.42939243560929));
#68616=CARTESIAN_POINT('Ctrl Pts',(0.230587372652463,-0.0555255467241055,
-1.42947748895719));
#68617=CARTESIAN_POINT('Ctrl Pts',(0.229998495429776,-0.0579142662485055,
-1.42964140513735));
#68618=CARTESIAN_POINT('Ctrl Pts',(0.229707822124248,-0.0590566380975076,
-1.42972021551665));
#68619=CARTESIAN_POINT('Ctrl Pts',(0.229015822727977,-0.0616938331768712,
-1.42990314707741));
#68620=CARTESIAN_POINT('Ctrl Pts',(0.228608359557043,-0.0631869753556153,
-1.43000746413829));
#68621=CARTESIAN_POINT('Ctrl Pts',(0.227262413432004,-0.0679356693006557,
-1.43034166487229));
#68622=CARTESIAN_POINT('Ctrl Pts',(0.226268809838192,-0.0711750191416556,
-1.43057332177028));
#68623=CARTESIAN_POINT('Ctrl Pts',(0.223763820229987,-0.0787583675917747,
-1.43112463823769));
#68624=CARTESIAN_POINT('Ctrl Pts',(0.222194834380575,-0.0830817575420814,
-1.4314460544567));
#68625=CARTESIAN_POINT('Ctrl Pts',(0.211856710958257,-0.109176751618474,
-1.43342971160973));
#68626=CARTESIAN_POINT('Ctrl Pts',(0.200023261566123,-0.129588831847011,
-1.43518731180815));
#68627=CARTESIAN_POINT('Ctrl Pts',(0.183115788880297,-0.150777517222346,
-1.43710599965592));
#68628=CARTESIAN_POINT('Ctrl Pts',(0.180778147620777,-0.153572513004489,
-1.43736088086582));
#68629=CARTESIAN_POINT('Ctrl Pts',(0.177616866838394,-0.157180021258988,
-1.43769105721541));
#68630=CARTESIAN_POINT('Ctrl Pts',(0.176850510712848,-0.158041790249973,
-1.43777002309563));
#68631=CARTESIAN_POINT('Ctrl Pts',(0.175600041117248,-0.159427459641087,
-1.43789709743272));
#68632=CARTESIAN_POINT('Ctrl Pts',(0.175119808028802,-0.159954812988614,
-1.43794548326542));
#68633=CARTESIAN_POINT('Ctrl Pts',(0.174180724207529,-0.160976740729747,
-1.43803928086469));
#68634=CARTESIAN_POINT('Ctrl Pts',(0.173722133680186,-0.161471533170899,
-1.43808470945402));
#68635=CARTESIAN_POINT('Ctrl Pts',(0.172598408722607,-0.16267363830348,
-1.4381951319603));
#68636=CARTESIAN_POINT('Ctrl Pts',(0.171931020374284,-0.163378846879691,
-1.43825995641693));
#68637=CARTESIAN_POINT('Ctrl Pts',(0.169509534141475,-0.165906285757507,
-1.43849253890809));
#68638=CARTESIAN_POINT('Ctrl Pts',(0.167730572779489,-0.167704603526047,
-1.4386585071294));
#68639=CARTESIAN_POINT('Ctrl Pts',(0.163177058129923,-0.17216270525143,
-1.43907227369118));
#68640=CARTESIAN_POINT('Ctrl Pts',(0.16036592203834,-0.174784220662538,
-1.43931774981842));
#68641=CARTESIAN_POINT('Ctrl Pts',(0.146744586031513,-0.186881306487395,
-1.44046812851552));
#68642=CARTESIAN_POINT('Ctrl Pts',(0.135150896485953,-0.195430006833203,
-1.44133605221261));
#68643=CARTESIAN_POINT('Ctrl Pts',(0.111834438521158,-0.209549496725397,
-1.44301440210219));
#68644=CARTESIAN_POINT('Ctrl Pts',(0.100291255550789,-0.21531263792928,
-1.44381864326232));
#68645=CARTESIAN_POINT('Ctrl Pts',(0.086120809048198,-0.220999764494372,
-1.4448123411068));
#68646=CARTESIAN_POINT('Ctrl Pts',(0.0838901169891483,-0.221856118350098,
-1.44496889198576));
#68647=CARTESIAN_POINT('Ctrl Pts',(0.0803656021851481,-0.22314841056952,
-1.44521662615804));
#68648=CARTESIAN_POINT('Ctrl Pts',(0.0790802638549645,-0.223607144096794,
-1.44530704962001));
#68649=CARTESIAN_POINT('Ctrl Pts',(0.0767001855823566,-0.224433499315008,
-1.44547466666692));
#68650=CARTESIAN_POINT('Ctrl Pts',(0.0756065761486757,-0.224804269632509,
-1.44555175318055));
#68651=CARTESIAN_POINT('Ctrl Pts',(0.0731717810759798,-0.22560997087226,
-1.44572355194719));
#68652=CARTESIAN_POINT('Ctrl Pts',(0.0718293457237878,-0.226040955241188,
-1.44581839095064));
#68653=CARTESIAN_POINT('Ctrl Pts',(0.0679315346937054,-0.227254106186454,
-1.44609414010938));
#68654=CARTESIAN_POINT('Ctrl Pts',(0.0653667523079446,-0.228005063230244,
-1.44627605806188));
#68655=CARTESIAN_POINT('Ctrl Pts',(0.0502687969417475,-0.232150002322363,
-1.44735011117685));
#68656=CARTESIAN_POINT('Ctrl Pts',(0.037488629829059,-0.234552932241655,
-1.4482737957892));
#68657=CARTESIAN_POINT('Ctrl Pts',(0.0116579680877888,-0.237244200540142,
-1.45015765546247));
#68658=CARTESIAN_POINT('Ctrl Pts',(-0.00135059597956813,-0.237526618653894,
-1.45111455511102));
#68659=CARTESIAN_POINT('Ctrl Pts',(-0.0207136129501226,-0.236355654367896,
-1.45251056038645));
#68660=CARTESIAN_POINT('Ctrl Pts',(-0.0270927506522178,-0.235709669280235,
-1.4529655266607));
#68661=CARTESIAN_POINT('Ctrl Pts',(-0.0347895741262106,-0.234613573098142,
-1.45350269108032));
#68662=CARTESIAN_POINT('Ctrl Pts',(-0.0361390404583626,-0.234409498795688,
-1.4535964256256));
#68663=CARTESIAN_POINT('Ctrl Pts',(-0.0382448730749671,-0.234072424364735,
-1.45374192339876));
#68664=CARTESIAN_POINT('Ctrl Pts',(-0.0390024565063026,-0.233947384241106,
-1.45379410986171));
#68665=CARTESIAN_POINT('Ctrl Pts',(-0.0404014421049144,-0.233709495303012,
-1.45389017247768));
#68666=CARTESIAN_POINT('Ctrl Pts',(-0.0410429860422308,-0.233597684131298,
-1.45393410314572));
#68667=CARTESIAN_POINT('Ctrl Pts',(-0.0425235031536307,-0.233333365346629,
-1.45403521088997));
#68668=CARTESIAN_POINT('Ctrl Pts',(-0.0433621221315177,-0.233178974449585,
-1.45409228119432));
#68669=CARTESIAN_POINT('Ctrl Pts',(-0.0459926076329107,-0.23268001649431,
-1.45427071397988));
#68670=CARTESIAN_POINT('Ctrl Pts',(-0.0477813926821057,-0.232319282557509,
-1.45439120696135));
#68671=CARTESIAN_POINT('Ctrl Pts',(-0.0519974765152204,-0.231418291479187,
-1.45467358720743));
#68672=CARTESIAN_POINT('Ctrl Pts',(-0.054420833424717,-0.23086042785102,
-1.45483462335879));
#68673=CARTESIAN_POINT('Ctrl Pts',(-0.0632751560660881,-0.228674958606493,
-1.4554198241311));
#68674=CARTESIAN_POINT('Ctrl Pts',(-0.0696462064266515,-0.226815786063484,
-1.4558347429976));
#68675=CARTESIAN_POINT('Ctrl Pts',(-0.0883866319381735,-0.220482730437716,
-1.45705887381467));
#68676=CARTESIAN_POINT('Ctrl Pts',(-0.100470320113976,-0.215245331034556,
-1.45785421754155));
#68677=CARTESIAN_POINT('Ctrl Pts',(-0.120884682909554,-0.204301682727748,
-1.45929249561858));
#68678=CARTESIAN_POINT('Ctrl Pts',(-0.129401950223741,-0.199016036320406,
-1.45992483000394));
#68679=CARTESIAN_POINT('Ctrl Pts',(-0.139421971966469,-0.191882057641465,
-1.46072617197113));
#68680=CARTESIAN_POINT('Ctrl Pts',(-0.141265559083674,-0.190528873219768,
-1.46087612721574));
#68681=CARTESIAN_POINT('Ctrl Pts',(-0.144159223654674,-0.188339849483859,
-1.46111569257743));
#68682=CARTESIAN_POINT('Ctrl Pts',(-0.145222301037575,-0.187521368980477,
-1.46120462463978));
#68683=CARTESIAN_POINT('Ctrl Pts',(-0.147156294487133,-0.186006047127048,
-1.4613681416619));
#68684=CARTESIAN_POINT('Ctrl Pts',(-0.148029353980594,-0.185311993302888,
-1.46144261437169));
#68685=CARTESIAN_POINT('Ctrl Pts',(-0.148929261989617,-0.184586178291161,
-1.46152007057849));
#68686=CARTESIAN_POINT('Ctrl Pts',(-0.148961044335912,-0.184560530892332,
-1.46152280702652));
#68687=CARTESIAN_POINT('Ctrl Pts',(-0.149021894573208,-0.184511400621211,
-1.46152804793698));
#68688=CARTESIAN_POINT('Ctrl Pts',(-0.149050963544898,-0.184487919083402,
-1.46153055234557));
#68689=CARTESIAN_POINT('Ctrl Pts',(-0.149106764748591,-0.184442821798687,
-1.46153536129486));
#68690=CARTESIAN_POINT('Ctrl Pts',(-0.149133497834717,-0.184421207106,-1.46153766579299));
#68691=CARTESIAN_POINT('Ctrl Pts',(-0.149184937196628,-0.184379597973357,
-1.46154210130256));
#68692=CARTESIAN_POINT('Ctrl Pts',(-0.149209644156208,-0.184359604376758,
-1.46154423227993));
#68693=CARTESIAN_POINT('Ctrl Pts',(-0.14925728815938,-0.184321033600422,
-1.46154834263563));
#68694=CARTESIAN_POINT('Ctrl Pts',(-0.149280225756973,-0.184302457102899,
-1.4615503219864));
#68695=CARTESIAN_POINT('Ctrl Pts',(-0.149324545929468,-0.184266549773775,
-1.46155414741404));
#68696=CARTESIAN_POINT('Ctrl Pts',(-0.149345928957762,-0.18424921949988,
-1.46155599346837));
#68697=CARTESIAN_POINT('Ctrl Pts',(-0.149387321254059,-0.18421566040183,
-1.46155956777281));
#68698=CARTESIAN_POINT('Ctrl Pts',(-0.149407330896319,-0.184199432038166,
-1.46156129600429));
#68699=CARTESIAN_POINT('Ctrl Pts',(-0.149446130482059,-0.184167954038028,
-1.46156464782109));
#68700=CARTESIAN_POINT('Ctrl Pts',(-0.149464920737452,-0.184152704784807,
-1.46156627139091));
#68701=CARTESIAN_POINT('Ctrl Pts',(-0.149501413410188,-0.184123079849844,
-1.46156942515416));
#68702=CARTESIAN_POINT('Ctrl Pts',(-0.149519116089556,-0.184108704489585,
-1.4615709553346));
#68703=CARTESIAN_POINT('Ctrl Pts',(-0.150638741112207,-0.183199251358231,
-1.46166775112811));
#68704=CARTESIAN_POINT('Ctrl Pts',(-0.151732585497013,-0.182294317979909,
-1.46176341422604));
#68705=CARTESIAN_POINT('Ctrl Pts',(-0.154073979078429,-0.180321618032845,
-1.46197059519738));
#68706=CARTESIAN_POINT('Ctrl Pts',(-0.155318688741653,-0.179250611296165,
-1.46208224283019));
#68707=CARTESIAN_POINT('Ctrl Pts',(-0.158604971914649,-0.176363009745009,
-1.46238111300163));
#68708=CARTESIAN_POINT('Ctrl Pts',(-0.160626388404096,-0.174523954223284,
-1.46256925180537));
#68709=CARTESIAN_POINT('Ctrl Pts',(-0.166798035983302,-0.168711020511071,
-1.46315734558808));
#68710=CARTESIAN_POINT('Ctrl Pts',(-0.170835719935327,-0.164621204565371,
-1.46356196397502));
#68711=CARTESIAN_POINT('Ctrl Pts',(-0.190433080646042,-0.143272721018108,
-1.46562831269273));
#68712=CARTESIAN_POINT('Ctrl Pts',(-0.203543292903344,-0.123942804942166,
-1.46737177133099));
#68713=CARTESIAN_POINT('Ctrl Pts',(-0.214616452691466,-0.10097957856647,
-1.46915379271452));
#68714=CARTESIAN_POINT('Ctrl Pts',(-0.215569780863005,-0.0989280929213326,
-1.46931054233741));
#68715=CARTESIAN_POINT('Ctrl Pts',(-0.216846180175783,-0.0960752821580489,
-1.46952484624184));
#68716=CARTESIAN_POINT('Ctrl Pts',(-0.217194407805216,-0.0952854394698288,
-1.46958379475124));
#68717=CARTESIAN_POINT('Ctrl Pts',(-0.217784905235448,-0.093926027963194,
-1.4696845713024));
#68718=CARTESIAN_POINT('Ctrl Pts',(-0.218029268836749,-0.0933573865871296,
-1.46972652277562));
#68719=CARTESIAN_POINT('Ctrl Pts',(-0.218537693353963,-0.0921613829037323,
-1.46981432171694));
#68720=CARTESIAN_POINT('Ctrl Pts',(-0.218801284065018,-0.0915338299492834,
-1.46986013882558));
#68721=CARTESIAN_POINT('Ctrl Pts',(-0.219446157546607,-0.0899798212374725,
-1.46997299494483));
#68722=CARTESIAN_POINT('Ctrl Pts',(-0.219824284505007,-0.0890520540117648,
-1.47003984641765));
#68723=CARTESIAN_POINT('Ctrl Pts',(-0.221215782656704,-0.085575017414246,
-1.47028853076473));
#68724=CARTESIAN_POINT('Ctrl Pts',(-0.222190825871268,-0.0830105089607385,
-1.47046823267838));
#68725=CARTESIAN_POINT('Ctrl Pts',(-0.224579214202513,-0.0763848317532693,
-1.47092445191497));
#68726=CARTESIAN_POINT('Ctrl Pts',(-0.225927062428807,-0.0723009883580598,
-1.47119799395673));
#68727=CARTESIAN_POINT('Ctrl Pts',(-0.233791840176752,-0.0460979656414309,
-1.47291810075487));
#68728=CARTESIAN_POINT('Ctrl Pts',(-0.23716441931536,-0.0231663128024612,
-1.47427942647711));
#68729=CARTESIAN_POINT('Ctrl Pts',(-0.237174975146335,-0.000108578706768982,
-1.47575156156963));
#68730=CARTESIAN_POINT('Ctrl Pts',(-0.237174975268681,-0.000108311127839238,
-1.47575157865337));
#68731=CARTESIAN_POINT('Ctrl Pts',(-0.237176942139156,0.00419865589782415,
-1.47602655971673));
#68732=CARTESIAN_POINT('Ctrl Pts',(-0.237061591014441,0.00850470375074625,
-1.47630458183463));
#68733=CARTESIAN_POINT('Ctrl Pts',(-0.23674953108947,0.0142762308575994,
-1.47668253285185));
#68734=CARTESIAN_POINT('Ctrl Pts',(-0.236656282952957,0.0157465811043548,
-1.47677928072747));
#68735=CARTESIAN_POINT('Ctrl Pts',(-0.236466528519261,0.0183538326312364,
-1.47695170294741));
#68736=CARTESIAN_POINT('Ctrl Pts',(-0.236375505087181,0.0194910954087698,
-1.47702720537737));
#68737=CARTESIAN_POINT('Ctrl Pts',(-0.236177920258972,0.0217543018139207,
-1.47717806497058));
#68738=CARTESIAN_POINT('Ctrl Pts',(-0.236071503487122,0.0228802279399359,
-1.47725341569058));
#68739=CARTESIAN_POINT('Ctrl Pts',(-0.235826903284639,0.0252844911395987,
-1.47741497731558));
#68740=CARTESIAN_POINT('Ctrl Pts',(-0.235686369531058,0.0265625471159161,
-1.47750125985415));
#68741=CARTESIAN_POINT('Ctrl Pts',(-0.23529017709805,0.0299145391006344,
-1.47772863696547));
#68742=CARTESIAN_POINT('Ctrl Pts',(-0.235017494159398,0.0319863101926931,
-1.47787026237332));
#68743=CARTESIAN_POINT('Ctrl Pts',(-0.233711756277124,0.040986079465285,
-1.47849040316061));
#68744=CARTESIAN_POINT('Ctrl Pts',(-0.232399548797854,0.0478693631792046,
-1.4789775804693));
#68745=CARTESIAN_POINT('Ctrl Pts',(-0.227985198379171,0.0664994283455132,
-1.48033214961534));
#68746=CARTESIAN_POINT('Ctrl Pts',(-0.224282571822886,0.0780813465774943,
-1.48121515174549));
#68747=CARTESIAN_POINT('Ctrl Pts',(-0.215995457900528,0.0984643019394832,
-1.48282214009222));
#68748=CARTESIAN_POINT('Ctrl Pts',(-0.211714293275484,0.107360772627073,
-1.48354300050456));
#68749=CARTESIAN_POINT('Ctrl Pts',(-0.205345684533884,0.118722889252388,
-1.48447141503645));
#68750=CARTESIAN_POINT('Ctrl Pts',(-0.203744912691526,0.121449525291398,
-1.48469479268469));
#68751=CARTESIAN_POINT('Ctrl Pts',(-0.200944168466027,0.126008786036631,
-1.48506832513154));
#68752=CARTESIAN_POINT('Ctrl Pts',(-0.199772488970182,0.127858228158493,
-1.48521985099335));
#68753=CARTESIAN_POINT('Ctrl Pts',(-0.198073755895315,0.130459224207009,
-1.48543267126681));
#68754=CARTESIAN_POINT('Ctrl Pts',(-0.197567732101147,0.131224286083186,
-1.4854952354785));
#68755=CARTESIAN_POINT('Ctrl Pts',(-0.196687051479929,0.132539152683675,
-1.48560267373702));
#68756=CARTESIAN_POINT('Ctrl Pts',(-0.196314500126047,0.133090346382632,
-1.4856476847727));
#68757=CARTESIAN_POINT('Ctrl Pts',(-0.19552604670506,0.134246357187083,
-1.48574201974106));
#68758=CARTESIAN_POINT('Ctrl Pts',(-0.195109651966513,0.134850817960496,
-1.48579131001653));
#68759=CARTESIAN_POINT('Ctrl Pts',(-0.193978175510031,0.136477117105381,
-1.4859238562774));
#68760=CARTESIAN_POINT('Ctrl Pts',(-0.193257816880505,0.137495281558845,
-1.48600676442978));
#68761=CARTESIAN_POINT('Ctrl Pts',(-0.189863940379462,0.142212859993805,
-1.48639080806166));
#68762=CARTESIAN_POINT('Ctrl Pts',(-0.187091828439924,0.14584055565954,
-1.48668583075819));
#68763=CARTESIAN_POINT('Ctrl Pts',(-0.181448784345523,0.152799308373986,
-1.48725611972243));
#68764=CARTESIAN_POINT('Ctrl Pts',(-0.178586588391015,0.15613495478841,
-1.48753159899791));
#68765=CARTESIAN_POINT('Ctrl Pts',(-0.16427753170964,0.17190229910262,-1.48885475749445));
#68766=CARTESIAN_POINT('Ctrl Pts',(-0.151617324412263,0.183165807133074,
-1.48986924296888));
#68767=CARTESIAN_POINT('Ctrl Pts',(-0.133652607439386,0.195999468553181,
-1.49125403085675));
#68768=CARTESIAN_POINT('Ctrl Pts',(-0.129340536682154,0.198871393849842,
-1.49158245329919));
#68769=CARTESIAN_POINT('Ctrl Pts',(-0.122774301136254,0.202940710414367,
-1.4920795099872));
#68770=CARTESIAN_POINT('Ctrl Pts',(-0.120589106158515,0.204246732317007,
-1.49224443472819));
#68771=CARTESIAN_POINT('Ctrl Pts',(-0.116551409552228,0.206572551991343,
-1.4925485933385));
#68772=CARTESIAN_POINT('Ctrl Pts',(-0.114705465280959,0.207603241940051,
-1.4926874302666));
#68773=CARTESIAN_POINT('Ctrl Pts',(-0.111723549725092,0.209216294145764,
-1.49291148799726));
#68774=CARTESIAN_POINT('Ctrl Pts',(-0.110596198904925,0.209814417948167,
-1.49299614643234));
#68775=CARTESIAN_POINT('Ctrl Pts',(-0.108479606801616,0.210915592323176,
-1.49315502775177));
#68776=CARTESIAN_POINT('Ctrl Pts',(-0.107491551325656,0.211420856346486,
-1.49322916992968));
#68777=CARTESIAN_POINT('Ctrl Pts',(-0.105192700118224,0.212576144309204,
-1.49340163206101));
#68778=CARTESIAN_POINT('Ctrl Pts',(-0.103879374560099,0.213221004269078,
-1.49350012919098));
#68779=CARTESIAN_POINT('Ctrl Pts',(-0.0999973484469963,0.215082750961096,
-1.49379123460219));
#68780=CARTESIAN_POINT('Ctrl Pts',(-0.097412719933139,0.21626562424125,
-1.49398500316672));
#68781=CARTESIAN_POINT('Ctrl Pts',(-0.0778616014625455,0.22479174676208,
-1.4954509833057));
#68782=CARTESIAN_POINT('Ctrl Pts',(-0.0601175388771464,0.230171626328724,
-1.49679027381849));
#68783=CARTESIAN_POINT('Ctrl Pts',(-0.0419392735583878,0.233437524743548,
-1.49813919362704));
#68784=CARTESIAN_POINT('',(-0.237174890926,0.00020565781626766,-1.49572693511662));
#68785=CARTESIAN_POINT('Ctrl Pts',(-0.0419392871413391,0.233437522303241,
-1.51768363453027));
#68786=CARTESIAN_POINT('Ctrl Pts',(-0.0471714318927572,0.232497517376314,
-1.51730097734907));
#68787=CARTESIAN_POINT('Ctrl Pts',(-0.0523726113577256,0.231381492634979,
-1.51692242868031));
#68788=CARTESIAN_POINT('Ctrl Pts',(-0.0595435759879914,0.229588401993189,
-1.51640681856276));
#68789=CARTESIAN_POINT('Ctrl Pts',(-0.0615466280965262,0.229059566642998,
-1.51626349131255));
#68790=CARTESIAN_POINT('Ctrl Pts',(-0.0643451390067523,0.228281356278343,
-1.51606446676699));
#68791=CARTESIAN_POINT('Ctrl Pts',(-0.0651465346722758,0.228053948904293,
-1.51600761450086));
#68792=CARTESIAN_POINT('Ctrl Pts',(-0.0665920699758293,0.227635516121258,
-1.51590534239749));
#68793=CARTESIAN_POINT('Ctrl Pts',(-0.0672366264977959,0.22744596738836,
-1.51585983957156));
#68794=CARTESIAN_POINT('Ctrl Pts',(-0.0685553060007903,0.227052079500925,
-1.51576696314701));
#68795=CARTESIAN_POINT('Ctrl Pts',(-0.069229337734572,0.226847472140091,
-1.5157196054318));
#68796=CARTESIAN_POINT('Ctrl Pts',(-0.07096672319545,0.226311610905123,
-1.51559780983191));
#68797=CARTESIAN_POINT('Ctrl Pts',(-0.0720286881448549,0.225975859855935,
-1.51552362858249));
#68798=CARTESIAN_POINT('Ctrl Pts',(-0.0765688759044532,0.224505175025978,
-1.51520746481205));
#68799=CARTESIAN_POINT('Ctrl Pts',(-0.0800231582017908,0.223297255022286,
-1.51496939487481));
#68800=CARTESIAN_POINT('Ctrl Pts',(-0.0895609428699645,0.219712223293451,
-1.5143153546838));
#68801=CARTESIAN_POINT('Ctrl Pts',(-0.0955765161121631,0.217162992879243,
-1.51390662097318));
#68802=CARTESIAN_POINT('Ctrl Pts',(-0.115163937034608,0.207890533857276,
-1.51256485681436));
#68803=CARTESIAN_POINT('Ctrl Pts',(-0.12819633713789,0.200117243049169,
-1.51165196407475));
#68804=CARTESIAN_POINT('Ctrl Pts',(-0.14714250026197,0.186201699203614,
-1.51018228661346));
#68805=CARTESIAN_POINT('Ctrl Pts',(-0.153618568216865,0.180895827529956,
-1.5096504936495));
#68806=CARTESIAN_POINT('Ctrl Pts',(-0.161433200390491,0.173770496131775,
-1.50896075478208));
#68807=CARTESIAN_POINT('Ctrl Pts',(-0.163045133068398,0.172258954934857,
-1.50881572440554));
#68808=CARTESIAN_POINT('Ctrl Pts',(-0.165579775709671,0.169814718831981,
-1.50858307790472));
#68809=CARTESIAN_POINT('Ctrl Pts',(-0.166516299625678,0.168896485155012,
-1.50849608771351));
#68810=CARTESIAN_POINT('Ctrl Pts',(-0.168274474096228,0.167143810159057,
-1.50833078211358));
#68811=CARTESIAN_POINT('Ctrl Pts',(-0.169097657189908,0.166310956208243,
-1.50825253819057));
#68812=CARTESIAN_POINT('Ctrl Pts',(-0.169935727207506,0.165450385790348,
-1.50817199347841));
#68813=CARTESIAN_POINT('Ctrl Pts',(-0.169956823886617,0.165428714418298,
-1.50816996535157));
#68814=CARTESIAN_POINT('Ctrl Pts',(-0.169997390835274,0.165387026437855,
-1.50816606433595));
#68815=CARTESIAN_POINT('Ctrl Pts',(-0.170016861717709,0.165367010423533,
-1.50816419147391));
#68816=CARTESIAN_POINT('Ctrl Pts',(-0.170054362569926,0.165328446025054,
-1.50816058339409));
#68817=CARTESIAN_POINT('Ctrl Pts',(-0.170072393042106,0.16530989812789,
-1.50815884819826));
#68818=CARTESIAN_POINT('Ctrl Pts',(-0.170107171171144,0.165274110249768,
-1.50815550044037));
#68819=CARTESIAN_POINT('Ctrl Pts',(-0.170123919243162,0.165256870671227,
-1.50815388789646));
#68820=CARTESIAN_POINT('Ctrl Pts',(-0.170156268160965,0.165223562278893,
-1.50815077255669));
#68821=CARTESIAN_POINT('Ctrl Pts',(-0.170171869352431,0.165207493800046,
-1.50814926977595));
#68822=CARTESIAN_POINT('Ctrl Pts',(-0.171178221271394,0.164170705799564,
-1.50805231260119));
#68823=CARTESIAN_POINT('Ctrl Pts',(-0.172159752148018,0.163141115807951,
-1.50795645913309));
#68824=CARTESIAN_POINT('Ctrl Pts',(-0.175241965133097,0.159849194895349,
-1.50765129272431));
#68825=CARTESIAN_POINT('Ctrl Pts',(-0.177307693064479,0.157554726575058,
-1.50744051267301));
#68826=CARTESIAN_POINT('Ctrl Pts',(-0.182033563850823,0.152094882062049,
-1.50694313634357));
#68827=CARTESIAN_POINT('Ctrl Pts',(-0.184656819752731,0.148899049221967,
-1.50665515382933));
#68828=CARTESIAN_POINT('Ctrl Pts',(-0.193902552873168,0.137014965635709,
-1.50559538619098));
#68829=CARTESIAN_POINT('Ctrl Pts',(-0.200005691996505,0.127941302566981,
-1.50480634350546));
#68830=CARTESIAN_POINT('Ctrl Pts',(-0.213271536587294,0.104936496587429,
-1.50287015943048));
#68831=CARTESIAN_POINT('Ctrl Pts',(-0.219723944567586,0.0906525363456694,
-1.50171871634479));
#68832=CARTESIAN_POINT('Ctrl Pts',(-0.225361513210689,0.0739469146941872,
-1.50049060972911));
#68833=CARTESIAN_POINT('Ctrl Pts',(-0.225975355009574,0.0720492707501277,
-1.50035279911072));
#68834=CARTESIAN_POINT('Ctrl Pts',(-0.226823716508061,0.0693090632846857,
-1.50015644688656));
#68835=CARTESIAN_POINT('Ctrl Pts',(-0.227077608573104,0.0684726541757891,
-1.50009686531871));
#68836=CARTESIAN_POINT('Ctrl Pts',(-0.227515387546249,0.0670012391406965,
-1.49999268975817));
#68837=CARTESIAN_POINT('Ctrl Pts',(-0.227701251991867,0.0663668403783956,
-1.49994798364524));
#68838=CARTESIAN_POINT('Ctrl Pts',(-0.228091569782818,0.0650136511197901,
-1.49985307585601));
#68839=CARTESIAN_POINT('Ctrl Pts',(-0.228295280472651,0.0642946653366138,
-1.49980291676825));
#68840=CARTESIAN_POINT('Ctrl Pts',(-0.228846330875349,0.0623141203021017,
-1.49966545208398));
#68841=CARTESIAN_POINT('Ctrl Pts',(-0.229186640602815,0.0610506077530508,
-1.49957853992801));
#68842=CARTESIAN_POINT('Ctrl Pts',(-0.229925465995759,0.0582142011210711,
-1.49938505447321));
#68843=CARTESIAN_POINT('Ctrl Pts',(-0.230318336993567,0.0566398896464389,
-1.49927877226639));
#68844=CARTESIAN_POINT('Ctrl Pts',(-0.234983752348552,0.0370929145236071,
-1.4979714404334));
#68845=CARTESIAN_POINT('Ctrl Pts',(-0.237158875310678,0.0186829392630581,
-1.49686470085717));
#68846=CARTESIAN_POINT('Ctrl Pts',(-0.237174910684078,0.000205832454907566,
-1.4957269803945));
#68847=CARTESIAN_POINT('Ctrl Pts',(-0.237174910837396,0.000205655715385434,
-1.49572696951183));
#68848=CARTESIAN_POINT('Ctrl Pts',(-0.23718515411427,-0.0116075257210512,
-1.49499957749808));
#68849=CARTESIAN_POINT('Ctrl Pts',(-0.236312832446797,-0.0234039734777036,
-1.49426295624968));
#68850=CARTESIAN_POINT('Ctrl Pts',(-0.234249678855294,-0.0371971188456194,
-1.49336070055333));
#68851=CARTESIAN_POINT('Ctrl Pts',(-0.233905402214962,-0.0393039443191361,
-1.49322177898696));
#68852=CARTESIAN_POINT('Ctrl Pts',(-0.233288649907576,-0.0427824888308832,
-1.49299041613219));
#68853=CARTESIAN_POINT('Ctrl Pts',(-0.233032392784451,-0.0441569847375077,
-1.4928984792637));
#68854=CARTESIAN_POINT('Ctrl Pts',(-0.232549374032932,-0.0466263801682069,
-1.4927323339357));
#68855=CARTESIAN_POINT('Ctrl Pts',(-0.232326992812036,-0.0477221021034335,
-1.49265826547222));
#68856=CARTESIAN_POINT('Ctrl Pts',(-0.231879993566383,-0.0498473625473571,
-1.49251390886118));
#68857=CARTESIAN_POINT('Ctrl Pts',(-0.231656244919416,-0.0508770586564626,
-1.49244364996621));
#68858=CARTESIAN_POINT('Ctrl Pts',(-0.231138381236587,-0.0531860161629698,
-1.49228537244786));
#68859=CARTESIAN_POINT('Ctrl Pts',(-0.230840494736191,-0.0544643871314177,
-1.49219723484231));
#68860=CARTESIAN_POINT('Ctrl Pts',(-0.230011562238014,-0.0578927115593672,
-1.4919594721015));
#68861=CARTESIAN_POINT('Ctrl Pts',(-0.229461001239384,-0.0600377643207175,
-1.49180922453777));
#68862=CARTESIAN_POINT('Ctrl Pts',(-0.226667329155433,-0.0703219593690826,
-1.49108150580196));
#68863=CARTESIAN_POINT('Ctrl Pts',(-0.224020994548223,-0.078344240590904,
-1.49049116571055));
#68864=CARTESIAN_POINT('Ctrl Pts',(-0.217536292916935,-0.0949647457629705,
-1.48921967676172));
#68865=CARTESIAN_POINT('Ctrl Pts',(-0.213602244430633,-0.103510379630981,
-1.48853685472646));
#68866=CARTESIAN_POINT('Ctrl Pts',(-0.202654065488087,-0.123993942641413,
-1.48684137696234));
#68867=CARTESIAN_POINT('Ctrl Pts',(-0.195081844294637,-0.135596112891994,
-1.48582715899228));
#68868=CARTESIAN_POINT('Ctrl Pts',(-0.185086862425553,-0.148325249313563,
-1.48469506267158));
#68869=CARTESIAN_POINT('Ctrl Pts',(-0.183604956647462,-0.150155743061591,
-1.48453180002851));
#68870=CARTESIAN_POINT('Ctrl Pts',(-0.18148198663144,-0.152699664057588,
-1.48430459970435));
#68871=CARTESIAN_POINT('Ctrl Pts',(-0.180863543041265,-0.153431671285566,
-1.48423918693189));
#68872=CARTESIAN_POINT('Ctrl Pts',(-0.179803818540037,-0.154670679733016,
-1.48412843534704));
#68873=CARTESIAN_POINT('Ctrl Pts',(-0.17936479200404,-0.155179585531877,
-1.48408293638605));
#68874=CARTESIAN_POINT('Ctrl Pts',(-0.178510952469771,-0.156160864634009,
-1.48399519681754));
#68875=CARTESIAN_POINT('Ctrl Pts',(-0.178096419711479,-0.156633460998203,
-1.48395293546085));
#68876=CARTESIAN_POINT('Ctrl Pts',(-0.176961809306586,-0.157916668666113,
-1.48383815466504));
#68877=CARTESIAN_POINT('Ctrl Pts',(-0.176238033274916,-0.158724011844247,
-1.48376590464018));
#68878=CARTESIAN_POINT('Ctrl Pts',(-0.173423334868071,-0.161820704265128,
-1.48348851206267));
#68879=CARTESIAN_POINT('Ctrl Pts',(-0.171293030393398,-0.164074048478592,
-1.48328609608841));
#68880=CARTESIAN_POINT('Ctrl Pts',(-0.158280087499714,-0.177308765826556,
-1.48208899933428));
#68881=CARTESIAN_POINT('Ctrl Pts',(-0.146387995992337,-0.187247569120274,
-1.48115337117834));
#68882=CARTESIAN_POINT('Ctrl Pts',(-0.125386894107019,-0.201566879575749,
-1.47959338592066));
#68883=CARTESIAN_POINT('Ctrl Pts',(-0.116817546009545,-0.206651200659605,
-1.47897885270855));
#68884=CARTESIAN_POINT('Ctrl Pts',(-0.104472683996936,-0.212961807546468,
-1.47809983542279));
#68885=CARTESIAN_POINT('Ctrl Pts',(-0.10094736143533,-0.214655306997721,
-1.47784955854477));
#68886=CARTESIAN_POINT('Ctrl Pts',(-0.0946756484998511,-0.217479450113013,
-1.47740434320699));
#68887=CARTESIAN_POINT('Ctrl Pts',(-0.0919468366995563,-0.218647130285726,
-1.47721064681708));
#68888=CARTESIAN_POINT('Ctrl Pts',(-0.0878803065073688,-0.220297642778365,
-1.47692166089365));
#68889=CARTESIAN_POINT('Ctrl Pts',(-0.0865589343164124,-0.220820176677017,
-1.47682770749383));
#68890=CARTESIAN_POINT('Ctrl Pts',(-0.085221778457886,-0.221335106219755,
-1.47673255891512));
#68891=CARTESIAN_POINT('Ctrl Pts',(-0.0852105861826441,-0.221339415313327,
-1.47673176249643));
#68892=CARTESIAN_POINT('Ctrl Pts',(-0.0851876530705312,-0.221348242702754,
-1.47673013061405));
#68893=CARTESIAN_POINT('Ctrl Pts',(-0.0851759122015334,-0.221352760913206,
-1.47672929514757));
#68894=CARTESIAN_POINT('Ctrl Pts',(-0.0851518516321547,-0.221362017886643,
-1.47672758301405));
#68895=CARTESIAN_POINT('Ctrl Pts',(-0.0851395318944815,-0.221366756555765,
-1.47672670634379));
#68896=CARTESIAN_POINT('Ctrl Pts',(-0.0851142813630605,-0.221376466511165,
-1.47672490950785));
#68897=CARTESIAN_POINT('Ctrl Pts',(-0.0851013505310047,-0.221381437692319,
-1.4767239893388));
#68898=CARTESIAN_POINT('Ctrl Pts',(-0.0850748435006703,-0.22139162549623,
-1.47672210306178));
#68899=CARTESIAN_POINT('Ctrl Pts',(-0.0850612672580441,-0.221396842003182,
-1.47672113694993));
#68900=CARTESIAN_POINT('Ctrl Pts',(-0.0850334328468549,-0.22140753410071,
-1.47671915618346));
#68901=CARTESIAN_POINT('Ctrl Pts',(-0.08501917462876,-0.221413009562947,
-1.47671814152451));
#68902=CARTESIAN_POINT('Ctrl Pts',(-0.0849899372882785,-0.221424234089587,
-1.47671606088757));
#68903=CARTESIAN_POINT('Ctrl Pts',(-0.0849749581118485,-0.221429983011144,
-1.47671499490486));
#68904=CARTESIAN_POINT('Ctrl Pts',(-0.084944237279569,-0.221441769913107,
-1.47671280865898));
#68905=CARTESIAN_POINT('Ctrl Pts',(-0.0849284955635096,-0.221447807734861,
-1.47671168839056));
#68906=CARTESIAN_POINT('Ctrl Pts',(-0.0848962052829576,-0.221460188900053,
-1.47670939041271));
#68907=CARTESIAN_POINT('Ctrl Pts',(-0.0848796566516423,-0.22146653206702,
-1.47670821269743));
#68908=CARTESIAN_POINT('Ctrl Pts',(-0.0837731946952754,-0.221890501821456,
-1.47662946843166));
#68909=CARTESIAN_POINT('Ctrl Pts',(-0.0826802311840069,-0.222300072504914,
-1.47655163503368));
#68910=CARTESIAN_POINT('Ctrl Pts',(-0.0803262679976836,-0.223162421462658,
-1.4763838731902));
#68911=CARTESIAN_POINT('Ctrl Pts',(-0.079064370756416,-0.223612613312384,
-1.47629386174449));
#68912=CARTESIAN_POINT('Ctrl Pts',(-0.0756450131076889,-0.224799934340451,
-1.4760497105278));
#68913=CARTESIAN_POINT('Ctrl Pts',(-0.0734806741502606,-0.225516669851043,
-1.47589490520239));
#68914=CARTESIAN_POINT('Ctrl Pts',(-0.061806631537716,-0.229196715682635,
-1.47505823942772));
#68915=CARTESIAN_POINT('Ctrl Pts',(-0.0521289607106422,-0.231589545149481,
-1.47435809973337));
#68916=CARTESIAN_POINT('Ctrl Pts',(-0.0291804723717781,-0.235752196584288,
-1.47268494077267));
#68917=CARTESIAN_POINT('Ctrl Pts',(-0.0158526900075045,-0.237021624268995,
-1.47170261479783));
#68918=CARTESIAN_POINT('Ctrl Pts',(0.00404036154203669,-0.237230495947095,
-1.47025604575925));
#68919=CARTESIAN_POINT('Ctrl Pts',(0.0105713654065964,-0.23702930295838,
-1.46978464202488));
#68920=CARTESIAN_POINT('Ctrl Pts',(0.0207355203658927,-0.23629516781333,
-1.46906363177332));
#68921=CARTESIAN_POINT('Ctrl Pts',(0.0243785750500932,-0.235947148434781,
-1.46880777220532));
#68922=CARTESIAN_POINT('Ctrl Pts',(0.0291183200395713,-0.235383399006347,
-1.46847944830705));
#68923=CARTESIAN_POINT('Ctrl Pts',(0.0302233733893709,-0.23524406244156,
-1.46840322589248));
#68924=CARTESIAN_POINT('Ctrl Pts',(0.0320256527664648,-0.235003902860228,
-1.46827948688433));
#68925=CARTESIAN_POINT('Ctrl Pts',(0.0327234679344847,-0.234907750987677,
-1.46823171814076));
#68926=CARTESIAN_POINT('Ctrl Pts',(0.0340859893669858,-0.234713820042142,
-1.46813873659073));
#68927=CARTESIAN_POINT('Ctrl Pts',(0.0347507231055326,-0.234616323495928,
-1.46809350946589));
#68928=CARTESIAN_POINT('Ctrl Pts',(0.0362387016816675,-0.234391618907756,
-1.46799255717252));
#68929=CARTESIAN_POINT('Ctrl Pts',(0.0370617171350629,-0.234262894391862,
-1.46793691625957));
#68930=CARTESIAN_POINT('Ctrl Pts',(0.0399288806333547,-0.233798964737036,
-1.46774371094434));
#68931=CARTESIAN_POINT('Ctrl Pts',(0.0419693719147703,-0.233441307310008,
-1.46760733407865));
#68932=CARTESIAN_POINT('Ctrl Pts',(0.055943315143799,-0.230802796110215,
-1.46667947043548));
#68933=CARTESIAN_POINT('Ctrl Pts',(0.0676924019440297,-0.22763435623067,
-1.46592938535968));
#68934=CARTESIAN_POINT('Ctrl Pts',(0.0893523920683164,-0.219966602000067,
-1.46451903935053));
#68935=CARTESIAN_POINT('Ctrl Pts',(0.0992971883847658,-0.215659951408117,
-1.46385948749981));
#68936=CARTESIAN_POINT('Ctrl Pts',(0.117010425830783,-0.20650335589636,
-1.46261624934149));
#68937=CARTESIAN_POINT('Ctrl Pts',(0.12485920386034,-0.201854466664892,
-1.46203818975448));
#68938=CARTESIAN_POINT('Ctrl Pts',(0.134232314174322,-0.195546506609168,
-1.46130111270457));
#68939=CARTESIAN_POINT('Ctrl Pts',(0.13602721805316,-0.194302202357451,
-1.46115774134598));
#68940=CARTESIAN_POINT('Ctrl Pts',(0.138867559287086,-0.192274510029199,
-1.46092713351769));
#68941=CARTESIAN_POINT('Ctrl Pts',(0.13992417989916,-0.191506945025557,
-1.46084050363642));
#68942=CARTESIAN_POINT('Ctrl Pts',(0.14191694789207,-0.190034034563014,
-1.46067548263932));
#68943=CARTESIAN_POINT('Ctrl Pts',(0.142854313901792,-0.189330397205168,
-1.46059715962374));
#68944=CARTESIAN_POINT('Ctrl Pts',(0.144977675316932,-0.187711741926462,
-1.46041811350873));
#68945=CARTESIAN_POINT('Ctrl Pts',(0.146160284771637,-0.186792385748309,
-1.46031722127542));
#68946=CARTESIAN_POINT('Ctrl Pts',(0.149778910432317,-0.183923874915833,
-1.46000481192785));
#68947=CARTESIAN_POINT('Ctrl Pts',(0.152185153197636,-0.1819378775954,-1.45979183178573));
#68948=CARTESIAN_POINT('Ctrl Pts',(0.167993145987693,-0.168357672447239,
-1.45835642167721));
#68949=CARTESIAN_POINT('Ctrl Pts',(0.180095960521503,-0.155342268676589,
-1.45707327796906));
#68950=CARTESIAN_POINT('Ctrl Pts',(0.193206272125239,-0.137629934209965,
-1.45546379644826));
#68951=CARTESIAN_POINT('Ctrl Pts',(0.195682311009935,-0.13408615282924,
-1.45514811947415));
#68952=CARTESIAN_POINT('Ctrl Pts',(0.201630114589586,-0.125057542498326,
-1.45436207173725));
#68953=CARTESIAN_POINT('Ctrl Pts',(0.204976417486793,-0.119493814367877,
-1.4538937575076));
#68954=CARTESIAN_POINT('Ctrl Pts',(0.209838731413352,-0.110602726333762,
-1.45317685456136));
#68955=CARTESIAN_POINT('Ctrl Pts',(0.211513188662552,-0.107365873966534,
-1.45292208995909));
#68956=CARTESIAN_POINT('Ctrl Pts',(0.213600586123493,-0.103092225859727,
-1.45259494324688));
#68957=CARTESIAN_POINT('Ctrl Pts',(0.214081649571237,-0.102089494389382,
-1.45251883537212));
#68958=CARTESIAN_POINT('Ctrl Pts',(0.214855710306689,-0.100446503344674,
-1.45239523513154));
#68959=CARTESIAN_POINT('Ctrl Pts',(0.215152934552959,-0.0998082715603084,
-1.4523474916534));
#68960=CARTESIAN_POINT('Ctrl Pts',(0.215728331291025,-0.0985582030945205,
-1.45225451931483));
#68961=CARTESIAN_POINT('Ctrl Pts',(0.21600675135178,-0.0979464941012095,
-1.45220927640747));
#68962=CARTESIAN_POINT('Ctrl Pts',(0.21662480099455,-0.0965731414169772,
-1.45210824755391));
#68963=CARTESIAN_POINT('Ctrl Pts',(0.216963024831639,-0.0958108655488671,
-1.45205254628071));
#68964=CARTESIAN_POINT('Ctrl Pts',(0.218129504727468,-0.0931440442815503,
-1.45185892534696));
#68965=CARTESIAN_POINT('Ctrl Pts',(0.21893678877651,-0.0912303516386376,
-1.45172219992765));
#68966=CARTESIAN_POINT('Ctrl Pts',(0.22426024029244,-0.0781331374932253,
-1.45079982215831));
#68967=CARTESIAN_POINT('Ctrl Pts',(0.227943353732895,-0.0666284086146129,
-1.45005492311008));
#68968=CARTESIAN_POINT('Ctrl Pts',(0.233210055274903,-0.0444901641214075,
-1.44865799371922));
#68969=CARTESIAN_POINT('Ctrl Pts',(0.234978406182421,-0.0339329397472972,
-1.44800655919398));
#68970=CARTESIAN_POINT('Ctrl Pts',(0.236942349735022,-0.0140320890595671,
-1.44676072748228));
#68971=CARTESIAN_POINT('Ctrl Pts',(0.237310355582883,-0.00472661951041226,
-1.44617107144383));
#68972=CARTESIAN_POINT('Ctrl Pts',(0.237088488501456,0.0067714356822805,
-1.44542090502571));
#68973=CARTESIAN_POINT('Ctrl Pts',(0.237015624852722,0.00896642430360502,
-1.44527674927325));
#68974=CARTESIAN_POINT('Ctrl Pts',(0.236850716485898,0.0124672065347807,
-1.44504517755603));
#68975=CARTESIAN_POINT('Ctrl Pts',(0.236778323660225,0.0137738326831459,
-1.44495837729446));
#68976=CARTESIAN_POINT('Ctrl Pts',(0.236620633908695,0.0162489627919629,
-1.44479322268115));
#68977=CARTESIAN_POINT('Ctrl Pts',(0.23653748416878,0.0174175681802019,
-1.44471493803572));
#68978=CARTESIAN_POINT('Ctrl Pts',(0.236328663921222,0.0200741912275866,
-1.44453624626719));
#68979=CARTESIAN_POINT('Ctrl Pts',(0.23619759210099,0.0215617219232392,
-1.44443567249847));
#68980=CARTESIAN_POINT('Ctrl Pts',(0.235751684794361,0.0261286277531596,
-1.44412525207691));
#68981=CARTESIAN_POINT('Ctrl Pts',(0.235390616438148,0.0292030509584075,
-1.44391396923633));
#68982=CARTESIAN_POINT('Ctrl Pts',(0.232511191979616,0.0501695646280451,
-1.44245661140471));
#68983=CARTESIAN_POINT('Ctrl Pts',(0.228015916144205,0.0677269613842048,
-1.44114708661915));
#68984=CARTESIAN_POINT('Ctrl Pts',(0.220164708528558,0.0882897355770886,
-1.43953950784137));
#68985=CARTESIAN_POINT('Ctrl Pts',(0.218664109567756,0.0919433747896704,
-1.43925116649498));
#68986=CARTESIAN_POINT('Ctrl Pts',(0.214440487029725,0.101537919074301,
-1.43848890248179));
#68987=CARTESIAN_POINT('Ctrl Pts',(0.211561832824276,0.107407047668004,
-1.43801727800746));
#68988=CARTESIAN_POINT('Ctrl Pts',(0.20669820461392,0.116366783659128,-1.43729597447291));
#68989=CARTESIAN_POINT('Ctrl Pts',(0.204877773285303,0.119542786422501,
-1.43704003683545));
#68990=CARTESIAN_POINT('Ctrl Pts',(0.202408298040216,0.123628889160507,
-1.43671162902922));
#68991=CARTESIAN_POINT('Ctrl Pts',(0.201825436287929,0.124578147125233,
-1.43663539846692));
#68992=CARTESIAN_POINT('Ctrl Pts',(0.200863085177926,0.12612096512354,-1.43651164958742));
#68993=CARTESIAN_POINT('Ctrl Pts',(0.200487609128549,0.126716989586637,
-1.43646387904636));
#68994=CARTESIAN_POINT('Ctrl Pts',(0.19974885607119,0.127878170400072,-1.43637089683534));
#68995=CARTESIAN_POINT('Ctrl Pts',(0.199385825417262,0.12844346852402,-1.43632567082774));
#68996=CARTESIAN_POINT('Ctrl Pts',(0.198567333545759,0.129706161972041,
-1.43622472396048));
#68997=CARTESIAN_POINT('Ctrl Pts',(0.198110585990482,0.130402723037392,
-1.43616908732682));
#68998=CARTESIAN_POINT('Ctrl Pts',(0.196505415726022,0.132822782033982,
-1.43597591144874));
#68999=CARTESIAN_POINT('Ctrl Pts',(0.195338056591969,0.134533691691649,
-1.43583955926682));
#69000=CARTESIAN_POINT('Ctrl Pts',(0.187165339638882,0.146181123179203,
-1.43491117934512));
#69001=CARTESIAN_POINT('Ctrl Pts',(0.179426473628093,0.155582781967428,
-1.43416061314105));
#69002=CARTESIAN_POINT('Ctrl Pts',(0.163462806086276,0.172192313192935,
-1.432746592364));
#69003=CARTESIAN_POINT('Ctrl Pts',(0.155395452420754,0.179506337252501,
-1.43208389056705));
#69004=CARTESIAN_POINT('Ctrl Pts',(0.139738541951283,0.191852164169122,
-1.43084043988288));
#69005=CARTESIAN_POINT('Ctrl Pts',(0.132307081654853,0.197050552727842,
-1.43026561501085));
#69006=CARTESIAN_POINT('Ctrl Pts',(0.122741654976787,0.202956205718214,
-1.42953219025916));
#69007=CARTESIAN_POINT('Ctrl Pts',(0.120870605688514,0.20407604334043,-1.42938904205155));
#69008=CARTESIAN_POINT('Ctrl Pts',(0.117855328784402,0.205824696630286,
-1.42915870843379));
#69009=CARTESIAN_POINT('Ctrl Pts',(0.116720858855932,0.206470155853359,
-1.42907212702932));
#69010=CARTESIAN_POINT('Ctrl Pts',(0.114557522802467,0.207677463186617,
-1.42890714372396));
#69011=CARTESIAN_POINT('Ctrl Pts',(0.113529702725674,0.20824111328019,-1.42882880946459));
#69012=CARTESIAN_POINT('Ctrl Pts',(0.111177888956655,0.209508246638588,
-1.42864966093714));
#69013=CARTESIAN_POINT('Ctrl Pts',(0.109851329531481,0.210206835338007,
-1.42854867681695));
#69014=CARTESIAN_POINT('Ctrl Pts',(0.105737897788014,0.212323467545589,
-1.42823569213766));
#69015=CARTESIAN_POINT('Ctrl Pts',(0.102929635006296,0.21369896234916,-1.42802222073969));
#69016=CARTESIAN_POINT('Ctrl Pts',(0.0841334307977906,0.222448945924058,
-1.42659410511235));
#69017=CARTESIAN_POINT('Ctrl Pts',(0.0673968609072315,0.228077634589926,
-1.42531962852989));
#69018=CARTESIAN_POINT('Ctrl Pts',(0.0457994821767047,0.232754416960778,
-1.42370567017068));
#69019=CARTESIAN_POINT('Ctrl Pts',(0.0413772883799832,0.233581103960074,
-1.42337713507821));
#69020=CARTESIAN_POINT('Ctrl Pts',(0.0305734752473814,0.235284312741661,
-1.42258208702174));
#69021=CARTESIAN_POINT('Ctrl Pts',(0.024174084774717,0.236027689082033,
-1.4221174941943));
#69022=CARTESIAN_POINT('Ctrl Pts',(0.01413710797081,0.236781045973489,-1.42140554479404));
#69023=CARTESIAN_POINT('Ctrl Pts',(0.0105162383851371,0.236969478690863,
-1.42115210482567));
#69024=CARTESIAN_POINT('Ctrl Pts',(0.00578259343837471,0.237107095192875,
-1.42082638304683));
#69025=CARTESIAN_POINT('Ctrl Pts',(0.00467270794150724,0.237131564538216,
-1.4207504143985));
#69026=CARTESIAN_POINT('Ctrl Pts',(0.00285915130602412,0.237158809495083,
-1.42062698282719));
#69027=CARTESIAN_POINT('Ctrl Pts',(0.00215558294161852,0.237166247941148,
-1.42057927005124));
#69028=CARTESIAN_POINT('Ctrl Pts',(0.000779610703593176,0.237174671771469,
-1.42048630870671));
#69029=CARTESIAN_POINT('Ctrl Pts',(0.000107220803301362,0.237175928888627,
-1.420441046422));
#69030=CARTESIAN_POINT('Ctrl Pts',(-0.00140021851308484,0.237172336748445,
-1.42033992379895));
#69031=CARTESIAN_POINT('Ctrl Pts',(-0.00223526377391046,0.237165936801454,
-1.42028414864492));
#69032=CARTESIAN_POINT('Ctrl Pts',(-0.00515354594639942,0.237128155942764,
-1.42009001796556));
#69033=CARTESIAN_POINT('Ctrl Pts',(-0.00723646033378336,0.237073734831898,
-1.41995286493257));
#69034=CARTESIAN_POINT('Ctrl Pts',(-0.0202610147860963,0.236561611929272,
-1.41910253015864));
#69035=CARTESIAN_POINT('Ctrl Pts',(-0.0311607401173676,0.235373990943297,
-1.41842278355567));
#69036=CARTESIAN_POINT('Ctrl Pts',(-0.0419392748056671,0.233437524519463,
-1.41774927189049));
#69037=CARTESIAN_POINT('Origin',(0.,0.,-2.1456589891905));
#69038=CARTESIAN_POINT('',(-0.0419392737720405,0.233437524705164,-1.29816138490414));
#69039=CARTESIAN_POINT('',(-0.0419392741368905,0.233437524639615,-1.31805175208418));
#69040=CARTESIAN_POINT('',(-0.0419392741328076,0.233437524640348,-2.1456589891905));
#69041=CARTESIAN_POINT('Ctrl Pts',(-0.0419392737720407,0.233437524705164,
-1.29816138490414));
#69042=CARTESIAN_POINT('Ctrl Pts',(-0.0318728565423017,0.235246052398536,
-1.29878870397928));
#69043=CARTESIAN_POINT('Ctrl Pts',(-0.0216995162353172,0.236401635171646,
-1.29941285583831));
#69044=CARTESIAN_POINT('Ctrl Pts',(-0.0024103744417276,0.237336633302986,
-1.30061709041487));
#69045=CARTESIAN_POINT('Ctrl Pts',(0.00667910759640316,0.237254816497144,
-1.30119317327307));
#69046=CARTESIAN_POINT('Ctrl Pts',(0.0179183508302511,0.236507242965848,
-1.30192804875745));
#69047=CARTESIAN_POINT('Ctrl Pts',(0.0200937231710433,0.236332361386772,
-1.30207131475618));
#69048=CARTESIAN_POINT('Ctrl Pts',(0.0235664635680065,0.236004889438547,
-1.3023018119501));
#69049=CARTESIAN_POINT('Ctrl Pts',(0.024865555383796,0.235871554206155,
-1.30238843792096));
#69050=CARTESIAN_POINT('Ctrl Pts',(0.0273288910901284,0.23559814791868,
-1.30255348974753));
#69051=CARTESIAN_POINT('Ctrl Pts',(0.0284933303413513,0.235460157206682,
-1.30263184777442));
#69052=CARTESIAN_POINT('Ctrl Pts',(0.0311442927438584,0.235126055116324,
-1.30281102806703));
#69053=CARTESIAN_POINT('Ctrl Pts',(0.0326300629188021,0.234924472073839,
-1.30291202008764));
#69054=CARTESIAN_POINT('Ctrl Pts',(0.0372071763632039,0.234259210752228,
-1.30322494625904));
#69055=CARTESIAN_POINT('Ctrl Pts',(0.0402912332081526,0.23374851164379,
-1.30343834998415));
#69056=CARTESIAN_POINT('Ctrl Pts',(0.0606950674918734,0.229953989604255,
-1.30486787521392));
#69057=CARTESIAN_POINT('Ctrl Pts',(0.0776095034816172,0.224809406618693,
-1.30614399388456));
#69058=CARTESIAN_POINT('Ctrl Pts',(0.102686612660891,0.214012066510612,
-1.30813810224086));
#69059=CARTESIAN_POINT('Ctrl Pts',(0.111336286194037,0.209642450517734,
-1.30884529806275));
#69060=CARTESIAN_POINT('Ctrl Pts',(0.122395508431192,0.203177519984765,
-1.30975809664146));
#69061=CARTESIAN_POINT('Ctrl Pts',(0.125064611282575,0.201545553441463,
-1.30997905753906));
#69062=CARTESIAN_POINT('Ctrl Pts',(0.12953093611788,0.198691806902404,-1.31034898631507));
#69063=CARTESIAN_POINT('Ctrl Pts',(0.131345028471709,0.19749729587155,-1.31049929311839));
#69064=CARTESIAN_POINT('Ctrl Pts',(0.133899218734225,0.19576469518554,-1.31071071533704));
#69065=CARTESIAN_POINT('Ctrl Pts',(0.134652944125372,0.195247026525157,
-1.31077307874387));
#69066=CARTESIAN_POINT('Ctrl Pts',(0.13594950503168,0.194345451959674,-1.31088028541602));
#69067=CARTESIAN_POINT('Ctrl Pts',(0.136493749002289,0.193963602629301,
-1.31092526404964));
#69068=CARTESIAN_POINT('Ctrl Pts',(0.137636544001775,0.193154609187066,
-1.31101965370857));
#69069=CARTESIAN_POINT('Ctrl Pts',(0.13823472076293,0.192726965699511,-1.31106903018319));
#69070=CARTESIAN_POINT('Ctrl Pts',(0.139846947296754,0.191562998444501,
-1.31120205827568));
#69071=CARTESIAN_POINT('Ctrl Pts',(0.140857183313191,0.190821395869145,
-1.31128535771404));
#69072=CARTESIAN_POINT('Ctrl Pts',(0.145573130683965,0.187301613002203,
-1.31167419120482));
#69073=CARTESIAN_POINT('Ctrl Pts',(0.149203101246535,0.18442307880345,-1.31197342557776));
#69074=CARTESIAN_POINT('Ctrl Pts',(0.155163216788652,0.179405504003362,
-1.31246908424052));
#69075=CARTESIAN_POINT('Ctrl Pts',(0.157538926960821,0.177323000920065,
-1.31266788326903));
#69076=CARTESIAN_POINT('Ctrl Pts',(0.170976909111297,0.165060208632435,
-1.31380424178202));
#69077=CARTESIAN_POINT('Ctrl Pts',(0.181093084635821,0.153893808827574,
-1.31470935671998));
#69078=CARTESIAN_POINT('Ctrl Pts',(0.196364816361512,0.133428316553375,
-1.31629290456829));
#69079=CARTESIAN_POINT('Ctrl Pts',(0.202078559425883,0.124605260854633,
-1.31695511577607));
#69080=CARTESIAN_POINT('Ctrl Pts',(0.20829081268262,0.113455043740425,-1.31778710713011));
#69081=CARTESIAN_POINT('Ctrl Pts',(0.209364631289577,0.111461025390306,
-1.31793568098041));
#69082=CARTESIAN_POINT('Ctrl Pts',(0.211020599189383,0.10827760489307,-1.31817270052789));
#69083=CARTESIAN_POINT('Ctrl Pts',(0.211621643640911,0.107098145762735,
-1.31826047827057));
#69084=CARTESIAN_POINT('Ctrl Pts',(0.212735047343839,0.104867287953199,
-1.31842646319314));
#69085=CARTESIAN_POINT('Ctrl Pts',(0.213249566190888,0.103817006727997,
-1.31850459184072));
#69086=CARTESIAN_POINT('Ctrl Pts',(0.214393111044191,0.10143833003414,-1.31868152279029));
#69087=CARTESIAN_POINT('Ctrl Pts',(0.215017593996348,0.100107816707867,
-1.31878047895287));
#69088=CARTESIAN_POINT('Ctrl Pts',(0.216826650429969,0.0961584407935901,
-1.31907422995178));
#69089=CARTESIAN_POINT('Ctrl Pts',(0.217975992875584,0.0935238329877993,
-1.31927021683345));
#69090=CARTESIAN_POINT('Ctrl Pts',(0.226682940753395,0.0725321709673598,
-1.32083262915924));
#69091=CARTESIAN_POINT('Ctrl Pts',(0.231955037949759,0.0533161961942209,
-1.32227791060544));
#69092=CARTESIAN_POINT('Ctrl Pts',(0.235948576275878,0.0254730994360653,
-1.32433082673592));
#69093=CARTESIAN_POINT('Ctrl Pts',(0.236694376928316,0.017216236257691,
-1.32493317461051));
#69094=CARTESIAN_POINT('Ctrl Pts',(0.237166923880965,0.00468417668534722,
-1.32582434843599));
#69095=CARTESIAN_POINT('Ctrl Pts',(0.237212803024866,0.000427656028375762,
-1.32612298124362));
#69096=CARTESIAN_POINT('Ctrl Pts',(0.237125169022792,-0.00500111645075131,
-1.3264968511908));
#69097=CARTESIAN_POINT('Ctrl Pts',(0.23709753001091,-0.00617400646635365,
-1.32657720792946));
#69098=CARTESIAN_POINT('Ctrl Pts',(0.237038958680632,-0.00806397607175334,
-1.3267059679238));
#69099=CARTESIAN_POINT('Ctrl Pts',(0.237013473121604,-0.00878118649158647,
-1.32675466170852));
#69100=CARTESIAN_POINT('Ctrl Pts',(0.236958117025209,-0.010162336191754,
-1.32684809399495));
#69101=CARTESIAN_POINT('Ctrl Pts',(0.236928710869638,-0.0108262772136131,
-1.32689285617956));
#69102=CARTESIAN_POINT('Ctrl Pts',(0.236857577223833,-0.0122928722308543,
-1.32699141164523));
#69103=CARTESIAN_POINT('Ctrl Pts',(0.236814559276926,-0.0130954632416445,
-1.32704513390151));
#69104=CARTESIAN_POINT('Ctrl Pts',(0.236647806088015,-0.0159363179718838,
-1.32723458790831));
#69105=CARTESIAN_POINT('Ctrl Pts',(0.236501824776447,-0.0179732558570746,
-1.32736915024778));
#69106=CARTESIAN_POINT('Ctrl Pts',(0.235081904851881,-0.0347448833719733,
-1.32846843083687));
#69107=CARTESIAN_POINT('Ctrl Pts',(0.232458404305983,-0.0493348075127487,
-1.3293707771645));
#69108=CARTESIAN_POINT('Ctrl Pts',(0.225417108335508,-0.074636901487737,
-1.33098035651496));
#69109=CARTESIAN_POINT('Ctrl Pts',(0.221544629299971,-0.0854487639734451,
-1.33168362053006));
#69110=CARTESIAN_POINT('Ctrl Pts',(0.215184927706626,-0.0998274523309159,
-1.33267730220626));
#69111=CARTESIAN_POINT('Ctrl Pts',(0.213360110607767,-0.10367031071428,
-1.33294880295714));
#69112=CARTESIAN_POINT('Ctrl Pts',(0.209986809922639,-0.110307336863774,
-1.3334298702877));
#69113=CARTESIAN_POINT('Ctrl Pts',(0.20848335008671,-0.113123207446429,
-1.33363793069504));
#69114=CARTESIAN_POINT('Ctrl Pts',(0.206184767297774,-0.117226736981188,
-1.3339474817845));
#69115=CARTESIAN_POINT('Ctrl Pts',(0.205433374906296,-0.118538577794571,
-1.33404741701478));
#69116=CARTESIAN_POINT('Ctrl Pts',(0.204076267862656,-0.120856261348862,
-1.33422576680816));
#69117=CARTESIAN_POINT('Ctrl Pts',(0.203475523510242,-0.121864967316903,
-1.33430399952499));
#69118=CARTESIAN_POINT('Ctrl Pts',(0.202194301645057,-0.123980372511511,
-1.33446938013217));
#69119=CARTESIAN_POINT('Ctrl Pts',(0.201512172553515,-0.125086020729689,
-1.33455658668214));
#69120=CARTESIAN_POINT('Ctrl Pts',(0.19967651071696,-0.128007418389305,
-1.33478909001379));
#69121=CARTESIAN_POINT('Ctrl Pts',(0.198507322310904,-0.129813137053506,
-1.33493496195895));
#69122=CARTESIAN_POINT('Ctrl Pts',(0.193092686939065,-0.137931378491709,
-1.33560085850526));
#69123=CARTESIAN_POINT('Ctrl Pts',(0.188570024744863,-0.144052679399986,
-1.33613119987034));
#69124=CARTESIAN_POINT('Ctrl Pts',(0.173903888267402,-0.162026343238043,
-1.33777777351593));
#69125=CARTESIAN_POINT('Ctrl Pts',(0.162879660220001,-0.173104655240237,
-1.33892334399001));
#69126=CARTESIAN_POINT('Ctrl Pts',(0.145585768374689,-0.187358753403299,
-1.34055434621625));
#69127=CARTESIAN_POINT('Ctrl Pts',(0.140136450290107,-0.191468812744281,
-1.34104741838494));
#69128=CARTESIAN_POINT('Ctrl Pts',(0.131416419089888,-0.197473744069596,
-1.34179712653934));
#69129=CARTESIAN_POINT('Ctrl Pts',(0.128265037058233,-0.199535057094684,
-1.34206056531066));
#69130=CARTESIAN_POINT('Ctrl Pts',(0.124109648538934,-0.202113932843209,
-1.34239703749904));
#69131=CARTESIAN_POINT('Ctrl Pts',(0.123149361223076,-0.2027004727848,-1.34247405592901));
#69132=CARTESIAN_POINT('Ctrl Pts',(0.121578893509951,-0.203644428404196,
-1.34259877010456));
#69133=CARTESIAN_POINT('Ctrl Pts',(0.120971238818345,-0.204005980253957,
-1.34264672518083));
#69134=CARTESIAN_POINT('Ctrl Pts',(0.119784229925712,-0.204705076740272,
-1.34273980511593));
#69135=CARTESIAN_POINT('Ctrl Pts',(0.119205049184147,-0.205042889286391,
-1.34278494610547));
#69136=CARTESIAN_POINT('Ctrl Pts',(0.117908058854139,-0.205792018040861,
-1.34288543551574));
#69137=CARTESIAN_POINT('Ctrl Pts',(0.117189506591715,-0.206202048069211,
-1.34294070233705));
#69138=CARTESIAN_POINT('Ctrl Pts',(0.114694105301188,-0.207608750484607,
-1.34313128551846));
#69139=CARTESIAN_POINT('Ctrl Pts',(0.112906510590903,-0.208586316949343,
-1.34326545643358));
#69140=CARTESIAN_POINT('Ctrl Pts',(0.0988281324601051,-0.216051207410918,
-1.34430562031925));
#69141=CARTESIAN_POINT('Ctrl Pts',(0.0859995524639044,-0.221470781655309,
-1.34515687352145));
#69142=CARTESIAN_POINT('Ctrl Pts',(0.0562006729503547,-0.231076797054721,
-1.34707588083529));
#69143=CARTESIAN_POINT('Ctrl Pts',(0.0390974139453236,-0.234576845660657,
-1.3481411629216));
#69144=CARTESIAN_POINT('Ctrl Pts',(0.0191139479844233,-0.236418551702822,
-1.34944404144082));
#69145=CARTESIAN_POINT('Ctrl Pts',(0.0164578992359098,-0.236618281658662,
-1.34961825459668));
#69146=CARTESIAN_POINT('Ctrl Pts',(0.0123934301455407,-0.236855158761854,
-1.34988670167322));
#69147=CARTESIAN_POINT('Ctrl Pts',(0.0109870498319288,-0.236924561695109,
-1.34997992727444));
#69148=CARTESIAN_POINT('Ctrl Pts',(0.00842641519950863,-0.237028077354934,
-1.35015031813964));
#69149=CARTESIAN_POINT('Ctrl Pts',(0.00727236299628516,-0.237066291536844,
-1.35022735253578));
#69150=CARTESIAN_POINT('Ctrl Pts',(0.00475220155882484,-0.237131322504469,
-1.35039612377189));
#69151=CARTESIAN_POINT('Ctrl Pts',(0.00338605444781345,-0.237154763881754,
-1.35048796355386));
#69152=CARTESIAN_POINT('Ctrl Pts',(-0.000376626373560403,-0.23718680840193,
-1.35074191567724));
#69153=CARTESIAN_POINT('Ctrl Pts',(-0.00277314986803306,-0.237170893728291,
-1.35090478611391));
#69154=CARTESIAN_POINT('Ctrl Pts',(-0.0202806608630571,-0.23678924777322,
-1.35210321463882));
#69155=CARTESIAN_POINT('Ctrl Pts',(-0.0353234499490055,-0.235016066115311,
-1.35318313313352));
#69156=CARTESIAN_POINT('Ctrl Pts',(-0.0616875174485937,-0.229319311422092,
-1.35514652493496));
#69157=CARTESIAN_POINT('Ctrl Pts',(-0.0730781341977933,-0.225947546942119,
-1.35601868456264));
#69158=CARTESIAN_POINT('Ctrl Pts',(-0.0897529703027928,-0.219617987423714,
-1.35729902081691));
#69159=CARTESIAN_POINT('Ctrl Pts',(-0.0952555907767075,-0.217287924551768,
-1.35772192455968));
#69160=CARTESIAN_POINT('Ctrl Pts',(-0.101843096852828,-0.214200041048182,
-1.35822397525818));
#69161=CARTESIAN_POINT('Ctrl Pts',(-0.103016824081451,-0.213638030582018,
-1.3583132582707));
#69162=CARTESIAN_POINT('Ctrl Pts',(-0.104855940123149,-0.2127387335393,
-1.35845282009326));
#69163=CARTESIAN_POINT('Ctrl Pts',(-0.105524443558607,-0.212407930119331,
-1.35850347921444));
#69164=CARTESIAN_POINT('Ctrl Pts',(-0.106783079708057,-0.211777695694204,
-1.3585987097302));
#69165=CARTESIAN_POINT('Ctrl Pts',(-0.107373516308844,-0.211478950518598,
-1.35864331898204));
#69166=CARTESIAN_POINT('Ctrl Pts',(-0.108743973514942,-0.210778316581784,
-1.35874672376161));
#69167=CARTESIAN_POINT('Ctrl Pts',(-0.109523023891553,-0.21037456551568,
-1.35880540252259));
#69168=CARTESIAN_POINT('Ctrl Pts',(-0.112081475832221,-0.209030556698077,
-1.35899782775761));
#69169=CARTESIAN_POINT('Ctrl Pts',(-0.113851208940743,-0.208071943675324,
-1.35913048436589));
#69170=CARTESIAN_POINT('Ctrl Pts',(-0.128906197390237,-0.199667488174845,
-1.36025699421414));
#69171=CARTESIAN_POINT('Ctrl Pts',(-0.141459878144863,-0.190979449466593,
-1.36118442651156));
#69172=CARTESIAN_POINT('Ctrl Pts',(-0.161639891119704,-0.173924401410632,
-1.36280382106334));
#69173=CARTESIAN_POINT('Ctrl Pts',(-0.16966275991616,-0.166107418033556,
-1.36349063718634));
#69174=CARTESIAN_POINT('Ctrl Pts',(-0.179892323263126,-0.154623128759083,
-1.36446318701204));
#69175=CARTESIAN_POINT('Ctrl Pts',(-0.182597445506285,-0.15141905330792,
-1.36473093215617));
#69176=CARTESIAN_POINT('Ctrl Pts',(-0.187187918017403,-0.145679886293315,
-1.3652059453144));
#69177=CARTESIAN_POINT('Ctrl Pts',(-0.189110226393582,-0.143175649690379,
-1.36541176078678));
#69178=CARTESIAN_POINT('Ctrl Pts',(-0.191874430459063,-0.139421839070389,
-1.36571860120614));
#69179=CARTESIAN_POINT('Ctrl Pts',(-0.192755373022699,-0.138201346842064,
-1.3658181105055));
#69180=CARTESIAN_POINT('Ctrl Pts',(-0.194302200536161,-0.136014749329729,
-1.36599598390912));
#69181=CARTESIAN_POINT('Ctrl Pts',(-0.194972651829061,-0.135051923800692,
-1.36607416972506));
#69182=CARTESIAN_POINT('Ctrl Pts',(-0.196372379931966,-0.133009646320417,
-1.36623974610283));
#69183=CARTESIAN_POINT('Ctrl Pts',(-0.197099959917208,-0.131929084350244,
-1.36632719750948));
#69184=CARTESIAN_POINT('Ctrl Pts',(-0.199014322998506,-0.129034793056295,
-1.36656106012519));
#69185=CARTESIAN_POINT('Ctrl Pts',(-0.20018518325261,-0.127210732406274,
-1.36670805848678));
#69186=CARTESIAN_POINT('Ctrl Pts',(-0.20546983525563,-0.118724208131854,
-1.36739039644434));
#69187=CARTESIAN_POINT('Ctrl Pts',(-0.209276680072112,-0.111877333672706,
-1.3679367073092));
#69188=CARTESIAN_POINT('Ctrl Pts',(-0.220242475636262,-0.0896291922228234,
-1.369699207038));
#69189=CARTESIAN_POINT('Ctrl Pts',(-0.226090417077609,-0.0736420839027499,
-1.3709513432726));
#69190=CARTESIAN_POINT('Ctrl Pts',(-0.231556805039093,-0.0516331267031599,
-1.37259524400254));
#69191=CARTESIAN_POINT('Ctrl Pts',(-0.232731946391666,-0.0460476223073438,
-1.37300537014251));
#69192=CARTESIAN_POINT('Ctrl Pts',(-0.234088995878537,-0.0382022299993802,
-1.37356727587456));
#69193=CARTESIAN_POINT('Ctrl Pts',(-0.234441737759472,-0.0359741684758743,
-1.37372527399775));
#69194=CARTESIAN_POINT('Ctrl Pts',(-0.235003462666067,-0.032065844513887,
-1.37399928675627));
#69195=CARTESIAN_POINT('Ctrl Pts',(-0.235226336770555,-0.0303877730415673,
-1.37411592904399));
#69196=CARTESIAN_POINT('Ctrl Pts',(-0.23553137299862,-0.0278861513270842,
-1.37428817807476));
#69197=CARTESIAN_POINT('Ctrl Pts',(-0.235627216419629,-0.0270643684048602,
-1.37434449940631));
#69198=CARTESIAN_POINT('Ctrl Pts',(-0.235784285608267,-0.0256534990311193,
-1.37444072472845));
#69199=CARTESIAN_POINT('Ctrl Pts',(-0.235847607184581,-0.0250646676608368,
-1.37448074375953));
#69200=CARTESIAN_POINT('Ctrl Pts',(-0.235987429711496,-0.0237169836300684,
-1.37457201246847));
#69201=CARTESIAN_POINT('Ctrl Pts',(-0.236062476539668,-0.0229579943710578,
-1.37462318037575));
#69202=CARTESIAN_POINT('Ctrl Pts',(-0.236259470637116,-0.0208625069446904,
-1.37476384003465));
#69203=CARTESIAN_POINT('Ctrl Pts',(-0.236373739881703,-0.019525290370001,
-1.37485291734278));
#69204=CARTESIAN_POINT('Ctrl Pts',(-0.236938100357669,-0.0121872429385602,
-1.37533834460322));
#69205=CARTESIAN_POINT('Ctrl Pts',(-0.23717107801787,-0.00617137255013728,
-1.37572390747684));
#69206=CARTESIAN_POINT('Ctrl Pts',(-0.237185663879248,0.0164961723705386,
-1.37715177446449));
#69207=CARTESIAN_POINT('Ctrl Pts',(-0.235443376631179,0.0331005582226649,
-1.37815009812945));
#69208=CARTESIAN_POINT('Ctrl Pts',(-0.229819634506442,0.0595162181980795,
-1.37982509561166));
#69209=CARTESIAN_POINT('Ctrl Pts',(-0.227002126689017,0.0694927282228469,
-1.38047813891077));
#69210=CARTESIAN_POINT('Ctrl Pts',(-0.222773324296751,0.0814206274086489,
-1.38130250023246));
#69211=CARTESIAN_POINT('Ctrl Pts',(-0.221973151845707,0.0835774601011955,
-1.38145332930051));
#69212=CARTESIAN_POINT('Ctrl Pts',(-0.220655730281342,0.0869760749368039,
-1.38169397737837));
#69213=CARTESIAN_POINT('Ctrl Pts',(-0.22015905901245,0.0882257191863792,
-1.3817831077328));
#69214=CARTESIAN_POINT('Ctrl Pts',(-0.219211491722091,0.0905520007675374,
-1.38195027226123));
#69215=CARTESIAN_POINT('Ctrl Pts',(-0.218763220562161,0.0916296687289643,
-1.38202821575225));
#69216=CARTESIAN_POINT('Ctrl Pts',(-0.217744262228406,0.0940291966348703,
-1.38220291374211));
#69217=CARTESIAN_POINT('Ctrl Pts',(-0.217169459997576,0.0953492477078107,
-1.38229980599598));
#69218=CARTESIAN_POINT('Ctrl Pts',(-0.215433515662661,0.0992387582484171,
-1.38258767710358));
#69219=CARTESIAN_POINT('Ctrl Pts',(-0.214238567629329,0.101792758849093,
-1.38277980488933));
#69220=CARTESIAN_POINT('Ctrl Pts',(-0.208569341916651,0.113367538751907,
-1.3836651786895));
#69221=CARTESIAN_POINT('Ctrl Pts',(-0.203569508197109,0.12211787820237,
-1.38437636179456));
#69222=CARTESIAN_POINT('Ctrl Pts',(-0.189541261975669,0.143401510018687,
-1.38621133985064));
#69223=CARTESIAN_POINT('Ctrl Pts',(-0.17981757480942,0.15542036194543,-1.38735081068616));
#69224=CARTESIAN_POINT('Ctrl Pts',(-0.164345785805216,0.171132625022037,
-1.38893927386564));
#69225=CARTESIAN_POINT('Ctrl Pts',(-0.159498851202622,0.175658893310532,
-1.38941031312268));
#69226=CARTESIAN_POINT('Ctrl Pts',(-0.153423819071305,0.18087290157415,
-1.38996355463857));
#69227=CARTESIAN_POINT('Ctrl Pts',(-0.152371633739448,0.181760172316185,
-1.39005809489226));
#69228=CARTESIAN_POINT('Ctrl Pts',(-0.150718488115591,0.18312976685428,
-1.39020457041831));
#69229=CARTESIAN_POINT('Ctrl Pts',(-0.150122820799587,0.183618389290984,
-1.39025693781813));
#69230=CARTESIAN_POINT('Ctrl Pts',(-0.14901467226277,0.184518399934664,
-1.39035358370004));
#69231=CARTESIAN_POINT('Ctrl Pts',(-0.148502862725296,0.184930560598091,
-1.39039791528265));
#69232=CARTESIAN_POINT('Ctrl Pts',(-0.14732314457597,0.185872532782397,
-1.39049940824487));
#69233=CARTESIAN_POINT('Ctrl Pts',(-0.14665408651702,0.186400875360567,
-1.39055646570941));
#69234=CARTESIAN_POINT('Ctrl Pts',(-0.144544920422733,0.18804805826034,
-1.39073481705062));
#69235=CARTESIAN_POINT('Ctrl Pts',(-0.143094707450883,0.189153935820108,
-1.39085524255602));
#69236=CARTESIAN_POINT('Ctrl Pts',(-0.139638856142722,0.19172674268913,
-1.39113743757307));
#69237=CARTESIAN_POINT('Ctrl Pts',(-0.137622604812363,0.193179123387222,
-1.39129835748516));
#69238=CARTESIAN_POINT('Ctrl Pts',(-0.130147561610856,0.198387226734763,
-1.3918829584528));
#69239=CARTESIAN_POINT('Ctrl Pts',(-0.124554568153433,0.201945665591074,
-1.39229741389112));
#69240=CARTESIAN_POINT('Ctrl Pts',(-0.116663997406113,0.206513184762994,
-1.39286162901114));
#69241=CARTESIAN_POINT('Ctrl Pts',(-0.114488924788223,0.207726912520161,
-1.39301509919563));
#69242=CARTESIAN_POINT('Ctrl Pts',(-0.0949889995657393,0.218208873400792,
-1.39437612568214));
#69243=CARTESIAN_POINT('Ctrl Pts',(-0.0765961291658136,0.225324152174435,
-1.39556460958456));
#69244=CARTESIAN_POINT('Ctrl Pts',(-0.0547249015365923,0.230793346803669,
-1.39702461114125));
#69245=CARTESIAN_POINT('Ctrl Pts',(-0.0519001250913411,0.231444938589804,
-1.39721385423976));
#69246=CARTESIAN_POINT('Ctrl Pts',(-0.0476212369053222,0.232349679773836,
-1.39750187036786));
#69247=CARTESIAN_POINT('Ctrl Pts',(-0.0461754744523153,0.232641314664901,
-1.39759941697803));
#69248=CARTESIAN_POINT('Ctrl Pts',(-0.0437988604473316,0.233097691697676,
-1.39776018666513));
#69249=CARTESIAN_POINT('Ctrl Pts',(-0.0428695642994561,0.233270389153531,
-1.39782315466176));
#69250=CARTESIAN_POINT('Ctrl Pts',(-0.0419392741322232,0.233437524640453,
-1.39788629978594));
#69251=CARTESIAN_POINT('Ctrl Pts',(-0.0419392748056671,0.233437524519463,
-1.41774927189049));
#69252=CARTESIAN_POINT('Ctrl Pts',(-0.0429471299453534,0.233256453743654,
-1.41768629466649));
#69253=CARTESIAN_POINT('Ctrl Pts',(-0.0439539256977684,0.233068835573067,
-1.41762337549457));
#69254=CARTESIAN_POINT('Ctrl Pts',(-0.0553224712183252,0.230873984485438,
-1.41691253152495));
#69255=CARTESIAN_POINT('Ctrl Pts',(-0.06554011284678,0.228183825399038,
-1.41626953355095));
#69256=CARTESIAN_POINT('Ctrl Pts',(-0.0845470134801674,0.221797166627857,
-1.41502133823456));
#69257=CARTESIAN_POINT('Ctrl Pts',(-0.0933589172298425,0.21823441694041,
-1.41442000382171));
#69258=CARTESIAN_POINT('Ctrl Pts',(-0.103926582184271,0.21320441263141,
-1.41365666145969));
#69259=CARTESIAN_POINT('Ctrl Pts',(-0.105906886730761,0.212227676923995,
-1.41351173996655));
#69260=CARTESIAN_POINT('Ctrl Pts',(-0.109040949761314,0.210627090303489,
-1.41327922726768));
#69261=CARTESIAN_POINT('Ctrl Pts',(-0.110203701302611,0.210021056079053,
-1.41319226071762));
#69262=CARTESIAN_POINT('Ctrl Pts',(-0.112395315967638,0.208855560161318,
-1.41302697402601));
#69263=CARTESIAN_POINT('Ctrl Pts',(-0.113425180465265,0.208298056672012,
-1.4129487251493));
#69264=CARTESIAN_POINT('Ctrl Pts',(-0.115754902574239,0.207014491955191,
-1.41277037102908));
#69265=CARTESIAN_POINT('Ctrl Pts',(-0.117052126120474,0.206283777704563,
-1.41267010151584));
#69266=CARTESIAN_POINT('Ctrl Pts',(-0.12100477299107,0.204007999381784,
-1.41236157398488));
#69267=CARTESIAN_POINT('Ctrl Pts',(-0.123637036916123,0.202423566950073,
-1.41215190508976));
#69268=CARTESIAN_POINT('Ctrl Pts',(-0.14168873956102,0.191074287202917,
-1.41068384569535));
#69269=CARTESIAN_POINT('Ctrl Pts',(-0.155964082793625,0.179610800336821,
-1.40936050605517));
#69270=CARTESIAN_POINT('Ctrl Pts',(-0.171438256427541,0.16393658487103,
-1.40775186298924));
#69271=CARTESIAN_POINT('Ctrl Pts',(-0.174030178785387,0.161182434296163,
-1.40747580711049));
#69272=CARTESIAN_POINT('Ctrl Pts',(-0.180927865979405,0.153492582535266,
-1.40672462599093));
#69273=CARTESIAN_POINT('Ctrl Pts',(-0.185097094813663,0.148438346239104,
-1.40625189756647));
#69274=CARTESIAN_POINT('Ctrl Pts',(-0.191265397099604,0.140295987032012,
-1.40552912763804));
#69275=CARTESIAN_POINT('Ctrl Pts',(-0.193410895170719,0.1373231422284,-1.40527279989218));
#69276=CARTESIAN_POINT('Ctrl Pts',(-0.196117824728577,0.133382987960167,
-1.40494397285027));
#69277=CARTESIAN_POINT('Ctrl Pts',(-0.196742428822608,0.132459954242744,
-1.40486770161186));
#69278=CARTESIAN_POINT('Ctrl Pts',(-0.197751246559312,0.130946254226803,
-1.40474390345106));
#69279=CARTESIAN_POINT('Ctrl Pts',(-0.198139366648698,0.130358231151531,
-1.40469612393591));
#69280=CARTESIAN_POINT('Ctrl Pts',(-0.198892400805194,0.129206210193456,
-1.40460313841397));
#69281=CARTESIAN_POINT('Ctrl Pts',(-0.199257547194572,0.128642379306804,
-1.4045579179733));
#69282=CARTESIAN_POINT('Ctrl Pts',(-0.200069914758296,0.127376226476415,
-1.40445699815584));
#69283=CARTESIAN_POINT('Ctrl Pts',(-0.200515847591602,0.126673078352879,
-1.40440138285757));
#69284=CARTESIAN_POINT('Ctrl Pts',(-0.202057029098631,0.124214407135713,
-1.40420835368872));
#69285=CARTESIAN_POINT('Ctrl Pts',(-0.203133038189173,0.122446851567583,
-1.40407212451938));
#69286=CARTESIAN_POINT('Ctrl Pts',(-0.210398053986977,0.110153239504552,
-1.40314038635887));
#69287=CARTESIAN_POINT('Ctrl Pts',(-0.215790055530291,0.0991756341979563,
-1.40238672240567));
#69288=CARTESIAN_POINT('Ctrl Pts',(-0.224366071248034,0.0776636051631953,
-1.40096535398361));
#69289=CARTESIAN_POINT('Ctrl Pts',(-0.227710469400293,0.0672287226322368,
-1.40029846074522));
#69290=CARTESIAN_POINT('Ctrl Pts',(-0.23173807816398,0.0508393571751145,
-1.39924548116094));
#69291=CARTESIAN_POINT('Ctrl Pts',(-0.232937127973371,0.0450273680455295,
-1.39887118490579));
#69292=CARTESIAN_POINT('Ctrl Pts',(-0.234594034787844,0.0351343118694262,
-1.39822768237138));
#69293=CARTESIAN_POINT('Ctrl Pts',(-0.235166141860016,0.0310751267202716,
-1.39796187696801));
#69294=CARTESIAN_POINT('Ctrl Pts',(-0.235822529548355,0.0253474491833521,
-1.39758335393401));
#69295=CARTESIAN_POINT('Ctrl Pts',(-0.235994829399859,0.02368963660025,
-1.39747339153144));
#69296=CARTESIAN_POINT('Ctrl Pts',(-0.236260910537195,0.0208374146375821,
-1.39728344957301));
#69297=CARTESIAN_POINT('Ctrl Pts',(-0.23636314237732,0.0196438420905053,
-1.39720373787824));
#69298=CARTESIAN_POINT('Ctrl Pts',(-0.236541317896038,0.0173602798973365,
-1.39705077733226));
#69299=CARTESIAN_POINT('Ctrl Pts',(-0.236618780331892,0.0162704368460603,
-1.39697757828265));
#69300=CARTESIAN_POINT('Ctrl Pts',(-0.236782862912788,0.0137120570755085,
-1.39680526371827));
#69301=CARTESIAN_POINT('Ctrl Pts',(-0.23686335489601,0.0122431865033005,
-1.39670595880646));
#69302=CARTESIAN_POINT('Ctrl Pts',(-0.23709509445159,0.00714687402652576,
-1.39636007339823));
#69303=CARTESIAN_POINT('Ctrl Pts',(-0.237176706813453,0.00351693476401216,
-1.39611134354054));
#69304=CARTESIAN_POINT('Ctrl Pts',(-0.237170428945466,-0.0096271083778691,
-1.39520165287263));
#69305=CARTESIAN_POINT('Ctrl Pts',(-0.236593455660036,-0.0191308966005396,
-1.39452629322106));
#69306=CARTESIAN_POINT('Ctrl Pts',(-0.233338429146559,-0.0459526329521729,
-1.39257640518096));
#69307=CARTESIAN_POINT('Ctrl Pts',(-0.229311743919245,-0.0630442636455679,
-1.39127764092337));
#69308=CARTESIAN_POINT('Ctrl Pts',(-0.222065781622701,-0.0834001484286103,
-1.38974309070626));
#69309=CARTESIAN_POINT('Ctrl Pts',(-0.220590552924236,-0.0872273410722001,
-1.38945540392021));
#69310=CARTESIAN_POINT('Ctrl Pts',(-0.218554935371255,-0.0921258317882973,
-1.38908993986535));
#69311=CARTESIAN_POINT('Ctrl Pts',(-0.21808469671968,-0.0932335447607527,
-1.38900748196616));
#69312=CARTESIAN_POINT('Ctrl Pts',(-0.217317997457725,-0.0950020684538213,
-1.38887618675399));
#69313=CARTESIAN_POINT('Ctrl Pts',(-0.217026913361217,-0.0956651657722182,
-1.38882703854436));
#69314=CARTESIAN_POINT('Ctrl Pts',(-0.21646116949202,-0.096938073019583,
-1.38873286072264));
#69315=CARTESIAN_POINT('Ctrl Pts',(-0.216186963279736,-0.0975480641393312,
-1.38868780644797));
#69316=CARTESIAN_POINT('Ctrl Pts',(-0.215521331154094,-0.0990122175391209,
-1.38857983181633));
#69317=CARTESIAN_POINT('Ctrl Pts',(-0.215127397500648,-0.0998652408191562,
-1.38851706308935));
#69318=CARTESIAN_POINT('Ctrl Pts',(-0.213740106358193,-0.10282297388671,
-1.38829982491187));
#69319=CARTESIAN_POINT('Ctrl Pts',(-0.212720809829733,-0.104915466418026,
-1.388146849749));
#69320=CARTESIAN_POINT('Ctrl Pts',(-0.210122481711546,-0.110055912561179,
-1.38777199047017));
#69321=CARTESIAN_POINT('Ctrl Pts',(-0.20850773805157,-0.113085308027284,
-1.38755190827367));
#69322=CARTESIAN_POINT('Ctrl Pts',(-0.201221121613751,-0.126068514666707,
-1.38660770909614));
#69323=CARTESIAN_POINT('Ctrl Pts',(-0.194897703930561,-0.135639722797267,
-1.38590853109235));
#69324=CARTESIAN_POINT('Ctrl Pts',(-0.178631829447137,-0.156760043844247,
-1.38427459882961));
#69325=CARTESIAN_POINT('Ctrl Pts',(-0.168221760574742,-0.167882118757019,
-1.38333965131958));
#69326=CARTESIAN_POINT('Ctrl Pts',(-0.154413733032921,-0.180051844099157,
-1.38215052405384));
#69327=CARTESIAN_POINT('Ctrl Pts',(-0.151964900048369,-0.182123406136785,
-1.38194147873121));
#69328=CARTESIAN_POINT('Ctrl Pts',(-0.148311745381434,-0.185088765740522,
-1.3816318269125));
#69329=CARTESIAN_POINT('Ctrl Pts',(-0.147139687643511,-0.186021872822759,
-1.38153280303838));
#69330=CARTESIAN_POINT('Ctrl Pts',(-0.145032621628037,-0.187666993041948,
-1.38135530928337));
#69331=CARTESIAN_POINT('Ctrl Pts',(-0.144101004916162,-0.188383284583807,
-1.381277012559));
#69332=CARTESIAN_POINT('Ctrl Pts',(-0.142133704031066,-0.189872749941943,
-1.38111202676177));
#69333=CARTESIAN_POINT('Ctrl Pts',(-0.141096948940548,-0.190644438358404,
-1.38102528297351));
#69334=CARTESIAN_POINT('Ctrl Pts',(-0.138341766994595,-0.192660419583374,
-1.38079526112967));
#69335=CARTESIAN_POINT('Ctrl Pts',(-0.136612895246199,-0.193890170228473,
-1.38065142923181));
#69336=CARTESIAN_POINT('Ctrl Pts',(-0.128100401593597,-0.199774751356675,
-1.37994548947575));
#69337=CARTESIAN_POINT('Ctrl Pts',(-0.121094958642767,-0.204097151313251,
-1.37937111212416));
#69338=CARTESIAN_POINT('Ctrl Pts',(-0.105352792476685,-0.212714047412349,
-1.37809420760581));
#69339=CARTESIAN_POINT('Ctrl Pts',(-0.0965475001049797,-0.216852552458957,
-1.37738840730181));
#69340=CARTESIAN_POINT('Ctrl Pts',(-0.0741821801217256,-0.225731544944955,
-1.3756318807314));
#69341=CARTESIAN_POINT('Ctrl Pts',(-0.0603967063129183,-0.229804345371231,
-1.37457931256262));
#69342=CARTESIAN_POINT('Ctrl Pts',(-0.0445002670189007,-0.2329703305017,
-1.37344939102814));
#69343=CARTESIAN_POINT('Ctrl Pts',(-0.0426695804121364,-0.233312571661833,
-1.37332052292008));
#69344=CARTESIAN_POINT('Ctrl Pts',(-0.0398705077542063,-0.233801800395719,
-1.37312559123558));
#69345=CARTESIAN_POINT('Ctrl Pts',(-0.0389049751829175,-0.233964403805189,
-1.37305873052469));
#69346=CARTESIAN_POINT('Ctrl Pts',(-0.0372777583448618,-0.234228088245201,
-1.37294672087146));
#69347=CARTESIAN_POINT('Ctrl Pts',(-0.0366166099122925,-0.234332354810391,
-1.37290139682346));
#69348=CARTESIAN_POINT('Ctrl Pts',(-0.0352548714283871,-0.234541204041472,
-1.37280843933128));
#69349=CARTESIAN_POINT('Ctrl Pts',(-0.0345542414362199,-0.234645449103323,
-1.37276082485481));
#69350=CARTESIAN_POINT('Ctrl Pts',(-0.0327330803718395,-0.23490808139759,
-1.37263758835211));
#69351=CARTESIAN_POINT('Ctrl Pts',(-0.0316118478432321,-0.235061592907282,
-1.37256223460363));
#69352=CARTESIAN_POINT('Ctrl Pts',(-0.0266917272786496,-0.235699380569875,
-1.37223367535917));
#69353=CARTESIAN_POINT('Ctrl Pts',(-0.0228822902957143,-0.23609966361483,
-1.3719847727049));
#69354=CARTESIAN_POINT('Ctrl Pts',(-0.0120826331528088,-0.236970578587025,
-1.37129038046716));
#69355=CARTESIAN_POINT('Ctrl Pts',(-0.0050786400173435,-0.2372240861543,
-1.37085324878858));
#69356=CARTESIAN_POINT('Ctrl Pts',(0.0179500283192576,-0.237036998915701,
-1.36943058559849));
#69357=CARTESIAN_POINT('Ctrl Pts',(0.0339182507468475,-0.235283419466258,
-1.36846447640405));
#69358=CARTESIAN_POINT('Ctrl Pts',(0.0564575881648879,-0.230464475200226,
-1.36701384257709));
#69359=CARTESIAN_POINT('Ctrl Pts',(0.0632582589663762,-0.228691302104172,
-1.36656481679112));
#69360=CARTESIAN_POINT('Ctrl Pts',(0.0719704511805524,-0.226001369708364,
-1.36596936728562));
#69361=CARTESIAN_POINT('Ctrl Pts',(0.0739628151600318,-0.225357197498067,
-1.36583180614467));
#69362=CARTESIAN_POINT('Ctrl Pts',(0.0771650071169762,-0.224274825017162,
-1.36560833610127));
#69363=CARTESIAN_POINT('Ctrl Pts',(0.0783802840535355,-0.223853001812999,
-1.3655229680166));
#69364=CARTESIAN_POINT('Ctrl Pts',(0.0807005860550093,-0.223026412877333,
-1.36535887620145));
#69365=CARTESIAN_POINT('Ctrl Pts',(0.0818061507671564,-0.222623267070293,
-1.36528020834205));
#69366=CARTESIAN_POINT('Ctrl Pts',(0.0843474518637464,-0.221675091774994,
-1.3650982412579));
#69367=CARTESIAN_POINT('Ctrl Pts',(0.0857809730416737,-0.221124316663985,
-1.36499475253513));
#69368=CARTESIAN_POINT('Ctrl Pts',(0.0902994010818894,-0.219337735912614,
-1.36466582372755));
#69369=CARTESIAN_POINT('Ctrl Pts',(0.0933636187113242,-0.218051042145838,
-1.36443868788434));
#69370=CARTESIAN_POINT('Ctrl Pts',(0.100496385621436,-0.214878015437962,
-1.36390006384044));
#69371=CARTESIAN_POINT('Ctrl Pts',(0.104540358629836,-0.212939883411607,
-1.36358692633651));
#69372=CARTESIAN_POINT('Ctrl Pts',(0.119731242323108,-0.205122396791407,
-1.36238071825746));
#69373=CARTESIAN_POINT('Ctrl Pts',(0.130457240857722,-0.198473202165949,
-1.36146467590324));
#69374=CARTESIAN_POINT('Ctrl Pts',(0.151176346371205,-0.183221343677735,
-1.35958568862047));
#69375=CARTESIAN_POINT('Ctrl Pts',(0.161085967741501,-0.174572979836453,
-1.35862569667976));
#69376=CARTESIAN_POINT('Ctrl Pts',(0.171666909520577,-0.16366647180175,
-1.35756581343514));
#69377=CARTESIAN_POINT('Ctrl Pts',(0.173084942369714,-0.16216610392902,
-1.35742299629438));
#69378=CARTESIAN_POINT('Ctrl Pts',(0.175046656083968,-0.160035435669459,
-1.35722455929758));
#69379=CARTESIAN_POINT('Ctrl Pts',(0.175606836291864,-0.159420549415688,
-1.35716779310845));
#69380=CARTESIAN_POINT('Ctrl Pts',(0.17661339218452,-0.158303952077766,
-1.35706562971752));
#69381=CARTESIAN_POINT('Ctrl Pts',(0.177060893198148,-0.157803268923824,
-1.35702015007105));
#69382=CARTESIAN_POINT('Ctrl Pts',(0.177973765308479,-0.156773136534114,
-1.35692726452776));
#69383=CARTESIAN_POINT('Ctrl Pts',(0.178438912007092,-0.156243502877947,
-1.35687987490297));
#69384=CARTESIAN_POINT('Ctrl Pts',(0.179634359814534,-0.15487001897758,
-1.35675789997811));
#69385=CARTESIAN_POINT('Ctrl Pts',(0.180361089120951,-0.154023062097295,
-1.35668357275254));
#69386=CARTESIAN_POINT('Ctrl Pts',(0.183458107362167,-0.150361704638763,
-1.35636589381563));
#69387=CARTESIAN_POINT('Ctrl Pts',(0.18576884883244,-0.14749731461147,-1.35612650132637));
#69388=CARTESIAN_POINT('Ctrl Pts',(0.192027494092287,-0.139358565646511,
-1.35546760397506));
#69389=CARTESIAN_POINT('Ctrl Pts',(0.195823875336761,-0.133971604301315,
-1.35505546605861));
#69390=CARTESIAN_POINT('Ctrl Pts',(0.201133990348386,-0.125727703035984,
-1.35444850223891));
#69391=CARTESIAN_POINT('Ctrl Pts',(0.202821461987519,-0.122986960986254,
-1.35425042430521));
#69392=CARTESIAN_POINT('Ctrl Pts',(0.213996540516776,-0.103980859844897,
-1.35289651813524));
#69393=CARTESIAN_POINT('Ctrl Pts',(0.221572491773095,-0.0866722844692302,
-1.3517541149914));
#69394=CARTESIAN_POINT('Ctrl Pts',(0.22789824770484,-0.0657535607218792,
-1.35033997355525));
#69395=CARTESIAN_POINT('Ctrl Pts',(0.228718781702932,-0.0628399522235472,
-1.35014247279239));
#69396=CARTESIAN_POINT('Ctrl Pts',(0.229857201130097,-0.0584793859985416,
-1.34984571138063));
#69397=CARTESIAN_POINT('Ctrl Pts',(0.2302176743965,-0.0570437877981794,
-1.34974782350547));
#69398=CARTESIAN_POINT('Ctrl Pts',(0.230839025646515,-0.0544673681293576,
-1.34957176917375));
#69399=CARTESIAN_POINT('Ctrl Pts',(0.231104944369353,-0.0533278028436546,
-1.34949376765513));
#69400=CARTESIAN_POINT('Ctrl Pts',(0.231652076489912,-0.0509021522962062,
-1.34932743410502));
#69401=CARTESIAN_POINT('Ctrl Pts',(0.231931035687726,-0.0496156045405141,
-1.34923903269144));
#69402=CARTESIAN_POINT('Ctrl Pts',(0.232654094637426,-0.0461414726759075,
-1.34899980147271));
#69403=CARTESIAN_POINT('Ctrl Pts',(0.233078036066404,-0.0439498778300113,
-1.34884833586036));
#69404=CARTESIAN_POINT('Ctrl Pts',(0.23521512146049,-0.0319998117682699,
-1.34801920778947));
#69405=CARTESIAN_POINT('Ctrl Pts',(0.236346216869232,-0.0221485761220135,
-1.34732340164914));
#69406=CARTESIAN_POINT('Ctrl Pts',(0.237385352686255,-0.00206735097595695,
-1.34588188362514));
#69407=CARTESIAN_POINT('Ctrl Pts',(0.237254544561929,0.00814475353624223,
-1.34513676143195));
#69408=CARTESIAN_POINT('Ctrl Pts',(0.236307634784926,0.0203697165068839,
-1.34424135858273));
#69409=CARTESIAN_POINT('Ctrl Pts',(0.23612181286623,0.0224212662869678,
-1.34409100529598));
#69410=CARTESIAN_POINT('Ctrl Pts',(0.234797871217047,0.0351849887777631,
-1.34315573282199));
#69411=CARTESIAN_POINT('Ctrl Pts',(0.232957608875962,0.0458130032771233,
-1.34237703706866));
#69412=CARTESIAN_POINT('Ctrl Pts',(0.230079265180973,0.0575964266217463,
-1.34153743714864));
#69413=CARTESIAN_POINT('Ctrl Pts',(0.229746450762631,0.0589099753947206,
-1.34144419070656));
#69414=CARTESIAN_POINT('Ctrl Pts',(0.229189630387646,0.0610311074394687,
-1.34129425723242));
#69415=CARTESIAN_POINT('Ctrl Pts',(0.228972575422344,0.0618404601477494,
-1.34123719966252));
#69416=CARTESIAN_POINT('Ctrl Pts',(0.228577999236883,0.0632811898750169,
-1.34113592353936));
#69417=CARTESIAN_POINT('Ctrl Pts',(0.22840214422485,0.063912997703503,-1.34109161242942));
#69418=CARTESIAN_POINT('Ctrl Pts',(0.228011219893008,0.0652952803985223,
-1.34099489265104));
#69419=CARTESIAN_POINT('Ctrl Pts',(0.227795064856602,0.0660454276271205,
-1.34094254711387));
#69420=CARTESIAN_POINT('Ctrl Pts',(0.227162888951108,0.0681993107448984,
-1.34079262361014));
#69421=CARTESIAN_POINT('Ctrl Pts',(0.226737560230538,0.0696003099903044,
-1.34069556504387));
#69422=CARTESIAN_POINT('Ctrl Pts',(0.223223889427796,0.0807999031382693,
-1.33992269814227));
#69423=CARTESIAN_POINT('Ctrl Pts',(0.219514397376743,0.0903936637310679,
-1.33927903149315));
#69424=CARTESIAN_POINT('Ctrl Pts',(0.208410349768753,0.114356542456391,
-1.33764771829156));
#69425=CARTESIAN_POINT('Ctrl Pts',(0.200151198567343,0.128264500313431,
-1.33667499509042));
#69426=CARTESIAN_POINT('Ctrl Pts',(0.186436603748621,0.146768389193457,
-1.33522438379733));
#69427=CARTESIAN_POINT('Ctrl Pts',(0.182089506981463,0.152128119778144,
-1.33478321621127));
#69428=CARTESIAN_POINT('Ctrl Pts',(0.176136271622478,0.158846840050143,
-1.33419689484953));
#69429=CARTESIAN_POINT('Ctrl Pts',(0.174736838051403,0.160384979812369,
-1.33406026392175));
#69430=CARTESIAN_POINT('Ctrl Pts',(0.172441387726069,0.162842240247576,
-1.33383793601572));
#69431=CARTESIAN_POINT('Ctrl Pts',(0.171557797697396,0.163772859011835,
-1.33375276960803));
#69432=CARTESIAN_POINT('Ctrl Pts',(0.169848915416609,0.165543690646399,
-1.33358881521645));
#69433=CARTESIAN_POINT('Ctrl Pts',(0.169024829627993,0.166385018748336,
-1.33351008108543));
#69434=CARTESIAN_POINT('Ctrl Pts',(0.167107085451819,0.168313937291127,
-1.33332759238982));
#69435=CARTESIAN_POINT('Ctrl Pts',(0.166009025680677,0.169397056324437,
-1.33322364470926));
#69436=CARTESIAN_POINT('Ctrl Pts',(0.162485511194223,0.172805465234497,
-1.33289173735513));
#69437=CARTESIAN_POINT('Ctrl Pts',(0.160021265152094,0.175089870768702,
-1.33266203808378));
#69438=CARTESIAN_POINT('Ctrl Pts',(0.154108437845492,0.180342072950492,
-1.33211621187048));
#69439=CARTESIAN_POINT('Ctrl Pts',(0.150621441701078,0.183264427782036,
-1.33179837493704));
#69440=CARTESIAN_POINT('Ctrl Pts',(0.12926598355019,0.200140515028974,-1.32987557459896));
#69441=CARTESIAN_POINT('Ctrl Pts',(0.109559503383775,0.211571239441693,
-1.32818217708357));
#69442=CARTESIAN_POINT('Ctrl Pts',(0.0844684286795744,0.221667002692134,
-1.32625765233554));
#69443=CARTESIAN_POINT('Ctrl Pts',(0.0803590516932933,0.223189615035733,
-1.32594979805719));
#69444=CARTESIAN_POINT('Ctrl Pts',(0.0750443276835538,0.22499298560114,
-1.32556295431464));
#69445=CARTESIAN_POINT('Ctrl Pts',(0.0738760162098553,0.225379300470429,
-1.32547860663166));
#69446=CARTESIAN_POINT('Ctrl Pts',(0.0720097249742363,0.225980338190002,
-1.32534502295089));
#69447=CARTESIAN_POINT('Ctrl Pts',(0.0713136883165767,0.226200954097564,
-1.32529545736386));
#69448=CARTESIAN_POINT('Ctrl Pts',(0.0699805046981877,0.226616754913183,
-1.32520102101074));
#69449=CARTESIAN_POINT('Ctrl Pts',(0.0693435447264682,0.226812472012421,
-1.32515612155123));
#69450=CARTESIAN_POINT('Ctrl Pts',(0.0678204103913752,0.227273465690268,
-1.32504926427574));
#69451=CARTESIAN_POINT('Ctrl Pts',(0.0669334819703331,0.227536250596239,
-1.32498744990321));
#69452=CARTESIAN_POINT('Ctrl Pts',(0.0638962244466875,0.228416852680628,
-1.32477709224167));
#69453=CARTESIAN_POINT('Ctrl Pts',(0.0617386241588662,0.229009452362055,
-1.32462991967725));
#69454=CARTESIAN_POINT('Ctrl Pts',(0.0564222575080445,0.230389028030097,
-1.32427207538616));
#69455=CARTESIAN_POINT('Ctrl Pts',(0.0532549881082419,0.231141696375161,
-1.32406300078719));
#69456=CARTESIAN_POINT('Ctrl Pts',(0.0399171142029785,0.234022562892254,
-1.32319588936015));
#69457=CARTESIAN_POINT('Ctrl Pts',(0.0296271888497427,0.235546595181886,
-1.32255883153795));
#69458=CARTESIAN_POINT('Ctrl Pts',(0.00270132566876937,0.237741502872241,
-1.32090298004351));
#69459=CARTESIAN_POINT('Ctrl Pts',(-0.0139611691113274,0.23734641893675,
-1.31988604334673));
#69460=CARTESIAN_POINT('Ctrl Pts',(-0.033591505261568,0.234805579509177,
-1.31860683335724));
#69461=CARTESIAN_POINT('Ctrl Pts',(-0.0367297670179699,0.234335170332696,
-1.31839997276463));
#69462=CARTESIAN_POINT('Ctrl Pts',(-0.0405519932500514,0.233683574011484,
-1.31814477381336));
#69463=CARTESIAN_POINT('Ctrl Pts',(-0.0412459145842788,0.23356209328554,
-1.31809831128101));
#69464=CARTESIAN_POINT('Ctrl Pts',(-0.0419392741369039,0.233437524639612,
-1.31805175208418));
#69465=CARTESIAN_POINT('Origin',(0.,0.,-2.1456589891905));
#69466=CARTESIAN_POINT('',(-0.0419392699415209,0.233437525393353,-1.19828290886153));
#69467=CARTESIAN_POINT('',(-0.041939274136423,0.233437524639699,-1.21783461098805));
#69468=CARTESIAN_POINT('',(-0.0419392741328076,0.233437524640348,-2.1456589891905));
#69469=CARTESIAN_POINT('',(-0.23717491446692,0.000201426436582323,-1.27600110192935));
#69470=CARTESIAN_POINT('Ctrl Pts',(-0.0419392699415209,0.233437525393353,
-1.19828290886153));
#69471=CARTESIAN_POINT('Ctrl Pts',(-0.0375335716888505,0.234229050954585,
-1.198602388006));
#69472=CARTESIAN_POINT('Ctrl Pts',(-0.033105142309298,0.234895910556959,
-1.19891811259145));
#69473=CARTESIAN_POINT('Ctrl Pts',(-0.0273288220524848,0.235599050176692,
-1.1993207924431));
#69474=CARTESIAN_POINT('Ctrl Pts',(-0.0259969815930074,0.235749727706377,
-1.199413009077));
#69475=CARTESIAN_POINT('Ctrl Pts',(-0.0238347252023007,0.235975807113033,
-1.19956162851533));
#69476=CARTESIAN_POINT('Ctrl Pts',(-0.0230050853663194,0.23605813218132,
-1.19961839155736));
#69477=CARTESIAN_POINT('Ctrl Pts',(-0.0215221072182611,0.236197395351657,
-1.19971936871144));
#69478=CARTESIAN_POINT('Ctrl Pts',(-0.0208689508174868,0.23625600012612,
-1.19976367287095));
#69479=CARTESIAN_POINT('Ctrl Pts',(-0.0194338546162219,0.236378766840449,
-1.19986064273661));
#69480=CARTESIAN_POINT('Ctrl Pts',(-0.0186518346691687,0.236441758634999,
-1.19991324313493));
#69481=CARTESIAN_POINT('Ctrl Pts',(-0.0163919179361852,0.236612513133608,
-1.20006459190996));
#69482=CARTESIAN_POINT('Ctrl Pts',(-0.0149132730379966,0.236710310103008,
-1.20016280565689));
#69483=CARTESIAN_POINT('Ctrl Pts',(-0.00222524823829375,0.237430124516555,
-1.20099934766508));
#69484=CARTESIAN_POINT('Ctrl Pts',(0.00901590548175787,0.237269464910186,
-1.20169925092852));
#69485=CARTESIAN_POINT('Ctrl Pts',(0.0387686965193935,0.234725603632027,
-1.20353873484218));
#69486=CARTESIAN_POINT('Ctrl Pts',(0.0570793929326259,0.230956743988287,
-1.20466237556514));
#69487=CARTESIAN_POINT('Ctrl Pts',(0.0787267563728954,0.223766728035313,
-1.20612397067814));
#69488=CARTESIAN_POINT('Ctrl Pts',(0.0826576774958468,0.222344677630813,
-1.206394736598));
#69489=CARTESIAN_POINT('Ctrl Pts',(0.0881554191161044,0.220189873714043,
-1.2067821181835));
#69490=CARTESIAN_POINT('Ctrl Pts',(0.0897550892326629,0.219542665785454,
-1.2068958907564));
#69491=CARTESIAN_POINT('Ctrl Pts',(0.092351989574049,0.218458864188389,
-1.20708238603676));
#69492=CARTESIAN_POINT('Ctrl Pts',(0.0933535468765892,0.218032751069364,
-1.20715475277753));
#69493=CARTESIAN_POINT('Ctrl Pts',(0.0954556219844288,0.217121282961472,
-1.20730758471329));
#69494=CARTESIAN_POINT('Ctrl Pts',(0.0965554486869348,0.216634421364518,
-1.20738809961092));
#69495=CARTESIAN_POINT('Ctrl Pts',(0.099192734216556,0.215442898124175,
-1.20758252374353));
#69496=CARTESIAN_POINT('Ctrl Pts',(0.100726433123141,0.214730124308128,
-1.2076967089646));
#69497=CARTESIAN_POINT('Ctrl Pts',(0.106091992143453,0.212166393656812,
-1.20810021416272));
#69498=CARTESIAN_POINT('Ctrl Pts',(0.109881337151372,0.210228868317865,
-1.20839250436415));
#69499=CARTESIAN_POINT('Ctrl Pts',(0.119098303118215,0.205198872537217,
-1.20912220733912));
#69500=CARTESIAN_POINT('Ctrl Pts',(0.124459553273245,0.201992057558137,
-1.20956331990691));
#69501=CARTESIAN_POINT('Ctrl Pts',(0.138566333363702,0.192779162508644,
-1.21076875221957));
#69502=CARTESIAN_POINT('Ctrl Pts',(0.14704558181697,0.186392067274509,-1.21154287397845));
#69503=CARTESIAN_POINT('Ctrl Pts',(0.164151871164029,0.171610771149758,
-1.21319388934757));
#69504=CARTESIAN_POINT('Ctrl Pts',(0.172627208081991,0.163082795514992,
-1.21406862173344));
#69505=CARTESIAN_POINT('Ctrl Pts',(0.181772243374075,0.152365239229572,
-1.21505150918695));
#69506=CARTESIAN_POINT('Ctrl Pts',(0.18310268747856,0.150763792618592,-1.21519556270663));
#69507=CARTESIAN_POINT('Ctrl Pts',(0.184936967490161,0.148495777033672,
-1.21539543456646));
#69508=CARTESIAN_POINT('Ctrl Pts',(0.185458585696061,0.147843805368463,
-1.21545242012444));
#69509=CARTESIAN_POINT('Ctrl Pts',(0.186394107378123,0.146661752388024,
-1.21555487112382));
#69510=CARTESIAN_POINT('Ctrl Pts',(0.186809219041781,0.146132640433667,
-1.21560042032738));
#69511=CARTESIAN_POINT('Ctrl Pts',(0.18765427416922,0.145046025926246,-1.21569331831912));
#69512=CARTESIAN_POINT('Ctrl Pts',(0.188083994851933,0.144488363422198,
-1.21574065171482));
#69513=CARTESIAN_POINT('Ctrl Pts',(0.18918561232246,0.143045516074784,-1.21586226105625));
#69514=CARTESIAN_POINT('Ctrl Pts',(0.189853791831849,0.142157495149407,
-1.21593628201826));
#69515=CARTESIAN_POINT('Ctrl Pts',(0.192679999325499,0.138345951144541,
-1.21625064542326));
#69516=CARTESIAN_POINT('Ctrl Pts',(0.194777058866314,0.135377565306569,
-1.21648713100904));
#69517=CARTESIAN_POINT('Ctrl Pts',(0.200411454103742,0.126999944798079,
-1.21713533541856));
#69518=CARTESIAN_POINT('Ctrl Pts',(0.203797327226507,0.121492379964609,
-1.21753997385796));
#69519=CARTESIAN_POINT('Ctrl Pts',(0.209111452476666,0.111999484198508,
-1.21821377993903));
#69520=CARTESIAN_POINT('Ctrl Pts',(0.211160658382324,0.108086362965915,
-1.21848512385362));
#69521=CARTESIAN_POINT('Ctrl Pts',(0.220850817074418,0.0882534555678281,
-1.21983893035908));
#69522=CARTESIAN_POINT('Ctrl Pts',(0.226805497127547,0.071574697556417,
-1.22091486815826));
#69523=CARTESIAN_POINT('Ctrl Pts',(0.231570621596853,0.0513496594690051,
-1.22225828064958));
#69524=CARTESIAN_POINT('Ctrl Pts',(0.232226870004729,0.0482951309811835,
-1.22246200318195));
#69525=CARTESIAN_POINT('Ctrl Pts',(0.23310843446395,0.0437571195147533,
-1.22276631444747));
#69526=CARTESIAN_POINT('Ctrl Pts',(0.233380333225057,0.0422829471140898,
-1.2228654241886));
#69527=CARTESIAN_POINT('Ctrl Pts',(0.233839973352956,0.0396512592634784,
-1.22304285243333));
#69528=CARTESIAN_POINT('Ctrl Pts',(0.234033140820919,0.0384947322581955,
-1.2231209959828));
#69529=CARTESIAN_POINT('Ctrl Pts',(0.234423333912465,0.0360470119439916,
-1.22328676447424));
#69530=CARTESIAN_POINT('Ctrl Pts',(0.234618284463202,0.0347555323619409,
-1.22337445235446));
#69531=CARTESIAN_POINT('Ctrl Pts',(0.235110584483999,0.0313011222896039,
-1.22360962838645));
#69532=CARTESIAN_POINT('Ctrl Pts',(0.235388745978136,0.0291356294528762,
-1.22375771536972));
#69533=CARTESIAN_POINT('Ctrl Pts',(0.236671314626061,0.0179284385121385,
-1.22452774614878));
#69534=CARTESIAN_POINT('Ctrl Pts',(0.237184672265297,0.00883934162330922,
-1.22516485220924));
#69535=CARTESIAN_POINT('Ctrl Pts',(0.23716317265967,-0.0110931547559999,
-1.22658884910768));
#69536=CARTESIAN_POINT('Ctrl Pts',(0.236408704781146,-0.0219162313744683,
-1.22737964729629));
#69537=CARTESIAN_POINT('Ctrl Pts',(0.233243498756143,-0.0446906506752908,
-1.22905888857587));
#69538=CARTESIAN_POINT('Ctrl Pts',(0.230646363080531,-0.0565870840435355,
-1.2299451411992));
#69539=CARTESIAN_POINT('Ctrl Pts',(0.226552130538029,-0.0702168360177963,
-1.23093785208365));
#69540=CARTESIAN_POINT('Ctrl Pts',(0.225930175862904,-0.0721929932594657,
-1.23108118188371));
#69541=CARTESIAN_POINT('Ctrl Pts',(0.225021859586135,-0.0749522349768024,
-1.23128022060694));
#69542=CARTESIAN_POINT('Ctrl Pts',(0.22475716305234,-0.0757422770246938,
-1.23133708444167));
#69543=CARTESIAN_POINT('Ctrl Pts',(0.224271454412186,-0.077167007120609,
-1.23143938159245));
#69544=CARTESIAN_POINT('Ctrl Pts',(0.224051897942451,-0.0778021806965472,
-1.23148489790129));
#69545=CARTESIAN_POINT('Ctrl Pts',(0.223596589534452,-0.0791014687970383,
-1.23157780822877));
#69546=CARTESIAN_POINT('Ctrl Pts',(0.223360572993072,-0.0797654792657574,
-1.23162518630813));
#69547=CARTESIAN_POINT('Ctrl Pts',(0.222743688972042,-0.0814768160695972,
-1.23174704688657));
#69548=CARTESIAN_POINT('Ctrl Pts',(0.222358387838322,-0.0825225424583822,
-1.23182127238899));
#69549=CARTESIAN_POINT('Ctrl Pts',(0.220675204369397,-0.0869933929168607,
-1.23213774736747));
#69550=CARTESIAN_POINT('Ctrl Pts',(0.219305368477771,-0.0903911233521313,
-1.2323760754072));
#69551=CARTESIAN_POINT('Ctrl Pts',(0.215271781032465,-0.0997638206390286,
-1.2330310195956));
#69552=CARTESIAN_POINT('Ctrl Pts',(0.212438670425472,-0.105662591894336,
-1.23344037618754));
#69553=CARTESIAN_POINT('Ctrl Pts',(0.207565674377541,-0.114817851775556,
-1.23408247598968));
#69554=CARTESIAN_POINT('Ctrl Pts',(0.205684564094864,-0.118154599439263,
-1.23431797982359));
#69555=CARTESIAN_POINT('Ctrl Pts',(0.194409279385959,-0.137068935582851,
-1.2356691781174));
#69556=CARTESIAN_POINT('Ctrl Pts',(0.183329837601139,-0.151568289716536,
-1.23677538157028));
#69557=CARTESIAN_POINT('Ctrl Pts',(0.168560572967574,-0.166879707730256,
-1.23815124522914));
#69558=CARTESIAN_POINT('Ctrl Pts',(0.166375106479975,-0.169058646987889,
-1.23835253008245));
#69559=CARTESIAN_POINT('Ctrl Pts',(0.163071042917213,-0.17222671408156,
-1.23865389315342));
#69560=CARTESIAN_POINT('Ctrl Pts',(0.161984560066371,-0.173248977516235,
-1.23875253452157));
#69561=CARTESIAN_POINT('Ctrl Pts',(0.160027601322428,-0.175055763783461,
-1.23892944317364));
#69562=CARTESIAN_POINT('Ctrl Pts',(0.159160811215797,-0.175844219999847,
-1.23900753940827));
#69563=CARTESIAN_POINT('Ctrl Pts',(0.157312469455246,-0.177500660132121,
-1.23917354399123));
#69564=CARTESIAN_POINT('Ctrl Pts',(0.156329499418021,-0.178366994944431,
-1.23926151778802));
#69565=CARTESIAN_POINT('Ctrl Pts',(0.153675191617895,-0.180667557593463,
-1.23949828294124));
#69566=CARTESIAN_POINT('Ctrl Pts',(0.151991005567457,-0.182086695124216,
-1.23964768738499));
#69567=CARTESIAN_POINT('Ctrl Pts',(0.143017698628761,-0.189436590708973,
-1.24043964756818));
#69568=CARTESIAN_POINT('Ctrl Pts',(0.135401559154596,-0.194952970771413,
-1.24109843569143));
#69569=CARTESIAN_POINT('Ctrl Pts',(0.118517889648167,-0.205714414925099,
-1.24253068438605));
#69570=CARTESIAN_POINT('Ctrl Pts',(0.109183376990809,-0.210817153469351,
-1.2433064161843));
#69571=CARTESIAN_POINT('Ctrl Pts',(0.0886256387895476,-0.220322580180069,
-1.24496044281448));
#69572=CARTESIAN_POINT('Ctrl Pts',(0.0773433116924118,-0.224531986851791,
-1.24583657246531));
#69573=CARTESIAN_POINT('Ctrl Pts',(0.0637935348351434,-0.228444043699048,
-1.24682040732057));
#69574=CARTESIAN_POINT('Ctrl Pts',(0.0617900912740089,-0.228994064429848,
-1.24696414925404));
#69575=CARTESIAN_POINT('Ctrl Pts',(0.0589723462046585,-0.229727967098623,
-1.2471636624892));
#69576=CARTESIAN_POINT('Ctrl Pts',(0.0581639773478486,-0.229933965033463,
-1.24722059570296));
#69577=CARTESIAN_POINT('Ctrl Pts',(0.0567021794328324,-0.230298274974983,
-1.24732298052519));
#69578=CARTESIAN_POINT('Ctrl Pts',(0.0560491333760602,-0.230458081431589,
-1.247368515565));
#69579=CARTESIAN_POINT('Ctrl Pts',(0.0547105801916713,-0.230779611491156,
-1.24746141877361));
#69580=CARTESIAN_POINT('Ctrl Pts',(0.0540250183372702,-0.23094106194336,
-1.24750877131527));
#69581=CARTESIAN_POINT('Ctrl Pts',(0.0522546133921074,-0.231349678920033,
-1.24763048832594));
#69582=CARTESIAN_POINT('Ctrl Pts',(0.0511687167463624,-0.231592273414444,
-1.24770459694924));
#69583=CARTESIAN_POINT('Ctrl Pts',(0.0465172289896875,-0.232597124113077,
-1.24801986346981));
#69584=CARTESIAN_POINT('Ctrl Pts',(0.04293581155542,-0.233284792408089,
-1.2482571369598));
#69585=CARTESIAN_POINT('Ctrl Pts',(0.0329342313703243,-0.234967036408672,
-1.24890821912993));
#69586=CARTESIAN_POINT('Ctrl Pts',(0.0264866970737981,-0.235780912877295,
-1.24931487121684));
#69587=CARTESIAN_POINT('Ctrl Pts',(0.00687954081525848,-0.237441338683237,
-1.25053339237953));
#69588=CARTESIAN_POINT('Ctrl Pts',(-0.00632420959262735,-0.237456796389125,
-1.25133061006629));
#69589=CARTESIAN_POINT('Ctrl Pts',(-0.0295998977389296,-0.23554048620596,
-1.25277999032555));
#69590=CARTESIAN_POINT('Ctrl Pts',(-0.0396734207663531,-0.234054387118378,
-1.25342192307541));
#69591=CARTESIAN_POINT('Ctrl Pts',(-0.0518601175622236,-0.23144709601843,
-1.25423380177062));
#69592=CARTESIAN_POINT('Ctrl Pts',(-0.0540934470559132,-0.230935333877508,
-1.25438403453708));
#69593=CARTESIAN_POINT('Ctrl Pts',(-0.0576231802799222,-0.230072493752527,
-1.25462394377638));
#69594=CARTESIAN_POINT('Ctrl Pts',(-0.0589246567527828,-0.229742612477567,
-1.25471293883549));
#69595=CARTESIAN_POINT('Ctrl Pts',(-0.0613523491467177,-0.229105287215435,
-1.25487998184532));
#69596=CARTESIAN_POINT('Ctrl Pts',(-0.0624792368081042,-0.228800542525143,
-1.25495794031191));
#69597=CARTESIAN_POINT('Ctrl Pts',(-0.0649935405305061,-0.228100638576624,
-1.25513284451306));
#69598=CARTESIAN_POINT('Ctrl Pts',(-0.0663796835255853,-0.227701117882089,
-1.25522992950839));
#69599=CARTESIAN_POINT('Ctrl Pts',(-0.0704775831593784,-0.226479403771714,
-1.25551895219583));
#69600=CARTESIAN_POINT('Ctrl Pts',(-0.0731782623176248,-0.225621255141515,
-1.25571205269697));
#69601=CARTESIAN_POINT('Ctrl Pts',(-0.0854993628401374,-0.221461703704126,
-1.256605488278));
#69602=CARTESIAN_POINT('Ctrl Pts',(-0.0949153568900448,-0.217592399978162,
-1.25732414063531));
#69603=CARTESIAN_POINT('Ctrl Pts',(-0.112525807015649,-0.208994793021325,
-1.25873543197637));
#69604=CARTESIAN_POINT('Ctrl Pts',(-0.120744111772503,-0.204356856942591,
-1.25942482440171));
#69605=CARTESIAN_POINT('Ctrl Pts',(-0.138211384784208,-0.193077068790269,
-1.26094278702197));
#69606=CARTESIAN_POINT('Ctrl Pts',(-0.147304152967612,-0.186232866438805,
-1.2617691230051));
#69607=CARTESIAN_POINT('Ctrl Pts',(-0.157431156384765,-0.177402626885747,
-1.26270633061598));
#69608=CARTESIAN_POINT('Ctrl Pts',(-0.158972736150481,-0.176022529564649,
-1.26284947525539));
#69609=CARTESIAN_POINT('Ctrl Pts',(-0.161109231262601,-0.174058868412775,
-1.26304830073329));
#69610=CARTESIAN_POINT('Ctrl Pts',(-0.16171937944521,-0.173492122113766,
-1.26310513334465));
#69611=CARTESIAN_POINT('Ctrl Pts',(-0.162816427076907,-0.172462294910592,
-1.26320739105558));
#69612=CARTESIAN_POINT('Ctrl Pts',(-0.16330436681252,-0.172000336954926,
-1.26325289895056));
#69613=CARTESIAN_POINT('Ctrl Pts',(-0.164300144224293,-0.171049525211686,
-1.2633458125583));
#69614=CARTESIAN_POINT('Ctrl Pts',(-0.164807776125104,-0.170560471472699,
-1.26339320219093));
#69615=CARTESIAN_POINT('Ctrl Pts',(-0.166061136652461,-0.169342160739758,
-1.26351029119111));
#69616=CARTESIAN_POINT('Ctrl Pts',(-0.166804258197174,-0.168610225247599,
-1.26357978669083));
#69617=CARTESIAN_POINT('Ctrl Pts',(-0.169842567043281,-0.165577904399008,
-1.2638643523494));
#69618=CARTESIAN_POINT('Ctrl Pts',(-0.17209531239819,-0.163235247481622,
-1.26407635958309));
#69619=CARTESIAN_POINT('Ctrl Pts',(-0.178046145200246,-0.156786716397018,
-1.26464167672656));
#69620=CARTESIAN_POINT('Ctrl Pts',(-0.181650208091099,-0.152596574309805,
-1.26498984948423));
#69621=CARTESIAN_POINT('Ctrl Pts',(-0.192170894356137,-0.1394634735735,
-1.26603783972241));
#69622=CARTESIAN_POINT('Ctrl Pts',(-0.198597626473805,-0.130148810332736,
-1.26672393660317));
#69623=CARTESIAN_POINT('Ctrl Pts',(-0.211088406002638,-0.108952149726945,
-1.26823749611137));
#69624=CARTESIAN_POINT('Ctrl Pts',(-0.216864221891957,-0.0969470252752098,
-1.26906651398851));
#69625=CARTESIAN_POINT('Ctrl Pts',(-0.222456474065697,-0.0822850555721773,
-1.27008769915586));
#69626=CARTESIAN_POINT('Ctrl Pts',(-0.22327577558371,-0.0800352458470144,
-1.27024456687028));
#69627=CARTESIAN_POINT('Ctrl Pts',(-0.224508736693512,-0.0764831570705249,
-1.27049269320788));
#69628=CARTESIAN_POINT('Ctrl Pts',(-0.224945457692375,-0.0751890091612959,
-1.27058318796867));
#69629=CARTESIAN_POINT('Ctrl Pts',(-0.22573071461815,-0.0727939451664079,
-1.27075087250793));
#69630=CARTESIAN_POINT('Ctrl Pts',(-0.226082437064376,-0.0716941109488004,
-1.27082795459784));
#69631=CARTESIAN_POINT('Ctrl Pts',(-0.226845376240919,-0.0692469510009841,
-1.27099966276104));
#69632=CARTESIAN_POINT('Ctrl Pts',(-0.227252646192095,-0.0678984506049609,
-1.27109441490519));
#69633=CARTESIAN_POINT('Ctrl Pts',(-0.228395959125987,-0.0639873051448738,
-1.27136965688094));
#69634=CARTESIAN_POINT('Ctrl Pts',(-0.229100812321567,-0.0614158460565036,
-1.27155114879985));
#69635=CARTESIAN_POINT('Ctrl Pts',(-0.230599005450093,-0.0555649249063948,
-1.27196545181937));
#69636=CARTESIAN_POINT('Ctrl Pts',(-0.231366002077995,-0.0522793772816916,
-1.27219905356402));
#69637=CARTESIAN_POINT('Ctrl Pts',(-0.235476150772003,-0.0328053735575508,
-1.27358951773686));
#69638=CARTESIAN_POINT('Ctrl Pts',(-0.23718894756512,-0.0163222182344524,
-1.27479481870023));
#69639=CARTESIAN_POINT('Ctrl Pts',(-0.23717491446692,0.000201426436582323,
-1.27600110192935));
#69640=CARTESIAN_POINT('Ctrl Pts',(-0.237174914325959,0.000201592345835819,
-1.2760011140413));
#69641=CARTESIAN_POINT('Ctrl Pts',(-0.237164711325221,0.0122054996164438,
-1.27687744077041));
#69642=CARTESIAN_POINT('Ctrl Pts',(-0.236243205108348,0.0241930379328251,
-1.2777500309929));
#69643=CARTESIAN_POINT('Ctrl Pts',(-0.234237295365433,0.037232730661517,
-1.27866541082618));
#69644=CARTESIAN_POINT('Ctrl Pts',(-0.234048209895879,0.0384034159463861,
-1.27874728070692));
#69645=CARTESIAN_POINT('Ctrl Pts',(-0.233720671664886,0.0403389675235547,
-1.27888207023377));
#69646=CARTESIAN_POINT('Ctrl Pts',(-0.233587227708098,0.0411046439954152,
-1.27893524295015));
#69647=CARTESIAN_POINT('Ctrl Pts',(-0.23333984698255,0.0424839489625012,
-1.27903074546642));
#69648=CARTESIAN_POINT('Ctrl Pts',(-0.233227248121317,0.0430978058118354,
-1.27907314705763));
#69649=CARTESIAN_POINT('Ctrl Pts',(-0.23299135169158,0.044355843035674,
-1.27915982637008));
#69650=CARTESIAN_POINT('Ctrl Pts',(-0.232867806255701,0.0449999511598508,
-1.27920408612858));
#69651=CARTESIAN_POINT('Ctrl Pts',(-0.232580899645795,0.046462919709769,
-1.27930434746129));
#69652=CARTESIAN_POINT('Ctrl Pts',(-0.2324158850276,0.0472814364017038,
-1.27936025490184));
#69653=CARTESIAN_POINT('Ctrl Pts',(-0.231973877075751,0.0494156730779478,
-1.27950558048546));
#69654=CARTESIAN_POINT('Ctrl Pts',(-0.231690007676864,0.0507299609639537,
-1.27959462625443));
#69655=CARTESIAN_POINT('Ctrl Pts',(-0.229285134333641,0.0614228190819688,
-1.28031596780371));
#69656=CARTESIAN_POINT('Ctrl Pts',(-0.226606491376217,0.0706681017237945,
-1.28092019026395));
#69657=CARTESIAN_POINT('Ctrl Pts',(-0.2197396681336,0.0899072699785791,
-1.28218447014225));
#69658=CARTESIAN_POINT('Ctrl Pts',(-0.215414026783435,0.0998280690438886,
-1.28284094821804));
#69659=CARTESIAN_POINT('Ctrl Pts',(-0.205278457628415,0.119320003481633,
-1.28419575650169));
#69660=CARTESIAN_POINT('Ctrl Pts',(-0.199438498708143,0.128843898637117,
-1.28489320437353));
#69661=CARTESIAN_POINT('Ctrl Pts',(-0.191229478648633,0.140328275660303,
-1.28580649322059));
#69662=CARTESIAN_POINT('Ctrl Pts',(-0.189463721957386,0.142703311984585,
-1.2859995224078));
#69663=CARTESIAN_POINT('Ctrl Pts',(-0.186727391371704,0.146243488590924,
-1.28629398268726));
#69664=CARTESIAN_POINT('Ctrl Pts',(-0.185789282195805,0.14743343950999,
-1.28639414273404));
#69665=CARTESIAN_POINT('Ctrl Pts',(-0.184103926614648,0.149529609829552,
-1.28657274471922));
#69666=CARTESIAN_POINT('Ctrl Pts',(-0.183361222864139,0.150439429257537,
-1.28665100293165));
#69667=CARTESIAN_POINT('Ctrl Pts',(-0.181783978282007,0.152342537969004,
-1.28681628383399));
#69668=CARTESIAN_POINT('Ctrl Pts',(-0.180947986126268,0.153334568299571,
-1.28690336404868));
#69669=CARTESIAN_POINT('Ctrl Pts',(-0.178709723529789,0.155946807167504,
-1.28713516627107));
#69670=CARTESIAN_POINT('Ctrl Pts',(-0.177293590594479,0.157554924258461,
-1.28728045729717));
#69671=CARTESIAN_POINT('Ctrl Pts',(-0.170869325001078,0.164653828080447,
-1.2879337325548));
#69672=CARTESIAN_POINT('Ctrl Pts',(-0.165627045253658,0.169926073398702,
-1.2884515267302));
#69673=CARTESIAN_POINT('Ctrl Pts',(-0.1467069323037,0.18724592294889,-1.29027063376794));
#69674=CARTESIAN_POINT('Ctrl Pts',(-0.131895116773179,0.197958337777178,
-1.29161756148034));
#69675=CARTESIAN_POINT('Ctrl Pts',(-0.111488680257177,0.209401721877813,
-1.2933093239065));
#69676=CARTESIAN_POINT('Ctrl Pts',(-0.106889022700937,0.211786568850279,
-1.29368053776999));
#69677=CARTESIAN_POINT('Ctrl Pts',(-0.0994022702734951,0.215362213773916,
-1.29426501866394));
#69678=CARTESIAN_POINT('Ctrl Pts',(-0.0965634841762156,0.216649925701232,
-1.29448224201419));
#69679=CARTESIAN_POINT('Ctrl Pts',(-0.0927842382502456,0.218275191950834,
-1.29476491903108));
#69680=CARTESIAN_POINT('Ctrl Pts',(-0.0918660066237008,0.218663236975568,
-1.29483309981837));
#69681=CARTESIAN_POINT('Ctrl Pts',(-0.0902943486979534,0.219315772471328,
-1.29494891378608));
#69682=CARTESIAN_POINT('Ctrl Pts',(-0.0896421493947211,0.219583156336118,
-1.29499671515367));
#69683=CARTESIAN_POINT('Ctrl Pts',(-0.0883659215240853,0.220099741073461,
-1.2950897354139));
#69684=CARTESIAN_POINT('Ctrl Pts',(-0.0877420124376722,0.220349203261255,
-1.29513496880239));
#69685=CARTESIAN_POINT('Ctrl Pts',(-0.0863425109168294,0.220901889754347,
-1.29523591061485));
#69686=CARTESIAN_POINT('Ctrl Pts',(-0.0855663567175502,0.221203690607967,
-1.29529153497173));
#69687=CARTESIAN_POINT('Ctrl Pts',(-0.0828563669927195,0.222241048706764,
-1.29548456233221));
#69688=CARTESIAN_POINT('Ctrl Pts',(-0.0809144429371287,0.222955410160999,
-1.29562078093307));
#69689=CARTESIAN_POINT('Ctrl Pts',(-0.0674903770669402,0.227695119963206,
-1.29654967589162));
#69690=CARTESIAN_POINT('Ctrl Pts',(-0.0557211499386474,0.230857637130987,
-1.29730081186011));
#69691=CARTESIAN_POINT('Ctrl Pts',(-0.0431533968831323,0.233216949903831,
-1.29808568538759));
#69692=CARTESIAN_POINT('Ctrl Pts',(-0.0425465299387445,0.233328425353389,
-1.29812354190914));
#69693=CARTESIAN_POINT('Ctrl Pts',(-0.0419392737720405,0.233437524705164,
-1.29816138490414));
#69694=CARTESIAN_POINT('',(-0.237174952428875,-0.000150217712243535,-1.29551725116514));
#69695=CARTESIAN_POINT('Ctrl Pts',(-0.0419392741369039,0.233437524639612,
-1.31805175208418));
#69696=CARTESIAN_POINT('Ctrl Pts',(-0.042730075991894,0.233295449556202,
-1.31799864962229));
#69697=CARTESIAN_POINT('Ctrl Pts',(-0.0435201470678421,0.233149357634431,
-1.31794542141065));
#69698=CARTESIAN_POINT('Ctrl Pts',(-0.0454620452621817,0.232780066948212,
-1.31781415312616));
#69699=CARTESIAN_POINT('Ctrl Pts',(-0.0466129730601121,0.232552333433665,
-1.31773597114705));
#69700=CARTESIAN_POINT('Ctrl Pts',(-0.0490359513137738,0.232054190364414,
-1.31757055131564));
#69701=CARTESIAN_POINT('Ctrl Pts',(-0.050307558321464,0.23178183976685,
-1.31748325375812));
#69702=CARTESIAN_POINT('Ctrl Pts',(-0.0536836674373283,0.231029659408946,
-1.31725015907493));
#69703=CARTESIAN_POINT('Ctrl Pts',(-0.0557839261533372,0.230531543875296,
-1.31710378126733));
#69704=CARTESIAN_POINT('Ctrl Pts',(-0.0663492673567317,0.227872945028406,
-1.31636027600193));
#69705=CARTESIAN_POINT('Ctrl Pts',(-0.0746961947294473,0.225274831226444,
-1.31574922389491));
#69706=CARTESIAN_POINT('Ctrl Pts',(-0.0981163616342415,0.21654006267436,
-1.31396641411693));
#69707=CARTESIAN_POINT('Ctrl Pts',(-0.112727240200996,0.209305772108647,
-1.31276685571552));
#69708=CARTESIAN_POINT('Ctrl Pts',(-0.133385234861601,0.196282870298228,
-1.31099755499191));
#69709=CARTESIAN_POINT('Ctrl Pts',(-0.140060670955096,0.191576679291413,
-1.31041362154172));
#69710=CARTESIAN_POINT('Ctrl Pts',(-0.147517045988519,0.18572139828791,
-1.30975778931733));
#69711=CARTESIAN_POINT('Ctrl Pts',(-0.14854653590204,0.184899008941244,
-1.30966716026067));
#69712=CARTESIAN_POINT('Ctrl Pts',(-0.150210778352039,0.183546686736372,
-1.30952059461133));
#69713=CARTESIAN_POINT('Ctrl Pts',(-0.150849690876075,0.183021952125626,
-1.30946431322245));
#69714=CARTESIAN_POINT('Ctrl Pts',(-0.151990015547791,0.182075383043787,
-1.30936385766208));
#69715=CARTESIAN_POINT('Ctrl Pts',(-0.152492434628887,0.181654802716175,
-1.30931959728962));
#69716=CARTESIAN_POINT('Ctrl Pts',(-0.152998514021164,0.181227578977539,
-1.30927501426978));
#69717=CARTESIAN_POINT('Ctrl Pts',(-0.153003903197675,0.181223029113358,
-1.30927453951051));
#69718=CARTESIAN_POINT('Ctrl Pts',(-0.153014573372623,0.181214019900141,
-1.30927359952144));
#69719=CARTESIAN_POINT('Ctrl Pts',(-0.15301985437923,0.181209560560513,
-1.30927313429093));
#69720=CARTESIAN_POINT('Ctrl Pts',(-0.153030312063891,0.181200729194285,
-1.30927221302026));
#69721=CARTESIAN_POINT('Ctrl Pts',(-0.153035488748899,0.18119635717723,
-1.3092717569795));
#69722=CARTESIAN_POINT('Ctrl Pts',(-0.153045741461448,0.181187697401525,
-1.30927085376493));
#69723=CARTESIAN_POINT('Ctrl Pts',(-0.15305081749675,0.181183409650905,
-1.30927040659045));
#69724=CARTESIAN_POINT('Ctrl Pts',(-0.153060872419423,0.181174915486908,
-1.30926952079929));
#69725=CARTESIAN_POINT('Ctrl Pts',(-0.153065851313057,0.181170709082049,
-1.30926908218206));
#69726=CARTESIAN_POINT('Ctrl Pts',(-0.153075715302852,0.181162374820004,
-1.30926821321026));
#69727=CARTESIAN_POINT('Ctrl Pts',(-0.153080600405643,0.181158246970298,
-1.30926778285511));
#69728=CARTESIAN_POINT('Ctrl Pts',(-0.153090280018972,0.181150067149086,
-1.3092669301251));
#69729=CARTESIAN_POINT('Ctrl Pts',(-0.153095074535158,0.181146015185209,
-1.30926650774975));
#69730=CARTESIAN_POINT('Ctrl Pts',(-0.153104576037755,0.181137984584362,
-1.30926567070958));
#69731=CARTESIAN_POINT('Ctrl Pts',(-0.153109283030601,0.181134005953715,
-1.3092652560442));
#69732=CARTESIAN_POINT('Ctrl Pts',(-0.153118612420609,0.181126119574247,
-1.30926443416548));
#69733=CARTESIAN_POINT('Ctrl Pts',(-0.153123234822777,0.181122211832359,
-1.30926402695171));
#69734=CARTESIAN_POINT('Ctrl Pts',(-0.153132397836263,0.181114464892435,
-1.30926321972914));
#69735=CARTESIAN_POINT('Ctrl Pts',(-0.153136938453594,0.181110625699921,
-1.30926281971982));
#69736=CARTESIAN_POINT('Ctrl Pts',(-0.153145940587735,0.18110301361556,
-1.30926202666915));
#69737=CARTESIAN_POINT('Ctrl Pts',(-0.153150402108979,0.181099240730042,
-1.30926163362742));
#69738=CARTESIAN_POINT('Ctrl Pts',(-0.153159248626411,0.181091759111717,
-1.30926085428506));
#69739=CARTESIAN_POINT('Ctrl Pts',(-0.15316363362728,0.181088050384534,
-1.30926046798403));
#69740=CARTESIAN_POINT('Ctrl Pts',(-0.153172329572949,0.181080695023181,
-1.30925970190556));
#69741=CARTESIAN_POINT('Ctrl Pts',(-0.153176640522496,0.181077048394114,
-1.30925932212772));
#69742=CARTESIAN_POINT('Ctrl Pts',(-0.153185190733487,0.181069815253067,
-1.30925856888705));
#69743=CARTESIAN_POINT('Ctrl Pts',(-0.153189429999315,0.181066228746057,
-1.30925819542383));
#69744=CARTESIAN_POINT('Ctrl Pts',(-0.153197839118215,0.181059113949964,
-1.30925745461198));
#69745=CARTESIAN_POINT('Ctrl Pts',(-0.15320200897386,0.18105558566697,-1.30925708726312));
#69746=CARTESIAN_POINT('Ctrl Pts',(-0.153210281449584,0.181048585501309,
-1.30925635848818));
#69747=CARTESIAN_POINT('Ctrl Pts',(-0.153214384074708,0.18104511362225,
-1.30925599706166));
#69748=CARTESIAN_POINT('Ctrl Pts',(-0.153222524185682,0.181038224513905,
-1.30925527994674));
#69749=CARTESIAN_POINT('Ctrl Pts',(-0.153226561675178,0.181034807289045,
-1.30925492425802));
#69750=CARTESIAN_POINT('Ctrl Pts',(-0.153234573525726,0.181028025809549,
-1.30925421844157));
#69751=CARTESIAN_POINT('Ctrl Pts',(-0.153238547890653,0.1810246615588,-1.3092538683135));
#69752=CARTESIAN_POINT('Ctrl Pts',(-0.153246435430799,0.181017984407744,
-1.30925317344755));
#69753=CARTESIAN_POINT('Ctrl Pts',(-0.153250348607233,0.18101467151325,
-1.30925282870958));
#69754=CARTESIAN_POINT('Ctrl Pts',(-0.153258115622694,0.181008095526915,
-1.30925214446066));
#69755=CARTESIAN_POINT('Ctrl Pts',(-0.153261969467306,0.181004832436878,
-1.30925180494923));
#69756=CARTESIAN_POINT('Ctrl Pts',(-0.153269619612282,0.180998354560623,
-1.30925113099543));
#69757=CARTESIAN_POINT('Ctrl Pts',(-0.153273415914893,0.180995139778744,
-1.30925079655287));
#69758=CARTESIAN_POINT('Ctrl Pts',(-0.153280952694623,0.180988757081913,
-1.30925013258541));
#69759=CARTESIAN_POINT('Ctrl Pts',(-0.153284693175082,0.180985589170099,
-1.30924980306023));
#69760=CARTESIAN_POINT('Ctrl Pts',(-0.153292119970424,0.180979298825339,
-1.30924914878129));
#69761=CARTESIAN_POINT('Ctrl Pts',(-0.153295806286824,0.180976176396815,
-1.30924882402742));
#69762=CARTESIAN_POINT('Ctrl Pts',(-0.153303126344122,0.180969975688781,
-1.30924817915103));
#69763=CARTESIAN_POINT('Ctrl Pts',(-0.153306760089473,0.180966897410959,
-1.30924785902814));
#69764=CARTESIAN_POINT('Ctrl Pts',(-0.15331397654739,0.180960783713698,
-1.30924722327781));
#69765=CARTESIAN_POINT('Ctrl Pts',(-0.153317559260781,0.180957748298785,
-1.30924690765032));
#69766=CARTESIAN_POINT('Ctrl Pts',(-0.153324675130603,0.180951719092528,
-1.3092462807608));
#69767=CARTESIAN_POINT('Ctrl Pts',(-0.153328208291232,0.18094872530263,
-1.3092459694984));
#69768=CARTESIAN_POINT('Ctrl Pts',(-0.153335226485888,0.180942778149307,
-1.30924535121307));
#69769=CARTESIAN_POINT('Ctrl Pts',(-0.153338711522067,0.180939824788851,
-1.30924504418995));
#69770=CARTESIAN_POINT('Ctrl Pts',(-0.15334563484607,0.180933957340709,
-1.30924443426177));
#69771=CARTESIAN_POINT('Ctrl Pts',(-0.153349073135526,0.180931043256233,
-1.30924413135656));
#69772=CARTESIAN_POINT('Ctrl Pts',(-0.153974111205272,0.180401268487822,
-1.30918906694146));
#69773=CARTESIAN_POINT('Ctrl Pts',(-0.154593003363402,0.179871198233511,
-1.30913453806626));
#69774=CARTESIAN_POINT('Ctrl Pts',(-0.156513418482666,0.17820916272353,
-1.30896527184002));
#69775=CARTESIAN_POINT('Ctrl Pts',(-0.157805368327269,0.177066151470791,
-1.30885130671589));
#69776=CARTESIAN_POINT('Ctrl Pts',(-0.160840949646248,0.174320899717232,
-1.30858298542288));
#69777=CARTESIAN_POINT('Ctrl Pts',(-0.162573311824768,0.17270641671578,
-1.30842941912404));
#69778=CARTESIAN_POINT('Ctrl Pts',(-0.168715494165297,0.166807848914186,
-1.30788206772881));
#69779=CARTESIAN_POINT('Ctrl Pts',(-0.172982790538499,0.16237838941339,
-1.30749630022158));
#69780=CARTESIAN_POINT('Ctrl Pts',(-0.190532264389932,0.142683933354184,
-1.3058597150181));
#69781=CARTESIAN_POINT('Ctrl Pts',(-0.202002789868823,0.125921094758135,
-1.30465033655044));
#69782=CARTESIAN_POINT('Ctrl Pts',(-0.213333168216489,0.103743831041836,
-1.30306022406101));
#69783=CARTESIAN_POINT('Ctrl Pts',(-0.215335873966919,0.0995202482763043,
-1.30275823840336));
#69784=CARTESIAN_POINT('Ctrl Pts',(-0.217936690649239,0.093588635341723,
-1.3023337883921));
#69785=CARTESIAN_POINT('Ctrl Pts',(-0.218642086521764,0.0919286217612416,
-1.30221497010903));
#69786=CARTESIAN_POINT('Ctrl Pts',(-0.219747912898177,0.0892415272025777,
-1.30202250882702));
#69787=CARTESIAN_POINT('Ctrl Pts',(-0.220160244942868,0.0882193962646792,
-1.30194927005371));
#69788=CARTESIAN_POINT('Ctrl Pts',(-0.221002999172407,0.0860875809313934,
-1.30179643888395));
#69789=CARTESIAN_POINT('Ctrl Pts',(-0.221432221402953,0.0849774585940837,
-1.30171680868392));
#69790=CARTESIAN_POINT('Ctrl Pts',(-0.222426897684242,0.0823461563325304,
-1.30152793309061));
#69791=CARTESIAN_POINT('Ctrl Pts',(-0.222985123949682,0.0808223270210209,
-1.30141845032215));
#69792=CARTESIAN_POINT('Ctrl Pts',(-0.224806734250036,0.0756871866577657,
-1.30104909428505));
#69793=CARTESIAN_POINT('Ctrl Pts',(-0.225998309472044,0.072051225791986,
-1.30078688038987));
#69794=CARTESIAN_POINT('Ctrl Pts',(-0.23112078003655,0.0550406911746145,
-1.29955625758056));
#69795=CARTESIAN_POINT('Ctrl Pts',(-0.233955043153285,0.0413668760454999,
-1.29855372346693));
#69796=CARTESIAN_POINT('Ctrl Pts',(-0.236645699533647,0.0183393274071569,
-1.29686353817375));
#69797=CARTESIAN_POINT('Ctrl Pts',(-0.237180810115524,0.00909833581418968,
-1.29618544677203));
#69798=CARTESIAN_POINT('Ctrl Pts',(-0.237174952428875,-0.000150217712243535,
-1.29551725116514));
#69799=CARTESIAN_POINT('Ctrl Pts',(-0.237174952219374,-0.000150548123425626,
-1.29551722729338));
#69800=CARTESIAN_POINT('Ctrl Pts',(-0.237171634097938,-0.00537794834055943,
-1.29513955477401));
#69801=CARTESIAN_POINT('Ctrl Pts',(-0.236995496033019,-0.0106042469816567,
-1.29476539307927));
#69802=CARTESIAN_POINT('Ctrl Pts',(-0.236475414555163,-0.018383575706604,
-1.29421726023887));
#69803=CARTESIAN_POINT('Ctrl Pts',(-0.236262459004787,-0.0209434790540369,
-1.29403832264722));
#69804=CARTESIAN_POINT('Ctrl Pts',(-0.235921164725,-0.0243711274954405,
-1.29380108654061));
#69805=CARTESIAN_POINT('Ctrl Pts',(-0.235829550734013,-0.025242243960233,
-1.29374099920503));
#69806=CARTESIAN_POINT('Ctrl Pts',(-0.235660972814824,-0.0267640770103183,
-1.29363640837812));
#69807=CARTESIAN_POINT('Ctrl Pts',(-0.2355861350564,-0.0274150127010362,
-1.29359179371062));
#69808=CARTESIAN_POINT('Ctrl Pts',(-0.235433595423304,-0.0286950261190728,
-1.29350431381029));
#69809=CARTESIAN_POINT('Ctrl Pts',(-0.235356067352883,-0.0293241193842705,
-1.29346143984812));
#69810=CARTESIAN_POINT('Ctrl Pts',(-0.235183068228193,-0.0306830036354225,
-1.2933690960295));
#69811=CARTESIAN_POINT('Ctrl Pts',(-0.235086721484119,-0.0314126680249628,
-1.29331967554479));
#69812=CARTESIAN_POINT('Ctrl Pts',(-0.234816635056893,-0.0333872502279775,
-1.29318635247581));
#69813=CARTESIAN_POINT('Ctrl Pts',(-0.23463638991153,-0.0346312760248702,
-1.29310280491599));
#69814=CARTESIAN_POINT('Ctrl Pts',(-0.233738782597306,-0.0404974072691783,
-1.29271070994837));
#69815=CARTESIAN_POINT('Ctrl Pts',(-0.232894630751464,-0.0450994062680839,
-1.29240859214907));
#69816=CARTESIAN_POINT('Ctrl Pts',(-0.230619787514339,-0.0557200987495107,
-1.29171782944799));
#69817=CARTESIAN_POINT('Ctrl Pts',(-0.229088689447391,-0.0617138335465195,
-1.2913328760493));
#69818=CARTESIAN_POINT('Ctrl Pts',(-0.222727433056254,-0.0830924110380073,
-1.28995607619125));
#69819=CARTESIAN_POINT('Ctrl Pts',(-0.216566812966617,-0.0980339839073789,
-1.28898367988846));
#69820=CARTESIAN_POINT('Ctrl Pts',(-0.20570165626276,-0.118260699163556,
-1.28753621870337));
#69821=CARTESIAN_POINT('Ctrl Pts',(-0.202206053653733,-0.124142911784749,
-1.28709834196644));
#69822=CARTESIAN_POINT('Ctrl Pts',(-0.197364389524526,-0.131541980008034,
-1.28652028957603));
#69823=CARTESIAN_POINT('Ctrl Pts',(-0.196246183779255,-0.133204465774659,
-1.28638855865525));
#69824=CARTESIAN_POINT('Ctrl Pts',(-0.194386793057418,-0.135894665593498,
-1.2861722417754));
#69825=CARTESIAN_POINT('Ctrl Pts',(-0.193658182465301,-0.136930981557038,
-1.28608813367788));
#69826=CARTESIAN_POINT('Ctrl Pts',(-0.192232963770691,-0.138923967124943,
-1.28592483948853));
#69827=CARTESIAN_POINT('Ctrl Pts',(-0.191537427492375,-0.139881359672107,
-1.28584569629284));
#69828=CARTESIAN_POINT('Ctrl Pts',(-0.189912248950479,-0.142083538730366,
-1.28566200207196));
#69829=CARTESIAN_POINT('Ctrl Pts',(-0.188977490960681,-0.1433244640304,
-1.28555725374669));
#69830=CARTESIAN_POINT('Ctrl Pts',(-0.185886145086666,-0.147345517049598,
-1.28521370262834));
#69831=CARTESIAN_POINT('Ctrl Pts',(-0.183679962746033,-0.150086739263715,
-1.28497295477629));
#69832=CARTESIAN_POINT('Ctrl Pts',(-0.168912809352094,-0.167621781113879,
-1.28338873371208));
#69833=CARTESIAN_POINT('Ctrl Pts',(-0.154639268560768,-0.18087292746228,
-1.28197236788306));
#69834=CARTESIAN_POINT('Ctrl Pts',(-0.13745828529144,-0.193288471559709,
-1.28042601100721));
#69835=CARTESIAN_POINT('Ctrl Pts',(-0.135989027908764,-0.194324979914469,
-1.28029497955843));
#69836=CARTESIAN_POINT('Ctrl Pts',(-0.129023477869157,-0.199121235296442,
-1.27967979088504));
#69837=CARTESIAN_POINT('Ctrl Pts',(-0.123381836011182,-0.202665385995047,
-1.27919884255916));
#69838=CARTESIAN_POINT('Ctrl Pts',(-0.115433704140734,-0.20720340892685,
-1.27855105574359));
#69839=CARTESIAN_POINT('Ctrl Pts',(-0.113249803560968,-0.208405076251547,
-1.2783760361788));
#69840=CARTESIAN_POINT('Ctrl Pts',(-0.109915405330685,-0.21017189422047,
-1.27811371159392));
#69841=CARTESIAN_POINT('Ctrl Pts',(-0.108778667310689,-0.210762480438063,
-1.27802512910914));
#69842=CARTESIAN_POINT('Ctrl Pts',(-0.106683914014119,-0.211829335827046,
-1.27786351424136));
#69843=CARTESIAN_POINT('Ctrl Pts',(-0.105727360575849,-0.212308385047584,
-1.27779032816967));
#69844=CARTESIAN_POINT('Ctrl Pts',(-0.104148176050817,-0.213085932704761,
-1.27767055123375));
#69845=CARTESIAN_POINT('Ctrl Pts',(-0.1035274373105,-0.213388207374404,
-1.27762373393007));
#69846=CARTESIAN_POINT('Ctrl Pts',(-0.102300169901742,-0.213979221144839,
-1.27753170390752));
#69847=CARTESIAN_POINT('Ctrl Pts',(-0.101693721967763,-0.214268100222872,
-1.27748648379952));
#69848=CARTESIAN_POINT('Ctrl Pts',(-0.100332867286164,-0.214909258926846,
-1.27738556559921));
#69849=CARTESIAN_POINT('Ctrl Pts',(-0.0995778086216152,-0.215260154028732,
-1.2773299515766));
#69850=CARTESIAN_POINT('Ctrl Pts',(-0.09694003186964,-0.216469147219884,
-1.27713693117663));
#69851=CARTESIAN_POINT('Ctrl Pts',(-0.0950478812284026,-0.217306609345889,
-1.27700070935946));
#69852=CARTESIAN_POINT('Ctrl Pts',(-0.0820238171277684,-0.222868363670622,
-1.27607666430147));
#69853=CARTESIAN_POINT('Ctrl Pts',(-0.0705542621662209,-0.22676063497048,
-1.27532986130998));
#69854=CARTESIAN_POINT('Ctrl Pts',(-0.0484440247797162,-0.232422554556084,
-1.273928823142));
#69855=CARTESIAN_POINT('Ctrl Pts',(-0.0378830685748147,-0.234375620482233,
-1.27327520930931));
#69856=CARTESIAN_POINT('Ctrl Pts',(-0.0180321672712933,-0.236669574006756,
-1.27203002205858));
#69857=CARTESIAN_POINT('Ctrl Pts',(-0.00878445716549035,-0.237192852391894,
-1.27144342271638));
#69858=CARTESIAN_POINT('Ctrl Pts',(0.00266243741233339,-0.237170194644882,
-1.27069670591225));
#69859=CARTESIAN_POINT('Ctrl Pts',(0.00485518784719147,-0.237135438983914,
-1.27055275456942));
#69860=CARTESIAN_POINT('Ctrl Pts',(0.0083544466254571,-0.237031421036525,
-1.27032143403947));
#69861=CARTESIAN_POINT('Ctrl Pts',(0.0096614444347577,-0.236981745525032,
-1.27023467817484));
#69862=CARTESIAN_POINT('Ctrl Pts',(0.0121383832377233,-0.236867079064401,
-1.27006955854794));
#69863=CARTESIAN_POINT('Ctrl Pts',(0.0133083877502891,-0.236804223405379,
-1.2699912640744));
#69864=CARTESIAN_POINT('Ctrl Pts',(0.0159695621484252,-0.236641473976454,
-1.26981248080178));
#69865=CARTESIAN_POINT('Ctrl Pts',(0.0174603375210886,-0.236536150633577,
-1.26971182471406));
#69866=CARTESIAN_POINT('Ctrl Pts',(0.022041762181863,-0.236168926455461,
-1.26940089093279));
#69867=CARTESIAN_POINT('Ctrl Pts',(0.0251282419003797,-0.235860490488281,
-1.26918917014795));
#69868=CARTESIAN_POINT('Ctrl Pts',(0.0460643524293472,-0.233352720933325,
-1.26773707333084));
#69869=CARTESIAN_POINT('Ctrl Pts',(0.063616607020624,-0.229190111206138,
-1.26643391523741));
#69870=CARTESIAN_POINT('Ctrl Pts',(0.0843219399406033,-0.221716201527491,
-1.2648261583496));
#69871=CARTESIAN_POINT('Ctrl Pts',(0.0880819126316785,-0.220249497086493,
-1.26453151117589));
#69872=CARTESIAN_POINT('Ctrl Pts',(0.0978193820114174,-0.216161812915336,
-1.26376362443696));
#69873=CARTESIAN_POINT('Ctrl Pts',(0.103729718730266,-0.213388654317691,
-1.26329263026846));
#69874=CARTESIAN_POINT('Ctrl Pts',(0.112762165808324,-0.208686480800197,
-1.26257216424315));
#69875=CARTESIAN_POINT('Ctrl Pts',(0.115966559720571,-0.206922966262217,
-1.2623164495848));
#69876=CARTESIAN_POINT('Ctrl Pts',(0.120091978619876,-0.204526617525639,
-1.26198828144166));
#69877=CARTESIAN_POINT('Ctrl Pts',(0.121050936636414,-0.203960514482649,
-1.26191207415715));
#69878=CARTESIAN_POINT('Ctrl Pts',(0.122609901682587,-0.203025340134603,
-1.26178835347969));
#69879=CARTESIAN_POINT('Ctrl Pts',(0.123212300933918,-0.20266032087964,
-1.26174058807389));
#69880=CARTESIAN_POINT('Ctrl Pts',(0.124386129497664,-0.201941879811416,
-1.26164760774918));
#69881=CARTESIAN_POINT('Ctrl Pts',(0.124957695741152,-0.201588705848002,
-1.26160237854773));
#69882=CARTESIAN_POINT('Ctrl Pts',(0.126234628231357,-0.2007921645663,-1.26150141617112));
#69883=CARTESIAN_POINT('Ctrl Pts',(0.126939181884179,-0.200347495294068,
-1.26144576730652));
#69884=CARTESIAN_POINT('Ctrl Pts',(0.129387855789633,-0.198783945879309,
-1.2612525072822));
#69885=CARTESIAN_POINT('Ctrl Pts',(0.131119704425123,-0.197645890911342,
-1.26111608454046));
#69886=CARTESIAN_POINT('Ctrl Pts',(0.142889682698122,-0.189688638844779,
-1.26018910740534));
#69887=CARTESIAN_POINT('Ctrl Pts',(0.152407791396253,-0.18212957541118,
-1.25943985144953));
#69888=CARTESIAN_POINT('Ctrl Pts',(0.169227325834228,-0.166525773452984,
-1.25803158513234));
#69889=CARTESIAN_POINT('Ctrl Pts',(0.176636746286817,-0.15864479611635,
-1.25737326660319));
#69890=CARTESIAN_POINT('Ctrl Pts',(0.189277757269659,-0.143211545128199,
-1.25612959322725));
#69891=CARTESIAN_POINT('Ctrl Pts',(0.194657998254533,-0.135808137752186,
-1.25554972705993));
#69892=CARTESIAN_POINT('Ctrl Pts',(0.200777796390083,-0.126273652379607,
-1.25481061043636));
#69893=CARTESIAN_POINT('Ctrl Pts',(0.201933020777368,-0.124417898244251,
-1.25466711528058));
#69894=CARTESIAN_POINT('Ctrl Pts',(0.203737408712755,-0.121427985283587,
-1.25443635532781));
#69895=CARTESIAN_POINT('Ctrl Pts',(0.2044031534096,-0.120303940414581,-1.25434969855404));
#69896=CARTESIAN_POINT('Ctrl Pts',(0.205648464610499,-0.118161174672097,
-1.25418465658479));
#69897=CARTESIAN_POINT('Ctrl Pts',(0.206229834282845,-0.117143542558504,
-1.25410633974369));
#69898=CARTESIAN_POINT('Ctrl Pts',(0.207536655641705,-0.114816195516537,
-1.25392735013452));
#69899=CARTESIAN_POINT('Ctrl Pts',(0.208257289599811,-0.113503847235874,
-1.25382650862904));
#69900=CARTESIAN_POINT('Ctrl Pts',(0.210439272130048,-0.109439491171847,
-1.25351441662176));
#69901=CARTESIAN_POINT('Ctrl Pts',(0.211858800665463,-0.106665535448604,
-1.25330170739145));
#69902=CARTESIAN_POINT('Ctrl Pts',(0.221009786292477,-0.0878795019611069,
-1.25186248216073));
#69903=CARTESIAN_POINT('Ctrl Pts',(0.226972714652791,-0.071072425063611,
-1.25057478603627));
#69904=CARTESIAN_POINT('Ctrl Pts',(0.23196578719813,-0.0496180113711474,
-1.2489659391383));
#69905=CARTESIAN_POINT('Ctrl Pts',(0.23281833876877,-0.0454499222168456,
-1.24865529365496));
#69906=CARTESIAN_POINT('Ctrl Pts',(0.234689074717624,-0.0348606316198101,
-1.24787346617379));
#69907=CARTESIAN_POINT('Ctrl Pts',(0.235556304334753,-0.0284159164161385,
-1.24740438800428));
#69908=CARTESIAN_POINT('Ctrl Pts',(0.236495178386044,-0.0183115955785285,
-1.24668646901585));
#69909=CARTESIAN_POINT('Ctrl Pts',(0.23674883461385,-0.0146723157346005,
-1.24643143326267));
#69910=CARTESIAN_POINT('Ctrl Pts',(0.236970187826219,-0.00991707694313436,
-1.24610399498103));
#69911=CARTESIAN_POINT('Ctrl Pts',(0.23701410034066,-0.0088053788183978,
-1.2460278586963));
#69912=CARTESIAN_POINT('Ctrl Pts',(0.237073029712417,-0.00698963480971464,
-1.24590422403685));
#69913=CARTESIAN_POINT('Ctrl Pts',(0.237092736053673,-0.00628577405220784,
-1.24585647429257));
#69914=CARTESIAN_POINT('Ctrl Pts',(0.237125123592204,-0.00490998964807286,
-1.2457634996832));
#69915=CARTESIAN_POINT('Ctrl Pts',(0.237138084012521,-0.00423808508776454,
-1.2457182607038));
#69916=CARTESIAN_POINT('Ctrl Pts',(0.237160723874961,-0.00273252965416426,
-1.24561725088874));
#69917=CARTESIAN_POINT('Ctrl Pts',(0.23716886402977,-0.00189885603442453,
-1.2455615646223));
#69918=CARTESIAN_POINT('Ctrl Pts',(0.237181929114934,0.0010103171958684,
-1.24536804708988));
#69919=CARTESIAN_POINT('Ctrl Pts',(0.237164006983026,0.0030858956645106,
-1.24523140839519));
#69920=CARTESIAN_POINT('Ctrl Pts',(0.236855975696026,0.0172380391428393,
-1.24430785743533));
#69921=CARTESIAN_POINT('Ctrl Pts',(0.235670793260351,0.029278926256905,
-1.24356183886617));
#69922=CARTESIAN_POINT('Ctrl Pts',(0.231711387432897,0.0517375644353026,
-1.24216194126137));
#69923=CARTESIAN_POINT('Ctrl Pts',(0.229135961708477,0.0621582230070684,
-1.24150868345963));
#69924=CARTESIAN_POINT('Ctrl Pts',(0.223037868932548,0.0811905635582971,
-1.24026338897375));
#69925=CARTESIAN_POINT('Ctrl Pts',(0.219697109667137,0.0898384556896925,
-1.23967628809932));
#69926=CARTESIAN_POINT('Ctrl Pts',(0.214950711467635,0.100264568671081,
-1.23892900526597));
#69927=CARTESIAN_POINT('Ctrl Pts',(0.214014255955503,0.102248177533602,
-1.23878502026979));
#69928=CARTESIAN_POINT('Ctrl Pts',(0.212475667693255,0.105393464085221,
-1.23855365838525));
#69929=CARTESIAN_POINT('Ctrl Pts',(0.211891186815793,0.106563673299053,
-1.23846689521107));
#69930=CARTESIAN_POINT('Ctrl Pts',(0.210764872071161,0.108772800560645,
-1.23830176983211));
#69931=CARTESIAN_POINT('Ctrl Pts',(0.210224959086611,0.10981265834605,-1.23822347698485));
#69932=CARTESIAN_POINT('Ctrl Pts',(0.2089789850388,0.112169502729805,-1.23804470881742));
#69933=CARTESIAN_POINT('Ctrl Pts',(0.208268143699632,0.113483891686965,
-1.23794406631471));
#69934=CARTESIAN_POINT('Ctrl Pts',(0.206044245486363,0.117504738436927,
-1.23763321728866));
#69935=CARTESIAN_POINT('Ctrl Pts',(0.204490550029108,0.12018821911787,-1.23742156881495));
#69936=CARTESIAN_POINT('Ctrl Pts',(0.193562812987793,0.138236613078181,
-1.23596858660539));
#69937=CARTESIAN_POINT('Ctrl Pts',(0.182520295047895,0.152518942990879,
-1.23466435896758));
#69938=CARTESIAN_POINT('Ctrl Pts',(0.16716816342122,0.168294240120174,-1.2330566403756));
#69939=CARTESIAN_POINT('Ctrl Pts',(0.164291207948998,0.171103903604674,
-1.23276306133683));
#69940=CARTESIAN_POINT('Ctrl Pts',(0.156560298139525,0.178279144287022,
-1.23199612319711));
#69941=CARTESIAN_POINT('Ctrl Pts',(0.151594827651014,0.182520135753204,
-1.2315250185454));
#69942=CARTESIAN_POINT('Ctrl Pts',(0.143583662718532,0.188809663702404,
-1.23080440570332));
#69943=CARTESIAN_POINT('Ctrl Pts',(0.140654847328787,0.191001504876608,
-1.23054865194719));
#69944=CARTESIAN_POINT('Ctrl Pts',(0.136769538780253,0.19377129301799,-1.23022044177899));
#69945=CARTESIAN_POINT('Ctrl Pts',(0.135858199523805,0.194411343499961,
-1.23014423041142));
#69946=CARTESIAN_POINT('Ctrl Pts',(0.134363122329689,0.195445716513194,
-1.23002050478715));
#69947=CARTESIAN_POINT('Ctrl Pts',(0.133782089102471,0.195843890417862,
-1.22997273848062));
#69948=CARTESIAN_POINT('Ctrl Pts',(0.132643381187188,0.19661679849068,-1.22987975782549));
#69949=CARTESIAN_POINT('Ctrl Pts',(0.13208587589669,0.196991759795486,-1.22983452918468));
#69950=CARTESIAN_POINT('Ctrl Pts',(0.130833527225999,0.197826345098317,
-1.22973356953006));
#69951=CARTESIAN_POINT('Ctrl Pts',(0.130137833216007,0.198284691994349,
-1.22967792281197));
#69952=CARTESIAN_POINT('Ctrl Pts',(0.127703553831087,0.199870147618594,
-1.22948467755738));
#69953=CARTESIAN_POINT('Ctrl Pts',(0.125952566342138,0.200978171250738,
-1.22934826720088));
#69954=CARTESIAN_POINT('Ctrl Pts',(0.113845466299531,0.208419146874247,
-1.22842105879279));
#69955=CARTESIAN_POINT('Ctrl Pts',(0.103029617362843,0.213972673431457,
-1.22767158618039));
#69956=CARTESIAN_POINT('Ctrl Pts',(0.0815401133080914,0.222997451456266,
-1.22624093729439));
#69957=CARTESIAN_POINT('Ctrl Pts',(0.0709533259188437,0.226588322450777,
-1.22556077352529));
#69958=CARTESIAN_POINT('Ctrl Pts',(0.051619799452518,0.231657509786112,
-1.2243130137973));
#69959=CARTESIAN_POINT('Ctrl Pts',(0.04296910465984,0.233416868901416,-1.22375291593235));
#69960=CARTESIAN_POINT('Ctrl Pts',(0.0320994835168327,0.235002741120943,
-1.22303612638464));
#69961=CARTESIAN_POINT('Ctrl Pts',(0.029953659643311,0.235285874927931,
-1.22289401866229));
#69962=CARTESIAN_POINT('Ctrl Pts',(0.0265115650955223,0.235692197664414,
-1.22266496356337));
#69963=CARTESIAN_POINT('Ctrl Pts',(0.0252175998501376,0.235834152884497,
-1.22257860821001));
#69964=CARTESIAN_POINT('Ctrl Pts',(0.0227555712173413,0.236083757272413,
-1.22241379870537));
#69965=CARTESIAN_POINT('Ctrl Pts',(0.0215877461187253,0.236193407193166,
-1.22233541004592));
#69966=CARTESIAN_POINT('Ctrl Pts',(0.018919161480489,0.236424010608196,
-1.22215577434696));
#69967=CARTESIAN_POINT('Ctrl Pts',(0.0174179800874936,0.236539343980611,
-1.22205435404391));
#69968=CARTESIAN_POINT('Ctrl Pts',(0.0127624308503408,0.236852464425862,
-1.22173862924454));
#69969=CARTESIAN_POINT('Ctrl Pts',(0.00960524562776476,0.237001491813655,
-1.22152281641792));
#69970=CARTESIAN_POINT('Ctrl Pts',(-0.00976928912817915,0.237528264782934,
-1.22018739965351));
#69971=CARTESIAN_POINT('Ctrl Pts',(-0.0259825454949993,0.236304302883026,
-1.21901805622511));
#69972=CARTESIAN_POINT('Ctrl Pts',(-0.0419392741364228,0.233437524639699,
-1.21783461098805));
#69973=CARTESIAN_POINT('Origin',(0.,0.,-2.1456589891905));
#69974=CARTESIAN_POINT('',(-0.0419392646935193,0.233437526336206,-1.0979250019446));
#69975=CARTESIAN_POINT('',(-0.0419392769977373,0.233437524125636,-1.11762795217595));
#69976=CARTESIAN_POINT('',(-0.0419392741328076,0.233437524640348,-2.1456589891905));
#69977=CARTESIAN_POINT('Ctrl Pts',(-0.0419392646935193,0.233437526336206,
-1.0979250019446));
#69978=CARTESIAN_POINT('Ctrl Pts',(-0.0367798115508998,0.234364471007092,
-1.09829310188845));
#69979=CARTESIAN_POINT('Ctrl Pts',(-0.031590035201231,0.23512029192747,
-1.09866598315669));
#69980=CARTESIAN_POINT('Ctrl Pts',(-0.0133490694662614,0.237161701207052,
-1.09998416170587));
#69981=CARTESIAN_POINT('Ctrl Pts',(-0.000221727773968937,0.237536913602359,
-1.1009477883589));
#69982=CARTESIAN_POINT('Ctrl Pts',(0.0193563500274205,0.236473110189919,
-1.10237332585635));
#69983=CARTESIAN_POINT('Ctrl Pts',(0.0258276626338947,0.235854072157193,
-1.10284226038659));
#69984=CARTESIAN_POINT('Ctrl Pts',(0.0358787685837513,0.234473867315965,
-1.10356000704841));
#69985=CARTESIAN_POINT('Ctrl Pts',(0.0394800893702072,0.23389443481767,
-1.10381500967153));
#69986=CARTESIAN_POINT('Ctrl Pts',(0.0441610573851744,0.233030083373694,
-1.10414242886719));
#69987=CARTESIAN_POINT('Ctrl Pts',(0.0452538604207088,0.232820331987028,
-1.1042185779424));
#69988=CARTESIAN_POINT('Ctrl Pts',(0.0470359159133121,0.232465264728848,
-1.10434223876748));
#69989=CARTESIAN_POINT('Ctrl Pts',(0.0477260532844254,0.2323245586722,-1.10439000193132));
#69990=CARTESIAN_POINT('Ctrl Pts',(0.0490737017725887,0.232043539874739,
-1.10448300818268));
#69991=CARTESIAN_POINT('Ctrl Pts',(0.0497312576145336,0.231903502855761,
-1.10452826535584));
#69992=CARTESIAN_POINT('Ctrl Pts',(0.0512033081783561,0.231583457172682,
-1.10462932263763));
#69993=CARTESIAN_POINT('Ctrl Pts',(0.052017474941726,0.231401941991485,
-1.10468503804935));
#69994=CARTESIAN_POINT('Ctrl Pts',(0.0548556102051486,0.230753455134415,
-1.10487869201424));
#69995=CARTESIAN_POINT('Ctrl Pts',(0.0568744577165943,0.230264178302399,
-1.10501543606347));
#69996=CARTESIAN_POINT('Ctrl Pts',(0.0705690603839299,0.226754121710169,
-1.10593777814762));
#69997=CARTESIAN_POINT('Ctrl Pts',(0.0820076009509888,0.222872726372553,
-1.10668263029302));
#69998=CARTESIAN_POINT('Ctrl Pts',(0.102936149509307,0.213940290431936,
-1.10807949606692));
#69999=CARTESIAN_POINT('Ctrl Pts',(0.11247468719825,0.209083080794677,-1.10873091381997));
#70000=CARTESIAN_POINT('Ctrl Pts',(0.129640777566244,0.198826156133788,
-1.10997670938076));
#70001=CARTESIAN_POINT('Ctrl Pts',(0.137340197346523,0.193587734490092,
-1.11056634640951));
#70002=CARTESIAN_POINT('Ctrl Pts',(0.146451822214929,0.186570816349023,
-1.1113165218975));
#70003=CARTESIAN_POINT('Ctrl Pts',(0.148173422293269,0.185206485136998,
-1.11146070741456));
#70004=CARTESIAN_POINT('Ctrl Pts',(0.150890307651567,0.182991281763887,
-1.11169233453881));
#70005=CARTESIAN_POINT('Ctrl Pts',(0.151897954224711,0.182155717808926,
-1.11177916024021));
#70006=CARTESIAN_POINT('Ctrl Pts',(0.153794553928681,0.180556332893498,
-1.11194436846431));
#70007=CARTESIAN_POINT('Ctrl Pts',(0.15468486571532,0.179794177880297,-1.11202268127352));
#70008=CARTESIAN_POINT('Ctrl Pts',(0.156697138930992,0.178045553509669,
-1.11220144501785));
#70009=CARTESIAN_POINT('Ctrl Pts',(0.157815492417706,0.177055027177479,
-1.11230206278249));
#70010=CARTESIAN_POINT('Ctrl Pts',(0.161223420302418,0.173978682412576,
-1.11261265044438));
#70011=CARTESIAN_POINT('Ctrl Pts',(0.163481476618586,0.171858600042796,
-1.1128240583128));
#70012=CARTESIAN_POINT('Ctrl Pts',(0.178610843598396,0.157085654089708,
-1.11428022246442));
#70013=CARTESIAN_POINT('Ctrl Pts',(0.190040553507443,0.143045743158656,
-1.11558827187724));
#70014=CARTESIAN_POINT('Ctrl Pts',(0.201906429152834,0.124505177128304,
-1.1171959901742));
#70015=CARTESIAN_POINT('Ctrl Pts',(0.203962424799734,0.121107700972162,
-1.11748589388616));
#70016=CARTESIAN_POINT('Ctrl Pts',(0.20917166458411,0.111990341899366,-1.11824942549489));
#70017=CARTESIAN_POINT('Ctrl Pts',(0.212175837015832,0.106188735867266,
-1.11872076896283));
#70018=CARTESIAN_POINT('Ctrl Pts',(0.216483745098903,0.0969544007845552,
-1.11944171790206));
#70019=CARTESIAN_POINT('Ctrl Pts',(0.217953760856338,0.0936030421037136,
-1.11969757404781));
#70020=CARTESIAN_POINT('Ctrl Pts',(0.219769482891282,0.0891885418279303,
-1.12002591083231));
#70021=CARTESIAN_POINT('Ctrl Pts',(0.220185980272891,0.0881552937625912,
-1.12010214917583));
#70022=CARTESIAN_POINT('Ctrl Pts',(0.220854006462542,0.0864637780669202,
-1.12022591815117));
#70023=CARTESIAN_POINT('Ctrl Pts',(0.221109903353052,0.085807271023417,
-1.12027370100594));
#70024=CARTESIAN_POINT('Ctrl Pts',(0.221604170550213,0.0845223280651768,
-1.12036671443582));
#70025=CARTESIAN_POINT('Ctrl Pts',(0.221842800630041,0.0838940055824742,
-1.12041195930821));
#70026=CARTESIAN_POINT('Ctrl Pts',(0.222371345300429,0.0824843015167374,
-1.12051295692071));
#70027=CARTESIAN_POINT('Ctrl Pts',(0.222659821661279,0.0817023810996366,
-1.1205686252894));
#70028=CARTESIAN_POINT('Ctrl Pts',(0.22365140598166,0.0789704132263401,
-1.12076195530891));
#70029=CARTESIAN_POINT('Ctrl Pts',(0.224333090305032,0.0770126150389728,
-1.12089842768379));
#70030=CARTESIAN_POINT('Ctrl Pts',(0.228825646436232,0.0635438726050909,
-1.12182479702267));
#70031=CARTESIAN_POINT('Ctrl Pts',(0.231775069070963,0.0517628573007589,
-1.12257346983025));
#70032=CARTESIAN_POINT('Ctrl Pts',(0.235621768978044,0.0291686353468052,
-1.12398030776406));
#70033=CARTESIAN_POINT('Ctrl Pts',(0.236704743517519,0.0184196155076348,
-1.12463779243811));
#70034=CARTESIAN_POINT('Ctrl Pts',(0.237347089273772,-0.0015250323724891,
-1.12588170695414));
#70035=CARTESIAN_POINT('Ctrl Pts',(0.237110933519941,-0.0106930850971394,
-1.1264627391622));
#70036=CARTESIAN_POINT('Ctrl Pts',(0.236162235121939,-0.0220037496602497,
-1.12720320249862));
#70037=CARTESIAN_POINT('Ctrl Pts',(0.235949240789082,-0.0241810161489934,
-1.12734680811525));
#70038=CARTESIAN_POINT('Ctrl Pts',(0.235560924218474,-0.0276539330917851,
-1.12757772263743));
#70039=CARTESIAN_POINT('Ctrl Pts',(0.235404950321511,-0.0289516542205399,
-1.12766442238254));
#70040=CARTESIAN_POINT('Ctrl Pts',(0.235088744104658,-0.0314107855699627,
-1.12782953169399));
#70041=CARTESIAN_POINT('Ctrl Pts',(0.234930610544518,-0.0325724300424209,
-1.12790787273382));
#70042=CARTESIAN_POINT('Ctrl Pts',(0.234550908608133,-0.0352149678859291,
-1.12808689777618));
#70043=CARTESIAN_POINT('Ctrl Pts',(0.234323917078178,-0.0366950187103823,
-1.1281877504441));
#70044=CARTESIAN_POINT('Ctrl Pts',(0.233581549313853,-0.0412473611854537,
-1.12849980461081));
#70045=CARTESIAN_POINT('Ctrl Pts',(0.233019663927399,-0.0443116192241604,
-1.12871246385869));
#70046=CARTESIAN_POINT('Ctrl Pts',(0.228843687765467,-0.0648016750872356,
-1.13015271215553));
#70047=CARTESIAN_POINT('Ctrl Pts',(0.223339037346654,-0.0817810165075423,
-1.13144160255495));
#70048=CARTESIAN_POINT('Ctrl Pts',(0.214238724560909,-0.101841608410182,
-1.13305048358938));
#70049=CARTESIAN_POINT('Ctrl Pts',(0.212384604892954,-0.105653796513923,
-1.13336001369849));
#70050=CARTESIAN_POINT('Ctrl Pts',(0.207430924343587,-0.115180884623488,
-1.13414073118266));
#70051=CARTESIAN_POINT('Ctrl Pts',(0.204196553583779,-0.120822197665742,
-1.13460980553231));
#70052=CARTESIAN_POINT('Ctrl Pts',(0.198791537851994,-0.129411012014511,
-1.13532773813752));
#70053=CARTESIAN_POINT('Ctrl Pts',(0.196777667369966,-0.132453156944946,
-1.13558279037206));
#70054=CARTESIAN_POINT('Ctrl Pts',(0.19405879078727,-0.136361301808681,
-1.13591026291336));
#70055=CARTESIAN_POINT('Ctrl Pts',(0.19341685635394,-0.13727031257325,-1.13598641718555));
#70056=CARTESIAN_POINT('Ctrl Pts',(0.192358195844793,-0.138747256569972,
-1.13611008430678));
#70057=CARTESIAN_POINT('Ctrl Pts',(0.191945304720318,-0.139317898144015,
-1.13615784861687));
#70058=CARTESIAN_POINT('Ctrl Pts',(0.191133356275669,-0.140429600537358,
-1.13625085528365));
#70059=CARTESIAN_POINT('Ctrl Pts',(0.190734531869393,-0.14097081598071,
-1.13629611173832));
#70060=CARTESIAN_POINT('Ctrl Pts',(0.189835746786442,-0.142179694670568,
-1.13639716553758));
#70061=CARTESIAN_POINT('Ctrl Pts',(0.189334549333362,-0.142846437882056,
-1.13645287820429));
#70062=CARTESIAN_POINT('Ctrl Pts',(0.187573158094216,-0.145164060184163,
-1.13664651325399));
#70063=CARTESIAN_POINT('Ctrl Pts',(0.186294762984918,-0.146801076335037,
-1.13678324143866));
#70064=CARTESIAN_POINT('Ctrl Pts',(0.17744585521328,-0.157830524743763,
-1.13770579236312));
#70065=CARTESIAN_POINT('Ctrl Pts',(0.169188828676269,-0.16665149611595,
-1.13845084416637));
#70066=CARTESIAN_POINT('Ctrl Pts',(0.152411067473868,-0.182036478942389,
-1.13984824140794));
#70067=CARTESIAN_POINT('Ctrl Pts',(0.144046763855794,-0.188724492665677,
-1.14049998640912));
#70068=CARTESIAN_POINT('Ctrl Pts',(0.127622223267001,-0.200127459957259,
-1.14174568685739));
#70069=CARTESIAN_POINT('Ctrl Pts',(0.119680166058774,-0.204975752704548,
-1.14233486674289));
#70070=CARTESIAN_POINT('Ctrl Pts',(0.109536259108629,-0.210377307727473,
-1.14308452634287));
#70071=CARTESIAN_POINT('Ctrl Pts',(0.10758362260767,-0.211382514132093,
-1.14322868138569));
#70072=CARTESIAN_POINT('Ctrl Pts',(0.104445394837434,-0.212943310233738,
-1.14346027106186));
#70073=CARTESIAN_POINT('Ctrl Pts',(0.103268643717226,-0.213516465370341,
-1.14354709014467));
#70074=CARTESIAN_POINT('Ctrl Pts',(0.101029351992212,-0.214584305688889,
-1.14371229314744));
#70075=CARTESIAN_POINT('Ctrl Pts',(0.0999677676067785,-0.215080913998919,
-1.14379060741616));
#70076=CARTESIAN_POINT('Ctrl Pts',(0.0975445528363097,-0.216192676143264,
-1.14396938477424));
#70077=CARTESIAN_POINT('Ctrl Pts',(0.0961807139521616,-0.216802866890058,
-1.14407001478885));
#70078=CARTESIAN_POINT('Ctrl Pts',(0.0919714157627855,-0.218638600606687,
-1.14438067882214));
#70079=CARTESIAN_POINT('Ctrl Pts',(0.0891077336828184,-0.219821266503457,
-1.14459215183858));
#70080=CARTESIAN_POINT('Ctrl Pts',(0.0694195379427486,-0.227504324527932,
-1.14604754065849));
#70081=CARTESIAN_POINT('Ctrl Pts',(0.0519271782830554,-0.232121991604896,
-1.14735465096144));
#70082=CARTESIAN_POINT('Ctrl Pts',(0.0301428343547714,-0.235285476744169,
-1.14896239364466));
#70083=CARTESIAN_POINT('Ctrl Pts',(0.0261872018706163,-0.235758514571029,
-1.14925322542085));
#70084=CARTESIAN_POINT('Ctrl Pts',(0.0157214208982848,-0.23674341107059,
-1.15001758514916));
#70085=CARTESIAN_POINT('Ctrl Pts',(0.00919840287627271,-0.237086496105111,
-1.15048883640984));
#70086=CARTESIAN_POINT('Ctrl Pts',(-0.000989006725740775,-0.237201151451644,
-1.15120966282682));
#70087=CARTESIAN_POINT('Ctrl Pts',(-0.00464787538912799,-0.237157680196853,
-1.15146548635012));
#70088=CARTESIAN_POINT('Ctrl Pts',(-0.00941777121983237,-0.236990563271742,
-1.15179378807042));
#70089=CARTESIAN_POINT('Ctrl Pts',(-0.0105307707046329,-0.236943715861734,
-1.15187002300753));
#70090=CARTESIAN_POINT('Ctrl Pts',(-0.0123471672718733,-0.236854437436524,
-1.15199378785587));
#70091=CARTESIAN_POINT('Ctrl Pts',(-0.0130507625365456,-0.236816711199495,
-1.15204156995918));
#70092=CARTESIAN_POINT('Ctrl Pts',(-0.0144251695490441,-0.236736872582281,
-1.15213458311347));
#70093=CARTESIAN_POINT('Ctrl Pts',(-0.0150959851280274,-0.236695043477522,
-1.15217982845365));
#70094=CARTESIAN_POINT('Ctrl Pts',(-0.0165982208412435,-0.236594958352632,
-1.15228082833727));
#70095=CARTESIAN_POINT('Ctrl Pts',(-0.0174295384816232,-0.236535169675584,
-1.15233649849688));
#70096=CARTESIAN_POINT('Ctrl Pts',(-0.0203274515066548,-0.236311389784029,
-1.15252984084061));
#70097=CARTESIAN_POINT('Ctrl Pts',(-0.0223922689776497,-0.236124681545236,
-1.15266632355011));
#70098=CARTESIAN_POINT('Ctrl Pts',(-0.0363692855367893,-0.234675828003325,
-1.15358314349622));
#70099=CARTESIAN_POINT('Ctrl Pts',(-0.048175032116428,-0.232539693511401,
-1.15432327526225));
#70100=CARTESIAN_POINT('Ctrl Pts',(-0.0699638891871704,-0.226865589767654,
-1.15570560675641));
#70101=CARTESIAN_POINT('Ctrl Pts',(-0.07996941314275,-0.223534844545659,
-1.15634735597856));
#70102=CARTESIAN_POINT('Ctrl Pts',(-0.0985374537651305,-0.215946938355736,
-1.15759586768057));
#70103=CARTESIAN_POINT('Ctrl Pts',(-0.107128782510009,-0.211816196857135,
-1.15819889367307));
#70104=CARTESIAN_POINT('Ctrl Pts',(-0.117378565001545,-0.206104677614221,
-1.15896417483642));
#70105=CARTESIAN_POINT('Ctrl Pts',(-0.119294071413432,-0.20500192594188,
-1.15910923653641));
#70106=CARTESIAN_POINT('Ctrl Pts',(-0.122321583501461,-0.203202195086298,
-1.15934194035894));
#70107=CARTESIAN_POINT('Ctrl Pts',(-0.123443730439871,-0.202522460916993,
-1.15942895632546));
#70108=CARTESIAN_POINT('Ctrl Pts',(-0.125557040455298,-0.201218245886004,
-1.15959431575223));
#70109=CARTESIAN_POINT('Ctrl Pts',(-0.126549332232269,-0.200595661249132,
-1.15967258771551));
#70110=CARTESIAN_POINT('Ctrl Pts',(-0.128792252297072,-0.199165140360875,
-1.15985096551648));
#70111=CARTESIAN_POINT('Ctrl Pts',(-0.130039956217819,-0.198352733778828,
-1.15995123546677));
#70112=CARTESIAN_POINT('Ctrl Pts',(-0.13383726454472,-0.195828997225761,
-1.16025965950965));
#70113=CARTESIAN_POINT('Ctrl Pts',(-0.136361265945692,-0.19407991432151,
-1.16046922264373));
#70114=CARTESIAN_POINT('Ctrl Pts',(-0.153745705485166,-0.181526304591085,
-1.16194554150995));
#70115=CARTESIAN_POINT('Ctrl Pts',(-0.167337942207479,-0.169077799770556,
-1.16327821337226));
#70116=CARTESIAN_POINT('Ctrl Pts',(-0.18174260520957,-0.15243004469822,
-1.16488600569931));
#70117=CARTESIAN_POINT('Ctrl Pts',(-0.184066024994794,-0.149616149185998,
-1.16515233782426));
#70118=CARTESIAN_POINT('Ctrl Pts',(-0.190381119026234,-0.141598069082342,
-1.16589454039798));
#70119=CARTESIAN_POINT('Ctrl Pts',(-0.194223494607145,-0.136279966921783,
-1.16636794035536));
#70120=CARTESIAN_POINT('Ctrl Pts',(-0.199864297572836,-0.127748599825389,
-1.16709162082814));
#70121=CARTESIAN_POINT('Ctrl Pts',(-0.201816713660103,-0.124641325233927,
-1.16734820356022));
#70122=CARTESIAN_POINT('Ctrl Pts',(-0.204267553770227,-0.120532114009814,
-1.16767732117223));
#70123=CARTESIAN_POINT('Ctrl Pts',(-0.204831992901538,-0.119570392818159,
-1.16775363527238));
#70124=CARTESIAN_POINT('Ctrl Pts',(-0.205742113495588,-0.117994322573419,
-1.16787749603055));
#70125=CARTESIAN_POINT('Ctrl Pts',(-0.206091868135685,-0.117382363865643,
-1.1679252955988));
#70126=CARTESIAN_POINT('Ctrl Pts',(-0.206769713668097,-0.116183981857287,
-1.16801831519171));
#70127=CARTESIAN_POINT('Ctrl Pts',(-0.207098047836004,-0.115597710748142,
-1.16806354969296));
#70128=CARTESIAN_POINT('Ctrl Pts',(-0.207827732597219,-0.114281703524437,
-1.16816449691621));
#70129=CARTESIAN_POINT('Ctrl Pts',(-0.208227744213148,-0.113551225395855,
-1.16822012554162));
#70130=CARTESIAN_POINT('Ctrl Pts',(-0.209608251784303,-0.110998394772349,
-1.16841318223844));
#70131=CARTESIAN_POINT('Ctrl Pts',(-0.210568772790058,-0.109165266905475,
-1.16854942543521));
#70132=CARTESIAN_POINT('Ctrl Pts',(-0.217030705839643,-0.0964301193337436,
-1.16948122206851));
#70133=CARTESIAN_POINT('Ctrl Pts',(-0.221707692869848,-0.0851285575530953,
-1.17023492700159));
#70134=CARTESIAN_POINT('Ctrl Pts',(-0.228886668415068,-0.0631085912129428,
-1.17165642729218));
#70135=CARTESIAN_POINT('Ctrl Pts',(-0.231555010257356,-0.0524792149611912,
-1.17232340992169));
#70136=CARTESIAN_POINT('Ctrl Pts',(-0.234522507227085,-0.035865684823955,
-1.173376367813));
#70137=CARTESIAN_POINT('Ctrl Pts',(-0.23534592502807,-0.0299906931523876,
-1.17375054319587));
#70138=CARTESIAN_POINT('Ctrl Pts',(-0.236364544315377,-0.0200144234771666,
-1.17439387417916));
#70139=CARTESIAN_POINT('Ctrl Pts',(-0.236675055693389,-0.0159276401333891,
-1.17465963204208));
#70140=CARTESIAN_POINT('Ctrl Pts',(-0.236962712114926,-0.0101701736989374,
-1.17503812091913));
#70141=CARTESIAN_POINT('Ctrl Pts',(-0.23702833711639,-0.00850450073222969,
-1.17514809805222));
#70142=CARTESIAN_POINT('Ctrl Pts',(-0.237110946904129,-0.00564051342665427,
-1.17533807811522));
#70143=CARTESIAN_POINT('Ctrl Pts',(-0.237136417925124,-0.00444249220207289,
-1.17541781319959));
#70144=CARTESIAN_POINT('Ctrl Pts',(-0.237167760966887,-0.00215140304656673,
-1.17557082767517));
#70145=CARTESIAN_POINT('Ctrl Pts',(-0.237175157069876,-0.0010583840107431,
-1.17564405729223));
#70146=CARTESIAN_POINT('Ctrl Pts',(-0.237174741680534,0.00178642760199683,
-1.17583527211774));
#70147=CARTESIAN_POINT('Ctrl Pts',(-0.23715507753422,0.00353812482777787,
-1.17595362460651));
#70148=CARTESIAN_POINT('Ctrl Pts',(-0.237011863470604,0.00995819632098395,
-1.17638972792835));
#70149=CARTESIAN_POINT('Ctrl Pts',(-0.236769853990665,0.0146225848959933,
-1.17671112571038));
#70150=CARTESIAN_POINT('Ctrl Pts',(-0.235812395804736,0.026364013917505,
-1.17753220430705));
#70151=CARTESIAN_POINT('Ctrl Pts',(-0.234916042727825,0.0334213101702695,
-1.17803691094854));
#70152=CARTESIAN_POINT('Ctrl Pts',(-0.230856515571357,0.0568889139292118,
-1.17974967845699));
#70153=CARTESIAN_POINT('Ctrl Pts',(-0.22627782844322,0.0730026233955595,
-1.18098663962895));
#70154=CARTESIAN_POINT('Ctrl Pts',(-0.217906823836924,0.0938158441443284,
-1.18259573249308));
#70155=CARTESIAN_POINT('Ctrl Pts',(-0.21557719070102,0.0990519230564529,
-1.18300110412899));
#70156=CARTESIAN_POINT('Ctrl Pts',(-0.212478364253266,0.105388225432735,
-1.1834881401991));
#70157=CARTESIAN_POINT('Ctrl Pts',(-0.211886766069377,0.106572660203199,
-1.18357902413048));
#70158=CARTESIAN_POINT('Ctrl Pts',(-0.210940642750093,0.108427862019017,
-1.18372105802144));
#70159=CARTESIAN_POINT('Ctrl Pts',(-0.21059277542902,0.109101966085748,
-1.18377260037059));
#70160=CARTESIAN_POINT('Ctrl Pts',(-0.209967279688984,0.110299925442415,
-1.18386406200718));
#70161=CARTESIAN_POINT('Ctrl Pts',(-0.209690921285973,0.110824409020092,
-1.18390405738454));
#70162=CARTESIAN_POINT('Ctrl Pts',(-0.209021449961354,0.112083487656867,
-1.18399996166854));
#70163=CARTESIAN_POINT('Ctrl Pts',(-0.208626429673238,0.112817053870883,
-1.18405574961404));
#70164=CARTESIAN_POINT('Ctrl Pts',(-0.207402921759457,0.115060746786211,
-1.18422616027394));
#70165=CARTESIAN_POINT('Ctrl Pts',(-0.206561820627709,0.116563982816697,
-1.18434002107219));
#70166=CARTESIAN_POINT('Ctrl Pts',(-0.198780679454096,0.130121854451292,
-1.1853653465641));
#70167=CARTESIAN_POINT('Ctrl Pts',(-0.190808059056369,0.141555124994127,
-1.18621936627424));
#70168=CARTESIAN_POINT('Ctrl Pts',(-0.170866808961038,0.16538090361281,
-1.18812422283224));
#70169=CARTESIAN_POINT('Ctrl Pts',(-0.158462159204998,0.17730191673118,
-1.18917161289272));
#70170=CARTESIAN_POINT('Ctrl Pts',(-0.142386233418689,0.189705219304556,
-1.19048406282894));
#70171=CARTESIAN_POINT('Ctrl Pts',(-0.139853423784967,0.19158008255297,
-1.19068951119054));
#70172=CARTESIAN_POINT('Ctrl Pts',(-0.136057571957042,0.194274496875286,
-1.19099590812578));
#70173=CARTESIAN_POINT('Ctrl Pts',(-0.134822804770519,0.195133426561145,
-1.191095347513));
#70174=CARTESIAN_POINT('Ctrl Pts',(-0.132610598882909,0.19664126203817,
-1.19127314290236));
#70175=CARTESIAN_POINT('Ctrl Pts',(-0.131636349362063,0.197294775181207,
-1.1913513211998));
#70176=CARTESIAN_POINT('Ctrl Pts',(-0.129569619459936,0.198658986384733,
-1.19151693059126));
#70177=CARTESIAN_POINT('Ctrl Pts',(-0.128476052404071,0.199367958808177,
-1.19160442289329));
#70178=CARTESIAN_POINT('Ctrl Pts',(-0.125546051942616,0.201233394959267,
-1.19183851259752));
#70179=CARTESIAN_POINT('Ctrl Pts',(-0.123699531701615,0.202373703122936,
-1.19198569916478));
#70180=CARTESIAN_POINT('Ctrl Pts',(-0.114201121407433,0.208060827212608,
-1.19274132021021));
#70181=CARTESIAN_POINT('Ctrl Pts',(-0.106314195626829,0.212199106191769,
-1.19336423610559));
#70182=CARTESIAN_POINT('Ctrl Pts',(-0.0878605932591958,0.220594383047642,
-1.19481131580663));
#70183=CARTESIAN_POINT('Ctrl Pts',(-0.0771822007688765,0.224553416472287,
-1.19564179880238));
#70184=CARTESIAN_POINT('Ctrl Pts',(-0.06297003361872,0.228688673782941,
-1.19672266195846));
#70185=CARTESIAN_POINT('Ctrl Pts',(-0.059657716118993,0.229575024998775,
-1.19697281403438));
#70186=CARTESIAN_POINT('Ctrl Pts',(-0.0515632186175443,0.231554029079316,
-1.19757855479759));
#70187=CARTESIAN_POINT('Ctrl Pts',(-0.0467648793695778,0.232570558798781,
-1.19793297986431));
#70188=CARTESIAN_POINT('Ctrl Pts',(-0.0419392699415209,0.233437525393353,
-1.19828290886153));
#70189=CARTESIAN_POINT('Ctrl Pts',(-0.041939274136423,0.233437524639699,
-1.21783461098805));
#70190=CARTESIAN_POINT('Ctrl Pts',(-0.0426432674237616,0.233311045542075,
-1.21778239868806));
#70191=CARTESIAN_POINT('Ctrl Pts',(-0.043346762008648,0.233181368630309,
-1.21773016760089));
#70192=CARTESIAN_POINT('Ctrl Pts',(-0.0540389257832951,0.231160385863027,
-1.21693553759598));
#70193=CARTESIAN_POINT('Ctrl Pts',(-0.0638968914046291,0.228631882994274,
-1.21619186825365));
#70194=CARTESIAN_POINT('Ctrl Pts',(-0.0766195564889107,0.224481099184353,
-1.21523749386044));
#70195=CARTESIAN_POINT('Ctrl Pts',(-0.0796560834308802,0.223421643636488,
-1.21501018080959));
#70196=CARTESIAN_POINT('Ctrl Pts',(-0.0847482635210627,0.221527938787716,
-1.21463080184728));
#70197=CARTESIAN_POINT('Ctrl Pts',(-0.0868154088882168,0.22072603268003,
-1.21447731157509));
#70198=CARTESIAN_POINT('Ctrl Pts',(-0.0897256243853002,0.219549863229728,
-1.21426225417374));
#70199=CARTESIAN_POINT('Ctrl Pts',(-0.0905781497778032,0.219199518634965,
-1.21419938160906));
#70200=CARTESIAN_POINT('Ctrl Pts',(-0.0920429676698517,0.218587547708031,
-1.2140915989717));
#70201=CARTESIAN_POINT('Ctrl Pts',(-0.0926562345163415,0.218328299040453,
-1.21404654933767));
#70202=CARTESIAN_POINT('Ctrl Pts',(-0.0939410738838145,0.217778765019048,
-1.21395233386869));
#70203=CARTESIAN_POINT('Ctrl Pts',(-0.0946124026783115,0.217487951739309,
-1.21390320021296));
#70204=CARTESIAN_POINT('Ctrl Pts',(-0.0964152105135642,0.21669706521441,
-1.21377148013796));
#70205=CARTESIAN_POINT('Ctrl Pts',(-0.0975441596143591,0.216191230120239,
-1.21368923432154));
#70206=CARTESIAN_POINT('Ctrl Pts',(-0.102719891697156,0.213823402332313,
-1.21331304579725));
#70207=CARTESIAN_POINT('Ctrl Pts',(-0.106717958595642,0.21185633567699,
-1.21302491633419));
#70208=CARTESIAN_POINT('Ctrl Pts',(-0.130637611581025,0.199238625398129,
-1.21130197056097));
#70209=CARTESIAN_POINT('Ctrl Pts',(-0.149009874234426,0.185899088748642,
-1.20997161250906));
#70210=CARTESIAN_POINT('Ctrl Pts',(-0.168478997329588,0.166995373724913,
-1.20826084139175));
#70211=CARTESIAN_POINT('Ctrl Pts',(-0.171647185520011,0.163737189538371,
-1.20797143840478));
#70212=CARTESIAN_POINT('Ctrl Pts',(-0.176989964973071,0.157917076966593,
-1.20746164681532));
#70213=CARTESIAN_POINT('Ctrl Pts',(-0.179207365019452,0.155396169167168,
-1.2072430350147));
#70214=CARTESIAN_POINT('Ctrl Pts',(-0.1823639492274,0.15165008381701,-1.20692079377868));
#70215=CARTESIAN_POINT('Ctrl Pts',(-0.183345928721492,0.150461384189584,
-1.20681891383569));
#70216=CARTESIAN_POINT('Ctrl Pts',(-0.185057349953819,0.148348052365386,
-1.20663838922153));
#70217=CARTESIAN_POINT('Ctrl Pts',(-0.185791632555776,0.147427394330266,
-1.20655994285945));
#70218=CARTESIAN_POINT('Ctrl Pts',(-0.18731183263042,0.145491942666614,
-1.2063954177499));
#70219=CARTESIAN_POINT('Ctrl Pts',(-0.188096427489744,0.144476163700002,
-1.20630928996589));
#70220=CARTESIAN_POINT('Ctrl Pts',(-0.190131143382502,0.141797241445922,
-1.20608268517788));
#70221=CARTESIAN_POINT('Ctrl Pts',(-0.191367668819423,0.140123960173734,
-1.20594168359108));
#70222=CARTESIAN_POINT('Ctrl Pts',(-0.196614008545141,0.132825568046982,
-1.20532880857199));
#70223=CARTESIAN_POINT('Ctrl Pts',(-0.200398658133802,0.127043539287908,
-1.20484852618026));
#70224=CARTESIAN_POINT('Ctrl Pts',(-0.212160122662664,0.107238754336975,
-1.20321973371885));
#70225=CARTESIAN_POINT('Ctrl Pts',(-0.218958395352845,0.09256984386528,
-1.20203580068697));
#70226=CARTESIAN_POINT('Ctrl Pts',(-0.227563828599233,0.0676178135817661,
-1.20011383446844));
#70227=CARTESIAN_POINT('Ctrl Pts',(-0.230278583307003,0.0576999922608403,
-1.19937301128378));
#70228=CARTESIAN_POINT('Ctrl Pts',(-0.232635944227891,0.0462021790844658,
-1.19856106024312));
#70229=CARTESIAN_POINT('Ctrl Pts',(-0.232916709799689,0.0447652819295154,
-1.19846042002002));
#70230=CARTESIAN_POINT('Ctrl Pts',(-0.233326763068729,0.0425583323512279,
-1.19830721017047));
#70231=CARTESIAN_POINT('Ctrl Pts',(-0.233465577801123,0.0417901189632514,
-1.19825413225684));
#70232=CARTESIAN_POINT('Ctrl Pts',(-0.233714030452848,0.0403752734776626,
-1.19815685866873));
#70233=CARTESIAN_POINT('Ctrl Pts',(-0.233824779758888,0.0397288702221894,
-1.19811260362287));
#70234=CARTESIAN_POINT('Ctrl Pts',(-0.234070929117119,0.0382554953722119,
-1.19801214958318));
#70235=CARTESIAN_POINT('Ctrl Pts',(-0.234204629049285,0.0374282589726527,
-1.19795604649148));
#70236=CARTESIAN_POINT('Ctrl Pts',(-0.234543053413201,0.0352614930589668,
-1.19780983328912));
#70237=CARTESIAN_POINT('Ctrl Pts',(-0.234740690846305,0.0339208647910625,
-1.19772010318464));
#70238=CARTESIAN_POINT('Ctrl Pts',(-0.236414371006712,0.0218518181606137,
-1.19691830900986));
#70239=CARTESIAN_POINT('Ctrl Pts',(-0.237165692648452,0.0110342417309567,
-1.19624196860633));
#70240=CARTESIAN_POINT('Ctrl Pts',(-0.237189966526827,-0.0174801366085886,
-1.19448383101853));
#70241=CARTESIAN_POINT('Ctrl Pts',(-0.235227740014875,-0.0351072123251257,
-1.19341787834779));
#70242=CARTESIAN_POINT('Ctrl Pts',(-0.230186434309013,-0.0573828222203118,
-1.19196437274814));
#70243=CARTESIAN_POINT('Ctrl Pts',(-0.228884237018761,-0.0623745352904542,
-1.19163189578001));
#70244=CARTESIAN_POINT('Ctrl Pts',(-0.226888867572798,-0.0691153367603384,
-1.19117160025476));
#70245=CARTESIAN_POINT('Ctrl Pts',(-0.226336055440587,-0.0709047084328291,
-1.19104831278622));
#70246=CARTESIAN_POINT('Ctrl Pts',(-0.225420383715599,-0.0737487263186357,
-1.19085051343898));
#70247=CARTESIAN_POINT('Ctrl Pts',(-0.225071167766121,-0.0748077094700161,
-1.19077645013998));
#70248=CARTESIAN_POINT('Ctrl Pts',(-0.224336316702724,-0.0769843849543035,
-1.19062334725718));
#70249=CARTESIAN_POINT('Ctrl Pts',(-0.223949766107451,-0.0781017329610288,
-1.19054427924332));
#70250=CARTESIAN_POINT('Ctrl Pts',(-0.223029129709321,-0.0806998499204871,
-1.19035929009358));
#70251=CARTESIAN_POINT('Ctrl Pts',(-0.222488629368415,-0.0821782700574747,
-1.19025315852848));
#70252=CARTESIAN_POINT('Ctrl Pts',(-0.220685338120716,-0.0869625506972465,
-1.18990682228929));
#70253=CARTESIAN_POINT('Ctrl Pts',(-0.219363319668876,-0.0902454171498826,
-1.18966465743708));
#70254=CARTESIAN_POINT('Ctrl Pts',(-0.216048375434738,-0.097973478762779,
-1.18908345578343));
#70255=CARTESIAN_POINT('Ctrl Pts',(-0.213991036099672,-0.102389129468412,
-1.18874239266833));
#70256=CARTESIAN_POINT('Ctrl Pts',(-0.20514865303143,-0.119934987770485,
-1.18735067571285));
#70257=CARTESIAN_POINT('Ctrl Pts',(-0.197279653408148,-0.132480269158027,
-1.18626837018449));
#70258=CARTESIAN_POINT('Ctrl Pts',(-0.181497998076469,-0.153086424613433,
-1.18437557275629));
#70259=CARTESIAN_POINT('Ctrl Pts',(-0.174080126472723,-0.161471810516364,
-1.18356618472631));
#70260=CARTESIAN_POINT('Ctrl Pts',(-0.165129842716036,-0.170252615626823,
-1.18269830427765));
#70261=CARTESIAN_POINT('Ctrl Pts',(-0.164154072812613,-0.171193629191316,
-1.18260502020909));
#70262=CARTESIAN_POINT('Ctrl Pts',(-0.1625620289862,-0.172702836549947,
-1.18245503838124));
#70263=CARTESIAN_POINT('Ctrl Pts',(-0.161950733553993,-0.173276204298726,
-1.18239796970843));
#70264=CARTESIAN_POINT('Ctrl Pts',(-0.160855683220197,-0.17429245513326,
-1.18229668173844));
#70265=CARTESIAN_POINT('Ctrl Pts',(-0.160373118015634,-0.174736584015536,
-1.18225236979393));
#70266=CARTESIAN_POINT('Ctrl Pts',(-0.159312196976313,-0.17570490528099,
-1.1821556574077));
#70267=CARTESIAN_POINT('Ctrl Pts',(-0.158733092249554,-0.176228247775858,
-1.18210332002352));
#70268=CARTESIAN_POINT('Ctrl Pts',(-0.157060789017248,-0.177724592910838,
-1.18195344369183));
#70269=CARTESIAN_POINT('Ctrl Pts',(-0.155961131073359,-0.178690369727646,
-1.18185642363749));
#70270=CARTESIAN_POINT('Ctrl Pts',(-0.147092081431071,-0.186335380591913,
-1.18108543255655));
#70271=CARTESIAN_POINT('Ctrl Pts',(-0.138905201989436,-0.192515856226519,
-1.18044342693715));
#70272=CARTESIAN_POINT('Ctrl Pts',(-0.116923368509795,-0.206975663473038,
-1.1788180998305));
#70273=CARTESIAN_POINT('Ctrl Pts',(-0.102642028157704,-0.214416897293547,
-1.17784964424824));
#70274=CARTESIAN_POINT('Ctrl Pts',(-0.0812338229270205,-0.222938909942981,
-1.1763990717586));
#70275=CARTESIAN_POINT('Ctrl Pts',(-0.0746391563416337,-0.22523248776701,
-1.17595288723864));
#70276=CARTESIAN_POINT('Ctrl Pts',(-0.0659518223529203,-0.227830424702331,
-1.17536070631811));
#70277=CARTESIAN_POINT('Ctrl Pts',(-0.0639424623218083,-0.228402509496634,
-1.17522344837878));
#70278=CARTESIAN_POINT('Ctrl Pts',(-0.0606850630214332,-0.229283571062877,
-1.17500035064011));
#70279=CARTESIAN_POINT('Ctrl Pts',(-0.0594415808420452,-0.229609083421537,
-1.17491504830998));
#70280=CARTESIAN_POINT('Ctrl Pts',(-0.0570544481608036,-0.230213283856152,
-1.17475100167034));
#70281=CARTESIAN_POINT('Ctrl Pts',(-0.0559112455733474,-0.230493597852465,
-1.17467231257606));
#70282=CARTESIAN_POINT('Ctrl Pts',(-0.0532697426525975,-0.23112048825232,
-1.1744901772587));
#70283=CARTESIAN_POINT('Ctrl Pts',(-0.0517700772258659,-0.231461021518108,
-1.17438654037031));
#70284=CARTESIAN_POINT('Ctrl Pts',(-0.047007957685412,-0.232493774222229,
-1.17405665198162));
#70285=CARTESIAN_POINT('Ctrl Pts',(-0.0437342859624637,-0.2331317511562,
-1.17382869066242));
#70286=CARTESIAN_POINT('Ctrl Pts',(-0.0360096315498282,-0.234468718296675,
-1.17328775003801));
#70287=CARTESIAN_POINT('Ctrl Pts',(-0.0315501541622061,-0.235110307354584,
-1.17297310204474));
#70288=CARTESIAN_POINT('Ctrl Pts',(-0.00519185329237518,-0.238139110969328,
-1.17109954244191));
#70289=CARTESIAN_POINT('Ctrl Pts',(0.0169309740180664,-0.237592714306224,
-1.16945751408562));
#70290=CARTESIAN_POINT('Ctrl Pts',(0.0435897094744356,-0.233188544262195,
-1.16752728814484));
#70291=CARTESIAN_POINT('Ctrl Pts',(0.0484942525374433,-0.2322181643712,
-1.16717491708163));
#70292=CARTESIAN_POINT('Ctrl Pts',(0.0546185946834486,-0.230803911213174,
-1.16674127149684));
#70293=CARTESIAN_POINT('Ctrl Pts',(0.0558699961668047,-0.230504186581823,
-1.16665300260769));
#70294=CARTESIAN_POINT('Ctrl Pts',(0.0578395936612615,-0.230015463309025,
-1.16651467641907));
#70295=CARTESIAN_POINT('Ctrl Pts',(0.0585594250101764,-0.229833256377454,
-1.16646424940534));
#70296=CARTESIAN_POINT('Ctrl Pts',(0.0599196974655453,-0.229482132515216,
-1.1663692133818));
#70297=CARTESIAN_POINT('Ctrl Pts',(0.0605602827239637,-0.229313914657534,
-1.16632456850734));
#70298=CARTESIAN_POINT('Ctrl Pts',(0.062068282962792,-0.228911153592259,
-1.1662197164826));
#70299=CARTESIAN_POINT('Ctrl Pts',(0.0629350812841534,-0.22867436148042,
-1.16615963890224));
#70300=CARTESIAN_POINT('Ctrl Pts',(0.0658038398927074,-0.227873126079228,
-1.16596137666121));
#70301=CARTESIAN_POINT('Ctrl Pts',(0.06779978693299,-0.227287255592521,
-1.16582435903735));
#70302=CARTESIAN_POINT('Ctrl Pts',(0.0792768821923279,-0.223753733212192,
-1.16504044166496));
#70303=CARTESIAN_POINT('Ctrl Pts',(0.0885742753545106,-0.220238964085418,
-1.16442088886412));
#70304=CARTESIAN_POINT('Ctrl Pts',(0.113709994481223,-0.208886396498186,
-1.16272027400538));
#70305=CARTESIAN_POINT('Ctrl Pts',(0.128932892464018,-0.199849368037075,
-1.16165628474119));
#70306=CARTESIAN_POINT('Ctrl Pts',(0.147143878956586,-0.186084608770122,
-1.1602038195267));
#70307=CARTESIAN_POINT('Ctrl Pts',(0.151171793568941,-0.182827474081539,
-1.15987003806815));
#70308=CARTESIAN_POINT('Ctrl Pts',(0.156514942831373,-0.178209433620596,
-1.15940768941758));
#70309=CARTESIAN_POINT('Ctrl Pts',(0.157925467869987,-0.176960661785372,
-1.15928368714886));
#70310=CARTESIAN_POINT('Ctrl Pts',(0.160148520271148,-0.174944791761097,
-1.15908503158904));
#70311=CARTESIAN_POINT('Ctrl Pts',(0.160970781155501,-0.174188507803499,
-1.15901083412621));
#70312=CARTESIAN_POINT('Ctrl Pts',(0.162651414624463,-0.172620663080795,
-1.15885767206547));
#70313=CARTESIAN_POINT('Ctrl Pts',(0.163509127065789,-0.171808443566612,
-1.15877868046286));
#70314=CARTESIAN_POINT('Ctrl Pts',(0.165490503833879,-0.169903883189675,
-1.15859424751607));
#70315=CARTESIAN_POINT('Ctrl Pts',(0.166609469420922,-0.168806756014027,
-1.15848859959192));
#70316=CARTESIAN_POINT('Ctrl Pts',(0.170191242252126,-0.165224581338649,
-1.15814549610098));
#70317=CARTESIAN_POINT('Ctrl Pts',(0.172609858264452,-0.162696207004697,
-1.157906130965));
#70318=CARTESIAN_POINT('Ctrl Pts',(0.178210440126726,-0.15657597942922,
-1.15733292593698));
#70319=CARTESIAN_POINT('Ctrl Pts',(0.181340973279195,-0.15293934826554,
-1.15699713391003));
#70320=CARTESIAN_POINT('Ctrl Pts',(0.193377046030653,-0.138068027708613,
-1.1556427945762));
#70321=CARTESIAN_POINT('Ctrl Pts',(0.201365622090606,-0.126131936532784,
-1.15459448459287));
#70322=CARTESIAN_POINT('Ctrl Pts',(0.213851484562006,-0.103235351280445,
-1.15269140409647));
#70323=CARTESIAN_POINT('Ctrl Pts',(0.218702504131413,-0.0925163502315752,
-1.15183913573745));
#70324=CARTESIAN_POINT('Ctrl Pts',(0.223206428849908,-0.0802042299955998,
-1.15093162811337));
#70325=CARTESIAN_POINT('Ctrl Pts',(0.223662451455706,-0.078923611252432,
-1.15083807838557));
#70326=CARTESIAN_POINT('Ctrl Pts',(0.224382169397844,-0.0768461252722291,
-1.15068775520898));
#70327=CARTESIAN_POINT('Ctrl Pts',(0.224652681774047,-0.0760516767686259,
-1.15063060818971));
#70328=CARTESIAN_POINT('Ctrl Pts',(0.225127096139052,-0.074633782038733,
-1.15052923654061));
#70329=CARTESIAN_POINT('Ctrl Pts',(0.225332634575074,-0.0740109091146725,
-1.15048491862404));
#70330=CARTESIAN_POINT('Ctrl Pts',(0.225776836108271,-0.0726457759233576,
-1.1503882580277));
#70331=CARTESIAN_POINT('Ctrl Pts',(0.226014424854859,-0.0719031868833949,
-1.1503359778874));
#70332=CARTESIAN_POINT('Ctrl Pts',(0.226686191203706,-0.0697673345178731,
-1.15018643258901));
#70333=CARTESIAN_POINT('Ctrl Pts',(0.227111186799947,-0.0683711879622448,
-1.15008968277201));
#70334=CARTESIAN_POINT('Ctrl Pts',(0.230362579922951,-0.0573251259809278,
-1.14933145496211));
#70335=CARTESIAN_POINT('Ctrl Pts',(0.232585962626882,-0.047506960406693,
-1.14870075649617));
#70336=CARTESIAN_POINT('Ctrl Pts',(0.236647272772651,-0.0221963316549909,
-1.14711626951225));
#70337=CARTESIAN_POINT('Ctrl Pts',(0.237593974859879,-0.00661129926719322,
-1.14617690937497));
#70338=CARTESIAN_POINT('Ctrl Pts',(0.236720771513213,0.0165016644178685,
-1.14472521323594));
#70339=CARTESIAN_POINT('Ctrl Pts',(0.236075278998369,0.0240306782890839,
-1.14424354496226));
#70340=CARTESIAN_POINT('Ctrl Pts',(0.234786703244166,0.0336420559040256,
-1.14361062633756));
#70341=CARTESIAN_POINT('Ctrl Pts',(0.234472772863252,0.0357645387869451,
-1.14346973376627));
#70342=CARTESIAN_POINT('Ctrl Pts',(0.233922836654266,0.0391633880952803,
-1.14324217168667));
#70343=CARTESIAN_POINT('Ctrl Pts',(0.233705068642686,0.0404426167860829,
-1.14315608033256));
#70344=CARTESIAN_POINT('Ctrl Pts',(0.233270327312588,0.0428755527529102,
-1.14299146956674));
#70345=CARTESIAN_POINT('Ctrl Pts',(0.233055263638428,0.04402956544546,-1.14291301311287));
#70346=CARTESIAN_POINT('Ctrl Pts',(0.23254337001669,0.0466674578513854,
-1.14273278763022));
#70347=CARTESIAN_POINT('Ctrl Pts',(0.232240889969586,0.0481501755166029,
-1.14263084121828));
#70348=CARTESIAN_POINT('Ctrl Pts',(0.231254337733099,0.0527604111687545,
-1.14231179123146));
#70349=CARTESIAN_POINT('Ctrl Pts',(0.230521141724206,0.0558769288640855,
-1.14209313318396));
#70350=CARTESIAN_POINT('Ctrl Pts',(0.228663209140359,0.0631138178054533,
-1.14157815574417));
#70351=CARTESIAN_POINT('Ctrl Pts',(0.227489837085896,0.0672204381811554,
-1.14128037762379));
#70352=CARTESIAN_POINT('Ctrl Pts',(0.22273413316225,0.0823098752403299,
-1.14016545633391));
#70353=CARTESIAN_POINT('Ctrl Pts',(0.218462121316603,0.0930572823219848,
-1.13932901333487));
#70354=CARTESIAN_POINT('Ctrl Pts',(0.207026492703291,0.11664989073627,-1.13741566163372));
#70355=CARTESIAN_POINT('Ctrl Pts',(0.199416796277902,0.129229182400962,
-1.13633821743566));
#70356=CARTESIAN_POINT('Ctrl Pts',(0.189474888511497,0.142672504028754,
-1.13517284077083));
#70357=CARTESIAN_POINT('Ctrl Pts',(0.188235529351324,0.144303717839589,
-1.1350312210815));
#70358=CARTESIAN_POINT('Ctrl Pts',(0.186480133724057,0.146553020090981,
-1.13483587175918));
#70359=CARTESIAN_POINT('Ctrl Pts',(0.18598189411616,0.147184792285298,-1.1347809955183));
#70360=CARTESIAN_POINT('Ctrl Pts',(0.185066232169903,0.14833378594118,-1.13468119793736));
#70361=CARTESIAN_POINT('Ctrl Pts',(0.184649832438878,0.148851811429472,
-1.13463620615016));
#70362=CARTESIAN_POINT('Ctrl Pts',(0.183779803802982,0.14992490848241,-1.13454301994349));
#70363=CARTESIAN_POINT('Ctrl Pts',(0.183325829322084,0.150479682373755,
-1.13449485085888));
#70364=CARTESIAN_POINT('Ctrl Pts',(0.182124172832322,0.151934642565317,
-1.13436851335886));
#70365=CARTESIAN_POINT('Ctrl Pts',(0.181372320531353,0.152831382336588,
-1.1342906388956));
#70366=CARTESIAN_POINT('Ctrl Pts',(0.177874875446163,0.156940649475194,
-1.13393354494358));
#70367=CARTESIAN_POINT('Ctrl Pts',(0.175050181434453,0.160085221321697,
-1.13365960265962));
#70368=CARTESIAN_POINT('Ctrl Pts',(0.166508432087525,0.169097630576571,
-1.13286652560206));
#70369=CARTESIAN_POINT('Ctrl Pts',(0.16056949764631,0.174747027053532,-1.13235885618539));
#70370=CARTESIAN_POINT('Ctrl Pts',(0.139154754956289,0.193102167292089,
-1.13062390588213));
#70371=CARTESIAN_POINT('Ctrl Pts',(0.122374374625392,0.204149272007522,
-1.12941495888262));
#70372=CARTESIAN_POINT('Ctrl Pts',(0.101844657950847,0.214214351954104,
-1.12793364640446));
#70373=CARTESIAN_POINT('Ctrl Pts',(0.0992601730673875,0.215424092985487,
-1.12774730711218));
#70374=CARTESIAN_POINT('Ctrl Pts',(0.0953166213266252,0.217183951896363,
-1.12746287091724));
#70375=CARTESIAN_POINT('Ctrl Pts',(0.093973185100963,0.217768610185506,
-1.12736595496512));
#70376=CARTESIAN_POINT('Ctrl Pts',(0.0915484904539209,0.218797213264977,
-1.12719096180378));
#70377=CARTESIAN_POINT('Ctrl Pts',(0.0904691954517588,0.219245686906772,
-1.12711304144637));
#70378=CARTESIAN_POINT('Ctrl Pts',(0.0881584162751297,0.220185904544184,
-1.12694613523589));
#70379=CARTESIAN_POINT('Ctrl Pts',(0.0869260391746348,0.220675332806878,
-1.1268570743614));
#70380=CARTESIAN_POINT('Ctrl Pts',(0.0835670349066219,0.221976830267272,
-1.12661416530842));
#70381=CARTESIAN_POINT('Ctrl Pts',(0.0814327624010879,0.222768640243523,
-1.12645964729178));
#70382=CARTESIAN_POINT('Ctrl Pts',(0.069161609172963,0.227121303014167,
-1.12556995828185));
#70383=CARTESIAN_POINT('Ctrl Pts',(0.0588048803807109,0.230020304572861,
-1.12481327104394));
#70384=CARTESIAN_POINT('Ctrl Pts',(0.0318700692891486,0.235621532120924,
-1.122834600259));
#70385=CARTESIAN_POINT('Ctrl Pts',(0.0151368066056107,0.237284733431819,
-1.12159275197029));
#70386=CARTESIAN_POINT('Ctrl Pts',(-0.00727937266991831,0.237130538190622,
-1.11998554124484));
#70387=CARTESIAN_POINT('Ctrl Pts',(-0.0129246656213208,0.236889945144055,
-1.11958601924403));
#70388=CARTESIAN_POINT('Ctrl Pts',(-0.01987106672925,0.236344790856433,
-1.11910494127196));
#70389=CARTESIAN_POINT('Ctrl Pts',(-0.021184827551682,0.236230655800076,
-1.11901442370359));
#70390=CARTESIAN_POINT('Ctrl Pts',(-0.0232513904948218,0.236033740842036,
-1.11887284609843));
#70391=CARTESIAN_POINT('Ctrl Pts',(-0.0240048407047941,0.235958304874383,
-1.1188213974902));
#70392=CARTESIAN_POINT('Ctrl Pts',(-0.0253475052931209,0.235817378555635,
-1.11873003233602));
#70393=CARTESIAN_POINT('Ctrl Pts',(-0.0259368354468668,0.235753287637763,
-1.11869004040564));
#70394=CARTESIAN_POINT('Ctrl Pts',(-0.0273551085037183,0.235593664798319,
-1.11859405626479));
#70395=CARTESIAN_POINT('Ctrl Pts',(-0.0281837947362655,0.235495967315535,
-1.11853818576082));
#70396=CARTESIAN_POINT('Ctrl Pts',(-0.0307287808913199,0.235182301381307,
-1.11836720624933));
#70397=CARTESIAN_POINT('Ctrl Pts',(-0.032443293570044,0.234951922723352,
-1.11825286679294));
#70398=CARTESIAN_POINT('Ctrl Pts',(-0.0367572909630109,0.234324126990049,
-1.11796695612443));
#70399=CARTESIAN_POINT('Ctrl Pts',(-0.0393523414674697,0.233902291759656,
-1.11779660855508));
#70400=CARTESIAN_POINT('Ctrl Pts',(-0.0419392769977373,0.233437524125636,
-1.11762795217595));
#70401=CARTESIAN_POINT('Origin',(0.,0.,-2.1456589891905));
#70402=CARTESIAN_POINT('',(-0.0419392532630312,0.233437528389801,-0.998011590250681));
#70403=CARTESIAN_POINT('',(-0.0419392742985056,0.233437524610579,-1.01798096863704));
#70404=CARTESIAN_POINT('',(-0.0419392741328076,0.233437524640348,-2.1456589891905));
#70405=CARTESIAN_POINT('',(-0.237174906576387,-0.000216561049440317,-1.0759596619759));
#70406=CARTESIAN_POINT('Ctrl Pts',(-0.0419392532630312,0.233437528389801,
-0.998011590250681));
#70407=CARTESIAN_POINT('Ctrl Pts',(-0.0328874669837367,0.235063767152132,
-0.998582398995608));
#70408=CARTESIAN_POINT('Ctrl Pts',(-0.0237399095455045,0.236163749446927,
-0.999162446510492));
#70409=CARTESIAN_POINT('Ctrl Pts',(-0.0117150820866228,0.236902426277311,
-0.999943121146646));
#70410=CARTESIAN_POINT('Ctrl Pts',(-0.00888529964478573,0.237025427029939,
-1.00012810595657));
#70411=CARTESIAN_POINT('Ctrl Pts',(-0.00459355961697687,0.237135012956913,
-1.00041089930749));
#70412=CARTESIAN_POINT('Ctrl Pts',(-0.00313274574200432,0.237158809457264,
-1.00050754806663));
#70413=CARTESIAN_POINT('Ctrl Pts',(-0.000503092558483613,0.237177346185061,
-1.00068227607908));
#70414=CARTESIAN_POINT('Ctrl Pts',(0.000665673775309822,0.237176945422453,
-1.00076020087131));
#70415=CARTESIAN_POINT('Ctrl Pts',(0.0031639062113637,0.237157622880442,
-1.00092735495426));
#70416=CARTESIAN_POINT('Ctrl Pts',(0.00449330666895667,0.237136160175794,
-1.0010166611308));
#70417=CARTESIAN_POINT('Ctrl Pts',(0.00811331635866864,0.237047265398379,
-1.00126085386602));
#70418=CARTESIAN_POINT('Ctrl Pts',(0.0104031907509557,0.236957812520127,
-1.00141642198706));
#70419=CARTESIAN_POINT('Ctrl Pts',(0.0237280251643335,0.236243771607516,
-1.00232837531452));
#70420=CARTESIAN_POINT('Ctrl Pts',(0.0347081994711379,0.23488170362907,
-1.00310759731519));
#70421=CARTESIAN_POINT('Ctrl Pts',(0.0588262379710849,0.230161696597181,
-1.00487713424754));
#70422=CARTESIAN_POINT('Ctrl Pts',(0.0718536144925931,0.226433128616646,
-1.0058730389529));
#70423=CARTESIAN_POINT('Ctrl Pts',(0.0879627006156639,0.220291504277364,
-1.00712273880018));
#70424=CARTESIAN_POINT('Ctrl Pts',(0.0914027502905743,0.218886552590294,
-1.00739058174466));
#70425=CARTESIAN_POINT('Ctrl Pts',(0.0993298084682449,0.215429570417215,
-1.00800811535297));
#70426=CARTESIAN_POINT('Ctrl Pts',(0.103788904671347,0.213317092807266,
-1.00835574730141));
#70427=CARTESIAN_POINT('Ctrl Pts',(0.109317569090208,0.210483457707194,
-1.00878430518142));
#70428=CARTESIAN_POINT('Ctrl Pts',(0.11045121507942,0.209890795776027,-1.00887204592977));
#70429=CARTESIAN_POINT('Ctrl Pts',(0.112233930905165,0.208940361061796,
-1.00900974461437));
#70430=CARTESIAN_POINT('Ctrl Pts',(0.112886193875657,0.208588678977381,
-1.00906006667923));
#70431=CARTESIAN_POINT('Ctrl Pts',(0.114118953759951,0.207916532909453,
-1.00915504600153));
#70432=CARTESIAN_POINT('Ctrl Pts',(0.114699751484382,0.207596693819212,
-1.00919973801262));
#70433=CARTESIAN_POINT('Ctrl Pts',(0.116067848969686,0.20683580292801,-1.00930489253789));
#70434=CARTESIAN_POINT('Ctrl Pts',(0.116853983652413,0.206392687633389,
-1.00936522341963));
#70435=CARTESIAN_POINT('Ctrl Pts',(0.119462227481973,0.204902836565376,
-1.00956514516226));
#70436=CARTESIAN_POINT('Ctrl Pts',(0.121273014794954,0.203836338420617,
-1.00970354236594));
#70437=CARTESIAN_POINT('Ctrl Pts',(0.131743308685783,0.19748072948478,-1.01050288285373));
#70438=CARTESIAN_POINT('Ctrl Pts',(0.140071413345457,0.191663731318453,
-1.01113529800079));
#70439=CARTESIAN_POINT('Ctrl Pts',(0.162298854787571,0.173913233054972,
-1.01288810378387));
#70440=CARTESIAN_POINT('Ctrl Pts',(0.175225468907639,0.160881092991682,
-1.01399132006797));
#70441=CARTESIAN_POINT('Ctrl Pts',(0.189314454932511,0.142941964745945,
-1.01544937550471));
#70442=CARTESIAN_POINT('Ctrl Pts',(0.192001204241583,0.139312244378768,
-1.01574136463577));
#70443=CARTESIAN_POINT('Ctrl Pts',(0.195600069986374,0.134148276139748,
-1.0161539904859));
#70444=CARTESIAN_POINT('Ctrl Pts',(0.196601057594817,0.132676943118815,
-1.01627124952305));
#70445=CARTESIAN_POINT('Ctrl Pts',(0.198192752576374,0.130279772499474,
-1.01646187371813));
#70446=CARTESIAN_POINT('Ctrl Pts',(0.198793765030266,0.129360833377872,
-1.01653484985654));
#70447=CARTESIAN_POINT('Ctrl Pts',(0.200034976506164,0.127433961445204,
-1.01668768413772));
#70448=CARTESIAN_POINT('Ctrl Pts',(0.200673986662028,0.126425303410582,
-1.01676758368978));
#70449=CARTESIAN_POINT('Ctrl Pts',(0.202174203059067,0.124017225489281,
-1.01695811367661));
#70450=CARTESIAN_POINT('Ctrl Pts',(0.203028526391919,0.122613611947533,
-1.01706899272458));
#70451=CARTESIAN_POINT('Ctrl Pts',(0.205885862603953,0.117807392083154,
-1.01744813865333));
#70452=CARTESIAN_POINT('Ctrl Pts',(0.20781837154148,0.114363854616889,-1.0177189180925));
#70453=CARTESIAN_POINT('Ctrl Pts',(0.219716648575738,0.0918640554198085,
-1.01948368449075));
#70454=CARTESIAN_POINT('Ctrl Pts',(0.227135822621361,0.0715777870506341,
-1.0210676646075));
#70455=CARTESIAN_POINT('Ctrl Pts',(0.233598132377264,0.0419700644412308,
-1.02326742557111));
#70456=CARTESIAN_POINT('Ctrl Pts',(0.23499585202499,0.0332649769896782,
-1.02389934409235));
#70457=CARTESIAN_POINT('Ctrl Pts',(0.236043393156607,0.023178974833921,
-1.02460094339431));
#70458=CARTESIAN_POINT('Ctrl Pts',(0.236169624155886,0.0218553690253736,
-1.02469240976647));
#70459=CARTESIAN_POINT('Ctrl Pts',(0.236356611385386,0.0197033648891967,
-1.02484006372003));
#70460=CARTESIAN_POINT('Ctrl Pts',(0.236424156608383,0.0188756074999746,
-1.02489660416898));
#70461=CARTESIAN_POINT('Ctrl Pts',(0.236537241350122,0.0173937891702756,
-1.02499734619934));
#70462=CARTESIAN_POINT('Ctrl Pts',(0.236584418191094,0.0167398790147472,
-1.02504163600444));
#70463=CARTESIAN_POINT('Ctrl Pts',(0.236682271258211,0.0153004152245222,
-1.02513876471091));
#70464=CARTESIAN_POINT('Ctrl Pts',(0.236731748733401,0.0145148000579126,
-1.02519153676507));
#70465=CARTESIAN_POINT('Ctrl Pts',(0.236863814288344,0.0122371202018512,
-1.02534388401045));
#70466=CARTESIAN_POINT('Ctrl Pts',(0.236936215633787,0.0107444699588521,
-1.02544291363546));
#70467=CARTESIAN_POINT('Ctrl Pts',(0.237469744551497,-0.0029233337106176,
-1.02634311689417));
#70468=CARTESIAN_POINT('Ctrl Pts',(0.237006223732121,-0.0151182247785406,
-1.02709898877298));
#70469=CARTESIAN_POINT('Ctrl Pts',(0.233359895024032,-0.0466738801794996,
-1.02905165307747));
#70470=CARTESIAN_POINT('Ctrl Pts',(0.228713478205454,-0.0657674262803102,
-1.03023622671175));
#70471=CARTESIAN_POINT('Ctrl Pts',(0.220743706638506,-0.0867908284242931,
-1.03169214632821));
#70472=CARTESIAN_POINT('Ctrl Pts',(0.219663356922596,-0.0894898896017913,
-1.03188192031583));
#70473=CARTESIAN_POINT('Ctrl Pts',(0.217959888565634,-0.0935288615691752,
-1.03217058702827));
#70474=CARTESIAN_POINT('Ctrl Pts',(0.217373387079859,-0.0948839891306491,
-1.03226824490129));
#70475=CARTESIAN_POINT('Ctrl Pts',(0.216299479621054,-0.0973030578894326,
-1.03244407088623));
#70476=CARTESIAN_POINT('Ctrl Pts',(0.215816776624352,-0.098369043922167,
-1.03252207613908));
#70477=CARTESIAN_POINT('Ctrl Pts',(0.214773064428318,-0.100629281616406,
-1.03268861721428));
#70478=CARTESIAN_POINT('Ctrl Pts',(0.214209940200906,-0.10182250693968,
-1.03277722396807));
#70479=CARTESIAN_POINT('Ctrl Pts',(0.212661990869801,-0.105032836442447,
-1.03301751246413));
#70480=CARTESIAN_POINT('Ctrl Pts',(0.211658459310503,-0.107040716971319,
-1.03316983939445));
#70481=CARTESIAN_POINT('Ctrl Pts',(0.205973115019017,-0.118023390920689,
-1.03401460575423));
#70482=CARTESIAN_POINT('Ctrl Pts',(0.20074956863665,-0.126704399862393,
-1.03472602563159));
#70483=CARTESIAN_POINT('Ctrl Pts',(0.189266154706185,-0.143287568152088,
-1.03617331534723));
#70484=CARTESIAN_POINT('Ctrl Pts',(0.18302486906244,-0.151178304973489,
-1.03690751354357));
#70485=CARTESIAN_POINT('Ctrl Pts',(0.173555566406408,-0.161701292355227,
-1.03794124076664));
#70486=CARTESIAN_POINT('Ctrl Pts',(0.170729944624433,-0.164681904472389,
-1.03824078853653));
#70487=CARTESIAN_POINT('Ctrl Pts',(0.164127239337451,-0.171294090140551,
-1.03891885496641));
#70488=CARTESIAN_POINT('Ctrl Pts',(0.160304174530373,-0.174877082034531,
-1.03929623101419));
#70489=CARTESIAN_POINT('Ctrl Pts',(0.15338834197926,-0.180941078839783,
-1.03994880934473));
#70490=CARTESIAN_POINT('Ctrl Pts',(0.150346170124209,-0.183476677229564,
-1.04022635704779));
#70491=CARTESIAN_POINT('Ctrl Pts',(0.146309856512411,-0.186673028196065,
-1.04058098470663));
#70492=CARTESIAN_POINT('Ctrl Pts',(0.145372428358341,-0.187403977520671,
-1.04066242095296));
#70493=CARTESIAN_POINT('Ctrl Pts',(0.14385756255374,-0.188566970246504,
-1.04079248906902));
#70494=CARTESIAN_POINT('Ctrl Pts',(0.143283595865195,-0.189003470241006,
-1.04084142183044));
#70495=CARTESIAN_POINT('Ctrl Pts',(0.142172060499349,-0.189840816116179,
-1.040935499293));
#70496=CARTESIAN_POINT('Ctrl Pts',(0.141634773774766,-0.190242006716238,
-1.04098066637468));
#70497=CARTESIAN_POINT('Ctrl Pts',(0.14033329058457,-0.191205251109326,
-1.04108935274394));
#70498=CARTESIAN_POINT('Ctrl Pts',(0.139567398979925,-0.191765016926872,
-1.04115271534903));
#70499=CARTESIAN_POINT('Ctrl Pts',(0.136865470104579,-0.193715008495149,
-1.04137424095241));
#70500=CARTESIAN_POINT('Ctrl Pts',(0.134911779621053,-0.195080686425464,
-1.04153083019186));
#70501=CARTESIAN_POINT('Ctrl Pts',(0.130002484486339,-0.198403369614229,
-1.04191638085985));
#70502=CARTESIAN_POINT('Ctrl Pts',(0.127022900960986,-0.200324058481473,
-1.0421434049713));
#70503=CARTESIAN_POINT('Ctrl Pts',(0.113618141034676,-0.208545586738434,
-1.04313946943985));
#70504=CARTESIAN_POINT('Ctrl Pts',(0.102759146159512,-0.214104986261021,
-1.043880738825));
#70505=CARTESIAN_POINT('Ctrl Pts',(0.078353275357788,-0.224313287520356,
-1.0455031004654));
#70506=CARTESIAN_POINT('Ctrl Pts',(0.0647175072562258,-0.228620345060222,
-1.0463840388326));
#70507=CARTESIAN_POINT('Ctrl Pts',(0.047637347623109,-0.232363944843467,
-1.04751365270468));
#70508=CARTESIAN_POINT('Ctrl Pts',(0.0444829098911758,-0.232988387831591,
-1.0477232174863));
#70509=CARTESIAN_POINT('Ctrl Pts',(0.0398398767476725,-0.233809783016239,
-1.04803351471761));
#70510=CARTESIAN_POINT('Ctrl Pts',(0.0383604657410812,-0.234057054813062,
-1.04813265536811));
#70511=CARTESIAN_POINT('Ctrl Pts',(0.0357174050464013,-0.234473090029224,
-1.04831030406536));
#70512=CARTESIAN_POINT('Ctrl Pts',(0.0345546481487389,-0.234647265436907,
-1.04838863815601));
#70513=CARTESIAN_POINT('Ctrl Pts',(0.0321113181250426,-0.234994709920152,
-1.04855364629658));
#70514=CARTESIAN_POINT('Ctrl Pts',(0.0308305313350409,-0.235166172450584,
-1.04864037468291));
#70515=CARTESIAN_POINT('Ctrl Pts',(0.0274456383381947,-0.235591190419684,
-1.04887022494702));
#70516=CARTESIAN_POINT('Ctrl Pts',(0.025339465049543,-0.23582701937936,
-1.04901389887267));
#70517=CARTESIAN_POINT('Ctrl Pts',(0.0150790451899801,-0.236836847666536,
-1.04971719532552));
#70518=CARTESIAN_POINT('Ctrl Pts',(0.00689247701912053,-0.237216222349132,
-1.05028897335556));
#70519=CARTESIAN_POINT('Ctrl Pts',(-0.010935306595929,-0.237118764713752,
-1.05155725051427));
#70520=CARTESIAN_POINT('Ctrl Pts',(-0.0205611797539401,-0.23647854088466,
-1.05225689039217));
#70521=CARTESIAN_POINT('Ctrl Pts',(-0.0444813435801031,-0.233415938758958,
-1.05401705718686));
#70522=CARTESIAN_POINT('Ctrl Pts',(-0.058644734225539,-0.230266061917528,
-1.05507986613364));
#70523=CARTESIAN_POINT('Ctrl Pts',(-0.0743911535359679,-0.225215816699783,
-1.0562325388305));
#70524=CARTESIAN_POINT('Ctrl Pts',(-0.0763407755922364,-0.224562451259908,
-1.05637469061892));
#70525=CARTESIAN_POINT('Ctrl Pts',(-0.0790425019147395,-0.223617783371932,
-1.05657065681236));
#70526=CARTESIAN_POINT('Ctrl Pts',(-0.0798019216930037,-0.22334789788808,
-1.05662562681713));
#70527=CARTESIAN_POINT('Ctrl Pts',(-0.0811855277493801,-0.22284822878947,
-1.05672555160807));
#70528=CARTESIAN_POINT('Ctrl Pts',(-0.0818101510958803,-0.222619680649577,
-1.05677057736536));
#70529=CARTESIAN_POINT('Ctrl Pts',(-0.0831057230684105,-0.222139444714125,
-1.05686378099344));
#70530=CARTESIAN_POINT('Ctrl Pts',(-0.0837765028109168,-0.221887340143546,
-1.05691193388252));
#70531=CARTESIAN_POINT('Ctrl Pts',(-0.0854211649531455,-0.221260692146922,
-1.05702976892045));
#70532=CARTESIAN_POINT('Ctrl Pts',(-0.0863937492568763,-0.22088275057311,
-1.05709925327053));
#70533=CARTESIAN_POINT('Ctrl Pts',(-0.0906408796508328,-0.219199991934776,
-1.05740194390823));
#70534=CARTESIAN_POINT('Ctrl Pts',(-0.0938887913882238,-0.217828610614234,
-1.05763149561957));
#70535=CARTESIAN_POINT('Ctrl Pts',(-0.102762227709214,-0.213846563826903,
-1.05825650708259));
#70536=CARTESIAN_POINT('Ctrl Pts',(-0.108318012812955,-0.211086824224093,
-1.05864544888771));
#70537=CARTESIAN_POINT('Ctrl Pts',(-0.130906403136762,-0.198739422430882,
-1.06024208565324));
#70538=CARTESIAN_POINT('Ctrl Pts',(-0.146828358876324,-0.187283951886437,
-1.06141161880125));
#70539=CARTESIAN_POINT('Ctrl Pts',(-0.164933380982727,-0.170514934803155,
-1.06298236528416));
#70540=CARTESIAN_POINT('Ctrl Pts',(-0.16858711682625,-0.166903388366593,
-1.06331349972926));
#70541=CARTESIAN_POINT('Ctrl Pts',(-0.173407270164107,-0.161819025781277,
-1.06377224666388));
#70542=CARTESIAN_POINT('Ctrl Pts',(-0.174677868838246,-0.16044662743858,
-1.06389536941813));
#70543=CARTESIAN_POINT('Ctrl Pts',(-0.176679745124417,-0.158232396170375,
-1.06409298896214));
#70544=CARTESIAN_POINT('Ctrl Pts',(-0.177421564252611,-0.157400165186986,
-1.06416703895057));
#70545=CARTESIAN_POINT('Ctrl Pts',(-0.178938429395325,-0.155674078535312,
-1.06432017840648));
#70546=CARTESIAN_POINT('Ctrl Pts',(-0.179712708512583,-0.15477959346681,
-1.0643992967408));
#70547=CARTESIAN_POINT('Ctrl Pts',(-0.18150325000867,-0.152679523876297,
-1.06458451566304));
#70548=CARTESIAN_POINT('Ctrl Pts',(-0.182514236298725,-0.15146953526645,
-1.06469082797053));
#70549=CARTESIAN_POINT('Ctrl Pts',(-0.185601172969272,-0.147699187317175,
-1.065020919775));
#70550=CARTESIAN_POINT('Ctrl Pts',(-0.187635793692647,-0.145105659311154,
-1.0652463335768));
#70551=CARTESIAN_POINT('Ctrl Pts',(-0.195901245011749,-0.134105089604968,
-1.06619612266519));
#70552=CARTESIAN_POINT('Ctrl Pts',(-0.201625529367028,-0.125333820426734,
-1.06693914961871));
#70553=CARTESIAN_POINT('Ctrl Pts',(-0.211529526301638,-0.107714086486119,
-1.06839988381389));
#70554=CARTESIAN_POINT('Ctrl Pts',(-0.215778630985866,-0.0989274259154191,
-1.06911441030379));
#70555=CARTESIAN_POINT('Ctrl Pts',(-0.223585882280169,-0.0798683966845085,
-1.07061571497298));
#70556=CARTESIAN_POINT('Ctrl Pts',(-0.227004321879618,-0.0695607733970581,
-1.07139992012034));
#70557=CARTESIAN_POINT('Ctrl Pts',(-0.230042881720824,-0.0577415812437741,
-1.07224462298994));
#70558=CARTESIAN_POINT('Ctrl Pts',(-0.230369105492029,-0.0564259965188515,
-1.07233789547921));
#70559=CARTESIAN_POINT('Ctrl Pts',(-0.230878795950737,-0.0542924006237782,
-1.07248787250035));
#70560=CARTESIAN_POINT('Ctrl Pts',(-0.231069229930386,-0.0534761088608329,
-1.07254494774915));
#70561=CARTESIAN_POINT('Ctrl Pts',(-0.231400995248288,-0.0520191351557926,
-1.07264625677788));
#70562=CARTESIAN_POINT('Ctrl Pts',(-0.231543999827295,-0.0513788594957119,
-1.072690583158));
#70563=CARTESIAN_POINT('Ctrl Pts',(-0.231851421600686,-0.0499750822061432,
-1.07278733957547));
#70564=CARTESIAN_POINT('Ctrl Pts',(-0.232014725645907,-0.0492113570970241,
-1.07283970641063));
#70565=CARTESIAN_POINT('Ctrl Pts',(-0.232345548010314,-0.0476259397672956,
-1.07294787467687));
#70566=CARTESIAN_POINT('Ctrl Pts',(-0.232512487172898,-0.046804136345465,
-1.0730036439289));
#70567=CARTESIAN_POINT('Ctrl Pts',(-0.232934153392311,-0.044670423374128,
-1.07314770599847));
#70568=CARTESIAN_POINT('Ctrl Pts',(-0.233182161286192,-0.0433571953696926,
-1.07323565141276));
#70569=CARTESIAN_POINT('Ctrl Pts',(-0.235904953605221,-0.02824009707736,
-1.07424050055651));
#70570=CARTESIAN_POINT('Ctrl Pts',(-0.237162096468213,-0.0142434182445045,
-1.07509988565631));
#70571=CARTESIAN_POINT('Ctrl Pts',(-0.237174901177882,-0.000216509264792025,
-1.07595967459035));
#70572=CARTESIAN_POINT('Ctrl Pts',(-0.237174901130082,-0.000216561620945157,
-1.07595967138114));
#70573=CARTESIAN_POINT('Ctrl Pts',(-0.237189705431092,0.0159968773670292,
-1.07695348516814));
#70574=CARTESIAN_POINT('Ctrl Pts',(-0.235542040756606,0.0321678926258792,
-1.07794491344652));
#70575=CARTESIAN_POINT('Ctrl Pts',(-0.23176777968398,0.0504135968378846,
-1.07914569342658));
#70576=CARTESIAN_POINT('Ctrl Pts',(-0.231241459655458,0.0527751940790963,
-1.07930264939856));
#70577=CARTESIAN_POINT('Ctrl Pts',(-0.230326963019487,0.056601820864279,
-1.07955971121239));
#70578=CARTESIAN_POINT('Ctrl Pts',(-0.229960703405532,0.0580719444617723,
-1.07965913188476));
#70579=CARTESIAN_POINT('Ctrl Pts',(-0.229223751514469,0.0609136334579724,
-1.07985265145588));
#70580=CARTESIAN_POINT('Ctrl Pts',(-0.228854769686687,0.0622855781284844,
-1.07994669231565));
#70581=CARTESIAN_POINT('Ctrl Pts',(-0.228160513377715,0.0647774704341915,
-1.08011865490051));
#70582=CARTESIAN_POINT('Ctrl Pts',(-0.227839259636772,0.0658984994159516,
-1.0801964439192));
#70583=CARTESIAN_POINT('Ctrl Pts',(-0.227125513974596,0.0683215244334877,
-1.08036553061352));
#70584=CARTESIAN_POINT('Ctrl Pts',(-0.226730067126667,0.0696225992475412,
-1.0804569224322));
#70585=CARTESIAN_POINT('Ctrl Pts',(-0.225615527623977,0.0731793646603695,
-1.08070844333898));
#70586=CARTESIAN_POINT('Ctrl Pts',(-0.224873830338733,0.0754277497807674,
-1.08086930698658));
#70587=CARTESIAN_POINT('Ctrl Pts',(-0.22021373697241,0.0888742967680971,
-1.08184294133655));
#70588=CARTESIAN_POINT('Ctrl Pts',(-0.215493881720441,0.0997749392634271,
-1.08268214585097));
#70589=CARTESIAN_POINT('Ctrl Pts',(-0.20511130094733,0.119544773962779,
-1.08429505731352));
#70590=CARTESIAN_POINT('Ctrl Pts',(-0.199634968243343,0.12848137665573,
-1.08506290981648));
#70591=CARTESIAN_POINT('Ctrl Pts',(-0.187760438733647,0.145257311659727,
-1.08655983209413));
#70592=CARTESIAN_POINT('Ctrl Pts',(-0.181414726954496,0.153109151133245,
-1.08728768669437));
#70593=CARTESIAN_POINT('Ctrl Pts',(-0.173496847363707,0.161720196384054,
-1.08809896660234));
#70594=CARTESIAN_POINT('Ctrl Pts',(-0.172393903535983,0.162895427631929,
-1.08820998287201));
#70595=CARTESIAN_POINT('Ctrl Pts',(-0.170818043531506,0.164540635583799,
-1.08836569809185));
#70596=CARTESIAN_POINT('Ctrl Pts',(-0.170355025013027,0.165019969198535,
-1.08841110296346));
#70597=CARTESIAN_POINT('Ctrl Pts',(-0.169424678355614,0.165975009130238,
-1.08850163178614));
#70598=CARTESIAN_POINT('Ctrl Pts',(-0.168957350123588,0.166450710954488,
-1.08854675488551));
#70599=CARTESIAN_POINT('Ctrl Pts',(-0.16797443054146,0.167442837392409,
-1.08864091991015));
#70600=CARTESIAN_POINT('Ctrl Pts',(-0.167458456231117,0.16795885979261,
-1.08868993110858));
#70601=CARTESIAN_POINT('Ctrl Pts',(-0.166067952773326,0.169336715430872,
-1.08882091867736));
#70602=CARTESIAN_POINT('Ctrl Pts',(-0.165189084824151,0.170194167196048,
-1.08890256112305));
#70603=CARTESIAN_POINT('Ctrl Pts',(-0.161167755970908,0.174057007744811,
-1.0892711727207));
#70604=CARTESIAN_POINT('Ctrl Pts',(-0.157949453299136,0.17698266422769,
-1.08955261297817));
#70605=CARTESIAN_POINT('Ctrl Pts',(-0.142864086655325,0.189956790708876,
-1.09082134948087));
#70606=CARTESIAN_POINT('Ctrl Pts',(-0.130106477553162,0.198912351494917,
-1.09175869978726));
#70607=CARTESIAN_POINT('Ctrl Pts',(-0.108842398924777,0.210912074384467,
-1.0932610700988));
#70608=CARTESIAN_POINT('Ctrl Pts',(-0.100884075607825,0.214832389749444,
-1.09381122744024));
#70609=CARTESIAN_POINT('Ctrl Pts',(-0.0893760010614183,0.219720628298945,
-1.09460603843072));
#70610=CARTESIAN_POINT('Ctrl Pts',(-0.0859943345376999,0.221066045291664,
-1.09483945884671));
#70611=CARTESIAN_POINT('Ctrl Pts',(-0.07993135007801,0.223318074355819,
-1.09525871385966));
#70612=CARTESIAN_POINT('Ctrl Pts',(-0.0772622037864236,0.224255510103424,
-1.095443537421));
#70613=CARTESIAN_POINT('Ctrl Pts',(-0.0732085240462829,0.225598251084243,
-1.09572492300848));
#70614=CARTESIAN_POINT('Ctrl Pts',(-0.0718359505443863,0.226039056226831,
-1.09582031734134));
#70615=CARTESIAN_POINT('Ctrl Pts',(-0.0693448632070169,0.226814093862479,
-1.09599370101598));
#70616=CARTESIAN_POINT('Ctrl Pts',(-0.0682277300479967,0.227152635900668,
-1.09607154634389));
#70617=CARTESIAN_POINT('Ctrl Pts',(-0.0658197149485878,0.227863007776267,
-1.09623956181735));
#70618=CARTESIAN_POINT('Ctrl Pts',(-0.0645280872643494,0.228232142814565,
-1.09632981677997));
#70619=CARTESIAN_POINT('Ctrl Pts',(-0.0610221660207296,0.22920196260782,
-1.09657519654198));
#70620=CARTESIAN_POINT('Ctrl Pts',(-0.0588022272735147,0.229781508898124,
-1.09673099792073));
#70621=CARTESIAN_POINT('Ctrl Pts',(-0.0517282751309758,0.231519042232843,
-1.0972289725201));
#70622=CARTESIAN_POINT('Ctrl Pts',(-0.0468474911537617,0.232555716920545,
-1.097574825708));
#70623=CARTESIAN_POINT('Ctrl Pts',(-0.0419392646935193,0.233437526336206,
-1.0979250019446));
#70624=CARTESIAN_POINT('',(-0.237174998221465,2.9045624302765E-5,-1.09587916587548));
#70625=CARTESIAN_POINT('Ctrl Pts',(-0.0419392769977373,0.233437524125636,
-1.11762795217595));
#70626=CARTESIAN_POINT('Ctrl Pts',(-0.0513124259767892,0.231753548540109,
-1.11701686568024));
#70627=CARTESIAN_POINT('Ctrl Pts',(-0.0605790275699475,0.229505954888564,
-1.11642777064907));
#70628=CARTESIAN_POINT('Ctrl Pts',(-0.0879950868366662,0.221078376363219,
-1.11466574714866));
#70629=CARTESIAN_POINT('Ctrl Pts',(-0.105550654404818,0.213255150629247,
-1.11350513299769));
#70630=CARTESIAN_POINT('Ctrl Pts',(-0.124485368601723,0.201900837211246,
-1.11207603739078));
#70631=CARTESIAN_POINT('Ctrl Pts',(-0.126968473698413,0.200348597502796,
-1.1118849554608));
#70632=CARTESIAN_POINT('Ctrl Pts',(-0.130674118200915,0.197935564341248,
-1.11159383872476));
#70633=CARTESIAN_POINT('Ctrl Pts',(-0.131918361143883,0.19710849454021,
-1.11149505217501));
#70634=CARTESIAN_POINT('Ctrl Pts',(-0.134100395479711,0.195628143615694,
-1.11131992125608));
#70635=CARTESIAN_POINT('Ctrl Pts',(-0.135041443410467,0.194979730037483,
-1.11124376235253));
#70636=CARTESIAN_POINT('Ctrl Pts',(-0.136110315901974,0.194231791184795,
-1.11115652475097));
#70637=CARTESIAN_POINT('Ctrl Pts',(-0.136242782026103,0.194138896533777,
-1.11114570038463));
#70638=CARTESIAN_POINT('Ctrl Pts',(-0.136434573915127,0.194004105473234,
-1.11113000944803));
#70639=CARTESIAN_POINT('Ctrl Pts',(-0.136493975877539,0.19396231708503,
-1.11112514701839));
#70640=CARTESIAN_POINT('Ctrl Pts',(-0.136596076258444,0.193890420870757,
-1.11111678494384));
#70641=CARTESIAN_POINT('Ctrl Pts',(-0.136638783968,0.193860326189709,-1.11111328580322));
#70642=CARTESIAN_POINT('Ctrl Pts',(-0.136713822532998,0.193807411931112,
-1.11110713533475));
#70643=CARTESIAN_POINT('Ctrl Pts',(-0.136746157640387,0.193784598360156,
-1.11110448423746));
#70644=CARTESIAN_POINT('Ctrl Pts',(-0.136803821010411,0.193743893177523,
-1.1110997551306));
#70645=CARTESIAN_POINT('Ctrl Pts',(-0.136829151483132,0.193726004684545,
-1.11109767724079));
#70646=CARTESIAN_POINT('Ctrl Pts',(-0.136874810623106,0.193693746573373,
-1.11109393090156));
#70647=CARTESIAN_POINT('Ctrl Pts',(-0.136895140541188,0.193679378718925,
-1.11109226251991));
#70648=CARTESIAN_POINT('Ctrl Pts',(-0.13693208422009,0.193653260623795,
-1.11108923016277));
#70649=CARTESIAN_POINT('Ctrl Pts',(-0.136948698734297,0.193641511443357,
-1.11108786622799));
#70650=CARTESIAN_POINT('Ctrl Pts',(-0.137008028291522,0.193599544282447,
-1.11108299495096));
#70651=CARTESIAN_POINT('Ctrl Pts',(-0.137050734821078,0.193569314323569,
-1.11107948714864));
#70652=CARTESIAN_POINT('Ctrl Pts',(-0.137134931478892,0.193509673607565,
-1.11107256876076));
#70653=CARTESIAN_POINT('Ctrl Pts',(-0.137176422159569,0.193480263631512,
-1.11106915820536));
#70654=CARTESIAN_POINT('Ctrl Pts',(-0.13725849991559,0.193422044512001,
-1.11106240881374));
#70655=CARTESIAN_POINT('Ctrl Pts',(-0.137299087389185,0.193393235932311,
-1.11105906999934));
#70656=CARTESIAN_POINT('Ctrl Pts',(-0.137379628812475,0.193336030307493,
-1.1110524420258));
#70657=CARTESIAN_POINT('Ctrl Pts',(-0.137419583034138,0.193307633647589,
-1.11104915288157));
#70658=CARTESIAN_POINT('Ctrl Pts',(-0.13749909645943,0.193251083969447,
-1.1110426047171));
#70659=CARTESIAN_POINT('Ctrl Pts',(-0.137538655827348,0.193222931185007,
-1.11103934570595));
#70660=CARTESIAN_POINT('Ctrl Pts',(-0.13761759481541,0.193166717009997,
-1.11103284013317));
#70661=CARTESIAN_POINT('Ctrl Pts',(-0.137656974504486,0.193138655720351,
-1.11102959357555));
#70662=CARTESIAN_POINT('Ctrl Pts',(-0.13773575257702,0.193082483486986,
-1.11102309657168));
#70663=CARTESIAN_POINT('Ctrl Pts',(-0.137775150942949,0.193054372522619,
-1.11101984612473));
#70664=CARTESIAN_POINT('Ctrl Pts',(-0.13907151442299,0.192128810646984,
-1.11091285472892));
#70665=CARTESIAN_POINT('Ctrl Pts',(-0.140319665436949,0.191219134239798,
-1.11080864375046));
#70666=CARTESIAN_POINT('Ctrl Pts',(-0.144603356338511,0.188032572701308,
-1.11044675414118));
#70667=CARTESIAN_POINT('Ctrl Pts',(-0.147592942604134,0.185695178882195,
-1.11018673188702));
#70668=CARTESIAN_POINT('Ctrl Pts',(-0.160659273511638,0.174964424376129,
-1.10901576787797));
#70669=CARTESIAN_POINT('Ctrl Pts',(-0.170084274352997,0.16581675588369,
-1.10807502211549));
#70670=CARTESIAN_POINT('Ctrl Pts',(-0.189708403693762,0.143327719309288,
-1.10590185709727));
#70671=CARTESIAN_POINT('Ctrl Pts',(-0.1993476841613,0.129586623932666,-1.10466559195508));
#70672=CARTESIAN_POINT('Ctrl Pts',(-0.20837924384152,0.113285773984156,
-1.1033690331386));
#70673=CARTESIAN_POINT('Ctrl Pts',(-0.209278287117749,0.111616194890113,
-1.10323812199244));
#70674=CARTESIAN_POINT('Ctrl Pts',(-0.210554283924761,0.109176956607938,
-1.10304977434837));
#70675=CARTESIAN_POINT('Ctrl Pts',(-0.21094721557263,0.108415804351397,
-1.10299140818392));
#70676=CARTESIAN_POINT('Ctrl Pts',(-0.211635058066689,0.107065479343845,
-1.10288860314279));
#70677=CARTESIAN_POINT('Ctrl Pts',(-0.21193164910076,0.106477184508045,
-1.10284406175229));
#70678=CARTESIAN_POINT('Ctrl Pts',(-0.212564060930533,0.105209670138415,
-1.10274863118305));
#70679=CARTESIAN_POINT('Ctrl Pts',(-0.212899081064536,0.10453007228669,
-1.10269779118598));
#70680=CARTESIAN_POINT('Ctrl Pts',(-0.213824737935954,0.102629439193682,
-1.10255648343408));
#70681=CARTESIAN_POINT('Ctrl Pts',(-0.2144081771224,0.101404901954349,-1.10246644628672));
#70682=CARTESIAN_POINT('Ctrl Pts',(-0.217940070430203,0.0938252929915238,
-1.1019148907721));
#70683=CARTESIAN_POINT('Ctrl Pts',(-0.22061656241397,0.0873465121088174,
-1.1014682033649));
#70684=CARTESIAN_POINT('Ctrl Pts',(-0.229720042864398,0.0622084831613126,
-1.09979318034984));
#70685=CARTESIAN_POINT('Ctrl Pts',(-0.234097051542799,0.0428932200546185,
-1.09861844446422));
#70686=CARTESIAN_POINT('Ctrl Pts',(-0.236542681461396,0.0180741705037209,
-1.0970467851354));
#70687=CARTESIAN_POINT('Ctrl Pts',(-0.236882552585845,0.0128750230385105,
-1.09671465885293));
#70688=CARTESIAN_POINT('Ctrl Pts',(-0.237133342782771,0.00512319446735597,
-1.09621256739257));
#70689=CARTESIAN_POINT('Ctrl Pts',(-0.237174686289266,0.00257615970376124,
-1.09604649594697));
#70690=CARTESIAN_POINT('Ctrl Pts',(-0.237174998221465,2.9045624302765E-5,
-1.09587916587548));
#70691=CARTESIAN_POINT('Ctrl Pts',(-0.237174998234998,2.89349044827048E-5,
-1.09587915860185));
#70692=CARTESIAN_POINT('Ctrl Pts',(-0.237175091574553,-0.000736155186613617,
-1.09582889677479));
#70693=CARTESIAN_POINT('Ctrl Pts',(-0.237171482819,-0.00150123555575333,
-1.09577852271994));
#70694=CARTESIAN_POINT('Ctrl Pts',(-0.23715504772398,-0.00322115387109381,
-1.09566501874773));
#70695=CARTESIAN_POINT('Ctrl Pts',(-0.237140156594989,-0.00417595238553839,
-1.09560182641588));
#70696=CARTESIAN_POINT('Ctrl Pts',(-0.237095373510457,-0.00624567023885131,
-1.09546443665023));
#70697=CARTESIAN_POINT('Ctrl Pts',(-0.237063382370882,-0.00736051648109467,
-1.0953901755463));
#70698=CARTESIAN_POINT('Ctrl Pts',(-0.236978720384648,-0.00972826804894033,
-1.0952318923194));
#70699=CARTESIAN_POINT('Ctrl Pts',(-0.236923973729274,-0.0109810601484171,
-1.09514780747047));
#70700=CARTESIAN_POINT('Ctrl Pts',(-0.236762754412604,-0.0141025542018507,
-1.09493743284993));
#70701=CARTESIAN_POINT('Ctrl Pts',(-0.236644091988894,-0.0159705130882173,
-1.09481076574039));
#70702=CARTESIAN_POINT('Ctrl Pts',(-0.236094200314016,-0.0232616765908722,
-1.0943132047075));
#70703=CARTESIAN_POINT('Ctrl Pts',(-0.235498567749214,-0.0286704243256552,
-1.09393724537711));
#70704=CARTESIAN_POINT('Ctrl Pts',(-0.2340185606868,-0.0388715235886166,
-1.09321467972771));
#70705=CARTESIAN_POINT('Ctrl Pts',(-0.233171416259019,-0.0436665498414046,
-1.0928693168324));
#70706=CARTESIAN_POINT('Ctrl Pts',(-0.227849219730846,-0.0691806141151254,
-1.09100251286758));
#70707=CARTESIAN_POINT('Ctrl Pts',(-0.2207598883747,-0.089253678435357,
-1.08941896474834));
#70708=CARTESIAN_POINT('Ctrl Pts',(-0.209741828236302,-0.110766449464546,
-1.08771852858905));
#70709=CARTESIAN_POINT('Ctrl Pts',(-0.208335094052613,-0.113390173611633,
-1.08751128898664));
#70710=CARTESIAN_POINT('Ctrl Pts',(-0.20637403424456,-0.116888005894681,
-1.08723588371031));
#70711=CARTESIAN_POINT('Ctrl Pts',(-0.205862915114923,-0.117785857436639,
-1.08716526998915));
#70712=CARTESIAN_POINT('Ctrl Pts',(-0.205002201128749,-0.119275102290707,
-1.08704831370501));
#70713=CARTESIAN_POINT('Ctrl Pts',(-0.204655879845547,-0.119868358521215,
-1.0870017680091));
#70714=CARTESIAN_POINT('Ctrl Pts',(-0.203995683534527,-0.12098808778858,
-1.08691401392839));
#70715=CARTESIAN_POINT('Ctrl Pts',(-0.203682337780679,-0.121514861582823,
-1.08687277112295));
#70716=CARTESIAN_POINT('Ctrl Pts',(-0.202851360180702,-0.12289959441002,
-1.08676444763731));
#70717=CARTESIAN_POINT('Ctrl Pts',(-0.202330320372337,-0.123755509700915,
-1.0866975851608));
#70718=CARTESIAN_POINT('Ctrl Pts',(-0.200466677005719,-0.126773695326562,
-1.08646204580914));
#70719=CARTESIAN_POINT('Ctrl Pts',(-0.199094655138995,-0.128917717934579,
-1.08629515694414));
#70720=CARTESIAN_POINT('Ctrl Pts',(-0.188870209299772,-0.144342501461747,
-1.08509445881174));
#70721=CARTESIAN_POINT('Ctrl Pts',(-0.178730613517719,-0.156723374597824,
-1.08412848094404));
#70722=CARTESIAN_POINT('Ctrl Pts',(-0.157112003028982,-0.178268626637153,
-1.08225579875219));
#70723=CARTESIAN_POINT('Ctrl Pts',(-0.145878519487975,-0.187572023640914,
-1.08135497780248));
#70724=CARTESIAN_POINT('Ctrl Pts',(-0.132277133420145,-0.196871623893918,
-1.08028575335904));
#70725=CARTESIAN_POINT('Ctrl Pts',(-0.130677092782299,-0.197937296623947,
-1.08016032714827));
#70726=CARTESIAN_POINT('Ctrl Pts',(-0.127964092362337,-0.199696999049357,
-1.07994813762921));
#70727=CARTESIAN_POINT('Ctrl Pts',(-0.126857992604295,-0.200401471953222,
-1.07986175943789));
#70728=CARTESIAN_POINT('Ctrl Pts',(-0.124681395355753,-0.201762501937129,
-1.07969200504493));
#70729=CARTESIAN_POINT('Ctrl Pts',(-0.123611412024013,-0.202419802020645,
-1.07960865960593));
#70730=CARTESIAN_POINT('Ctrl Pts',(-0.121575919518454,-0.203648065363674,
-1.07945027477432));
#70731=CARTESIAN_POINT('Ctrl Pts',(-0.120611478102009,-0.204220738439006,
-1.07937530062942));
#70732=CARTESIAN_POINT('Ctrl Pts',(-0.118339985056488,-0.205547819302834,
-1.07919886278744));
#70733=CARTESIAN_POINT('Ctrl Pts',(-0.117029735858778,-0.206296628243834,
-1.07909720025318));
#70734=CARTESIAN_POINT('Ctrl Pts',(-0.113094023585103,-0.208496331788863,
-1.07879210453458));
#70735=CARTESIAN_POINT('Ctrl Pts',(-0.110448173802008,-0.209909928318222,
-1.07858735915639));
#70736=CARTESIAN_POINT('Ctrl Pts',(-0.0913656990865444,-0.219644442121292,
-1.07711260343937));
#70737=CARTESIAN_POINT('Ctrl Pts',(-0.0740385308444054,-0.226073912500243,
-1.075776182441));
#70738=CARTESIAN_POINT('Ctrl Pts',(-0.0525204209895835,-0.231316911483036,
-1.07415868752096));
#70739=CARTESIAN_POINT('Ctrl Pts',(-0.0488741492114006,-0.232114683593674,
-1.07388628746343));
#70740=CARTESIAN_POINT('Ctrl Pts',(-0.0388544078163394,-0.234060332633326,
-1.07314424345131));
#70741=CARTESIAN_POINT('Ctrl Pts',(-0.032449957179367,-0.235033861177777,
-1.07267700638897));
#70742=CARTESIAN_POINT('Ctrl Pts',(-0.0223970304159877,-0.236143156378797,
-1.07196153656108));
#70743=CARTESIAN_POINT('Ctrl Pts',(-0.0187718046415923,-0.236458960940458,
-1.07170715473292));
#70744=CARTESIAN_POINT('Ctrl Pts',(-0.0140312424593468,-0.236762202170247,
-1.07138041968398));
#70745=CARTESIAN_POINT('Ctrl Pts',(-0.0129214589011289,-0.23682536216366,
-1.07130435196625));
#70746=CARTESIAN_POINT('Ctrl Pts',(-0.0111082135382834,-0.236915773428376,
-1.07118080037567));
#70747=CARTESIAN_POINT('Ctrl Pts',(-0.0104050176440958,-0.236947698338747,
-1.07113306575395));
#70748=CARTESIAN_POINT('Ctrl Pts',(-0.00903007294455535,-0.237003987767055,
-1.07104009660934));
#70749=CARTESIAN_POINT('Ctrl Pts',(-0.00835834786370987,-0.237028627961647,
-1.07099484813483));
#70750=CARTESIAN_POINT('Ctrl Pts',(-0.00685271293237036,-0.237077449192227,
-1.07089379231548));
#70751=CARTESIAN_POINT('Ctrl Pts',(-0.0060187534657266,-0.237100086986591,
-1.07083806979067));
#70752=CARTESIAN_POINT('Ctrl Pts',(-0.00310644659155155,-0.237163765609716,
-1.07064430234653));
#70753=CARTESIAN_POINT('Ctrl Pts',(-0.0010276219452319,-0.237181884733494,
-1.07050745403679));
#70754=CARTESIAN_POINT('Ctrl Pts',(0.0130863627277286,-0.237119325070918,
-1.06958664053427));
#70755=CARTESIAN_POINT('Ctrl Pts',(0.0251015762151883,-0.236149978756105,
-1.06884324054553));
#70756=CARTESIAN_POINT('Ctrl Pts',(0.0475138118662097,-0.23261099535582,
-1.06745032962378));
#70757=CARTESIAN_POINT('Ctrl Pts',(0.0579110556338668,-0.230242781766925,
-1.06680137983303));
#70758=CARTESIAN_POINT('Ctrl Pts',(0.0770815438338459,-0.224495144659416,
-1.06555484079948));
#70759=CARTESIAN_POINT('Ctrl Pts',(0.0858814662879557,-0.221278053191992,
-1.06496173061427));
#70760=CARTESIAN_POINT('Ctrl Pts',(0.0964852814027841,-0.216673509714544,
-1.06420766652896));
#70761=CARTESIAN_POINT('Ctrl Pts',(0.0984906270219844,-0.215769356475152,
-1.06406328178946));
#70762=CARTESIAN_POINT('Ctrl Pts',(0.101669132734447,-0.214282716537924,
-1.06383142868202));
#70763=CARTESIAN_POINT('Ctrl Pts',(0.102850577795691,-0.213718164151304,
-1.06374457868879));
#70764=CARTESIAN_POINT('Ctrl Pts',(0.105079993683318,-0.212630072589506,
-1.06357938474551));
#70765=CARTESIAN_POINT('Ctrl Pts',(0.10612888203209,-0.212108493831807,
-1.06350111096879));
#70766=CARTESIAN_POINT('Ctrl Pts',(0.10850479443007,-0.210904993185594,
-1.06332252101537));
#70767=CARTESIAN_POINT('Ctrl Pts',(0.109829323046227,-0.210218282237729,
-1.06322203890897));
#70768=CARTESIAN_POINT('Ctrl Pts',(0.113875523225334,-0.208071824061476,
-1.06291218950026));
#70769=CARTESIAN_POINT('Ctrl Pts',(0.116575139732711,-0.206571425869621,
-1.06270139366936));
#70770=CARTESIAN_POINT('Ctrl Pts',(0.134940388899677,-0.195889691099852,
-1.06123844749755));
#70771=CARTESIAN_POINT('Ctrl Pts',(0.149533093597661,-0.184989972385553,
-1.05992212966255));
#70772=CARTESIAN_POINT('Ctrl Pts',(0.165544430822195,-0.169887944322956,
-1.05831462477069));
#70773=CARTESIAN_POINT('Ctrl Pts',(0.168286668523524,-0.167171977485508,
-1.05803288850312));
#70774=CARTESIAN_POINT('Ctrl Pts',(0.175495847398169,-0.159674626734347,
-1.05727656477406));
#70775=CARTESIAN_POINT('Ctrl Pts',(0.179833520130493,-0.154773044979963,
-1.0568043292003));
#70776=CARTESIAN_POINT('Ctrl Pts',(0.186275209715283,-0.146856884427125,
-1.05608221386023));
#70777=CARTESIAN_POINT('Ctrl Pts',(0.18852122677911,-0.143962317855598,
-1.05582606020811));
#70778=CARTESIAN_POINT('Ctrl Pts',(0.19136190051001,-0.140120823239754,
-1.05549742024885));
#70779=CARTESIAN_POINT('Ctrl Pts',(0.192018065215006,-0.139220274481664,
-1.05542116715528));
#70780=CARTESIAN_POINT('Ctrl Pts',(0.193078717955802,-0.137742824145694,
-1.055297390978));
#70781=CARTESIAN_POINT('Ctrl Pts',(0.193487015613042,-0.137168698154314,
-1.05524961546611));
#70782=CARTESIAN_POINT('Ctrl Pts',(0.194279639560536,-0.1360435722647,-1.05515663142343));
#70783=CARTESIAN_POINT('Ctrl Pts',(0.194664191553741,-0.135492746839748,
-1.05511140850166));
#70784=CARTESIAN_POINT('Ctrl Pts',(0.195520196121846,-0.134255454313557,
-1.05501047662591));
#70785=CARTESIAN_POINT('Ctrl Pts',(0.195990388869477,-0.133568116058034,
-1.05495485181618));
#70786=CARTESIAN_POINT('Ctrl Pts',(0.197616678398928,-0.131163691172546,
-1.05476175725491));
#70787=CARTESIAN_POINT('Ctrl Pts',(0.198753948395189,-0.129433898867819,
-1.05462547325677));
#70788=CARTESIAN_POINT('Ctrl Pts',(0.206427772586406,-0.117422283885265,
-1.05369545313188));
#70789=CARTESIAN_POINT('Ctrl Pts',(0.212187092026569,-0.106663643226348,
-1.05294336708235));
#70790=CARTESIAN_POINT('Ctrl Pts',(0.22148826207626,-0.0855217818231289,
-1.05152570006612));
#70791=CARTESIAN_POINT('Ctrl Pts',(0.225187494961732,-0.0752436529550886,
-1.05086090103726));
#70792=CARTESIAN_POINT('Ctrl Pts',(0.230625826470045,-0.0560794113212364,
-1.04961829083679));
#70793=CARTESIAN_POINT('Ctrl Pts',(0.232589460107917,-0.0472788204214101,
-1.04904664657693));
#70794=CARTESIAN_POINT('Ctrl Pts',(0.234400022564185,-0.0362401678811255,
-1.04831681355707));
#70795=CARTESIAN_POINT('Ctrl Pts',(0.234722793368587,-0.034087095810669,
-1.04817388664357));
#70796=CARTESIAN_POINT('Ctrl Pts',(0.235191488870558,-0.0306373282530253,
-1.04794382495191));
#70797=CARTESIAN_POINT('Ctrl Pts',(0.235356436951206,-0.0293433091148237,
-1.04785729162268));
#70798=CARTESIAN_POINT('Ctrl Pts',(0.235649343438506,-0.0268838620793663,
-1.04769234555208));
#70799=CARTESIAN_POINT('Ctrl Pts',(0.235779351885715,-0.0257187138578892,
-1.04761399999654));
#70800=CARTESIAN_POINT('Ctrl Pts',(0.236056057896234,-0.0230601373195481,
-1.04743474919486));
#70801=CARTESIAN_POINT('Ctrl Pts',(0.236197229786942,-0.0215661972405644,
-1.04733367337973));
#70802=CARTESIAN_POINT('Ctrl Pts',(0.236589422685795,-0.016948367597855,
-1.04702011391224));
#70803=CARTESIAN_POINT('Ctrl Pts',(0.2367927022762,-0.0138208755589679,
-1.0468061515963));
#70804=CARTESIAN_POINT('Ctrl Pts',(0.237722037298659,0.00677620364881257,
-1.04538587271513));
#70805=CARTESIAN_POINT('Ctrl Pts',(0.236576147313844,0.0242732632793495,
-1.04412065615394));
#70806=CARTESIAN_POINT('Ctrl Pts',(0.231077711792158,0.0552262430860495,
-1.04182459464647));
#70807=CARTESIAN_POINT('Ctrl Pts',(0.227427272091829,0.0687296762748372,
-1.04080404284123));
#70808=CARTESIAN_POINT('Ctrl Pts',(0.222090132341755,0.0832479479033649,
-1.03973332840307));
#70809=CARTESIAN_POINT('Ctrl Pts',(0.221557148684481,0.0846562335241625,
-1.03962977432557));
#70810=CARTESIAN_POINT('Ctrl Pts',(0.220724352835959,0.0867949524713409,
-1.03947307988995));
#70811=CARTESIAN_POINT('Ctrl Pts',(0.220434257605839,0.0875290913289815,
-1.03941939594348));
#70812=CARTESIAN_POINT('Ctrl Pts',(0.219896656181607,0.0888699643860071,
-1.03932155150976));
#70813=CARTESIAN_POINT('Ctrl Pts',(0.219650299542593,0.0894771250243933,
-1.0392773264773));
#70814=CARTESIAN_POINT('Ctrl Pts',(0.219087230717095,0.0908485015742039,
-1.03917761291892));
#70815=CARTESIAN_POINT('Ctrl Pts',(0.21876903443996,0.0916120872141515,
-1.03912221427717));
#70816=CARTESIAN_POINT('Ctrl Pts',(0.217933084267518,0.093588949350268,
-1.03897906968969));
#70817=CARTESIAN_POINT('Ctrl Pts',(0.217409183732837,0.094799618574917,
-1.03889167822227));
#70818=CARTESIAN_POINT('Ctrl Pts',(0.213580967907953,0.103447474205728,
-1.03826896095055));
#70819=CARTESIAN_POINT('Ctrl Pts',(0.209905514373401,0.110715470439914,
-1.03775364882532));
#70820=CARTESIAN_POINT('Ctrl Pts',(0.203568743915175,0.121791192591615,
-1.03695921095531));
#70821=CARTESIAN_POINT('Ctrl Pts',(0.201157532622864,0.125733756117386,
-1.03667449757163));
#70822=CARTESIAN_POINT('Ctrl Pts',(0.193202655206651,0.137925546639449,
-1.03578044117108));
#70823=CARTESIAN_POINT('Ctrl Pts',(0.187255165100317,0.145897979656046,
-1.03517502885233));
#70824=CARTESIAN_POINT('Ctrl Pts',(0.174176957476517,0.161306931076453,
-1.03392066065903));
#70825=CARTESIAN_POINT('Ctrl Pts',(0.167027487007076,0.168698896557807,
-1.03327217708998));
#70826=CARTESIAN_POINT('Ctrl Pts',(0.157754326489912,0.177117549237143,
-1.03245568373969));
#70827=CARTESIAN_POINT('Ctrl Pts',(0.156065250086892,0.178607645179499,
-1.03230790604976));
#70828=CARTESIAN_POINT('Ctrl Pts',(0.153352434336726,0.180933015403953,
-1.03207188359628));
#70829=CARTESIAN_POINT('Ctrl Pts',(0.152342468736309,0.181784205253794,
-1.03198429735767));
#70830=CARTESIAN_POINT('Ctrl Pts',(0.150424938152886,0.183373079636745,
-1.03181850480131));
#70831=CARTESIAN_POINT('Ctrl Pts',(0.149518920503259,0.184112576107187,
-1.03174037548469));
#70832=CARTESIAN_POINT('Ctrl Pts',(0.147459360863589,0.18576837112643,-1.03156321280375));
#70833=CARTESIAN_POINT('Ctrl Pts',(0.146302685382501,0.186680676280721,
-1.03146402359801));
#70834=CARTESIAN_POINT('Ctrl Pts',(0.142850364442756,0.189351834811302,
-1.03116883024725));
#70835=CARTESIAN_POINT('Ctrl Pts',(0.140531036795825,0.191079487061952,
-1.03097161614323));
#70836=CARTESIAN_POINT('Ctrl Pts',(0.122165203349238,0.204244819851684,
-1.02941780110421));
#70837=CARTESIAN_POINT('Ctrl Pts',(0.104784162220107,0.213682601983038,
-1.02798368722188));
#70838=CARTESIAN_POINT('Ctrl Pts',(0.0841692305464473,0.221750930055794,
-1.02636782537346));
#70839=CARTESIAN_POINT('Ctrl Pts',(0.0818834250948052,0.222605119581157,
-1.02618990283439));
#70840=CARTESIAN_POINT('Ctrl Pts',(0.0733384096662811,0.225648901353173,
-1.02553012043249));
#70841=CARTESIAN_POINT('Ctrl Pts',(0.067000990327593,0.227611133647803,
-1.02505127370563));
#70842=CARTESIAN_POINT('Ctrl Pts',(0.0570163551471063,0.230249371175679,
-1.02432038737577));
#70843=CARTESIAN_POINT('Ctrl Pts',(0.0534216029919816,0.231109873773933,
-1.02406190742171));
#70844=CARTESIAN_POINT('Ctrl Pts',(0.0487152233525572,0.232120780696613,
-1.02373076888635));
#70845=CARTESIAN_POINT('Ctrl Pts',(0.0476208014169346,0.232347776435435,
-1.02365427435596));
#70846=CARTESIAN_POINT('Ctrl Pts',(0.0458332384667774,0.232705376511691,
-1.02353020565478));
#70847=CARTESIAN_POINT('Ctrl Pts',(0.0451410629968801,0.232840637498089,
-1.02348237686285));
#70848=CARTESIAN_POINT('Ctrl Pts',(0.0437889121513203,0.23309861087764,
-1.02338937283421));
#70849=CARTESIAN_POINT('Ctrl Pts',(0.0431290049686393,0.233221611707747,
-1.02334418263677));
#70850=CARTESIAN_POINT('Ctrl Pts',(0.0416511707215966,0.233490579871536,
-1.02324341014954));
#70851=CARTESIAN_POINT('Ctrl Pts',(0.0408329725228978,0.233635055841077,
-1.02318791113496));
#70852=CARTESIAN_POINT('Ctrl Pts',(0.0379847521636842,0.23412257000662,
-1.02299567993711));
#70853=CARTESIAN_POINT('Ctrl Pts',(0.0359509664546327,0.234443485511614,
-1.02286011965641));
#70854=CARTESIAN_POINT('Ctrl Pts',(0.0209030832056344,0.23661749123796,
-1.0218679409433));
#70855=CARTESIAN_POINT('Ctrl Pts',(0.00775741603820414,0.237412491359641,
-1.02106005793333));
#70856=CARTESIAN_POINT('Ctrl Pts',(-0.0176494674194245,0.236835177217374,
-1.01950176485479));
#70857=CARTESIAN_POINT('Ctrl Pts',(-0.0298697332375505,0.235605932599213,
-1.01875328707626));
#70858=CARTESIAN_POINT('Ctrl Pts',(-0.0419392742985053,0.233437524610579,
-1.01798096863704));
#70859=CARTESIAN_POINT('Origin',(0.,0.,-2.1456589891905));
#70860=CARTESIAN_POINT('',(-0.0419392741323876,0.233437524640424,-0.898335233456629));
#70861=CARTESIAN_POINT('',(-0.0419392742314872,0.23343752462262,-0.917975447697368));
#70862=CARTESIAN_POINT('',(-0.0419392741328076,0.233437524640348,-2.1456589891905));
#70863=CARTESIAN_POINT('Ctrl Pts',(-0.0419392741323876,0.233437524640424,
-0.898335233456629));
#70864=CARTESIAN_POINT('Ctrl Pts',(-0.0403252167073179,0.233727505426162,
-0.898443857794283));
#70865=CARTESIAN_POINT('Ctrl Pts',(-0.038708130257032,0.234000749953858,
-0.898551621961256));
#70866=CARTESIAN_POINT('Ctrl Pts',(-0.0251098457204889,0.236153669473257,
-0.899449899231117));
#70867=CARTESIAN_POINT('Ctrl Pts',(-0.0130019729095658,0.237128835285574,
-0.900198716281383));
#70868=CARTESIAN_POINT('Ctrl Pts',(0.00992325448858503,0.237213055365717,
-0.901605921069753));
#70869=CARTESIAN_POINT('Ctrl Pts',(0.0207077636629997,0.236515715439281,
-0.902263625290515));
#70870=CARTESIAN_POINT('Ctrl Pts',(0.0404854078477219,0.233873476118602,
-0.903507465746095));
#70871=CARTESIAN_POINT('Ctrl Pts',(0.0494850752401278,0.232135884354093,
-0.904088180041554));
#70872=CARTESIAN_POINT('Ctrl Pts',(0.0604810905426268,0.229344288161047,
-0.904828284488241));
#70873=CARTESIAN_POINT('Ctrl Pts',(0.0625935115543583,0.228776783373871,
-0.904971868424185));
#70874=CARTESIAN_POINT('Ctrl Pts',(0.0659551457550852,0.227823632645041,
-0.905202756304612));
#70875=CARTESIAN_POINT('Ctrl Pts',(0.0672095761349562,0.227456724681438,
-0.90528945134025));
#70876=CARTESIAN_POINT('Ctrl Pts',(0.0695833611387194,0.226741065846799,
-0.905454556972059));
#70877=CARTESIAN_POINT('Ctrl Pts',(0.0707032910172304,0.226394345430478,
-0.905532899086215));
#70878=CARTESIAN_POINT('Ctrl Pts',(0.0732477607157296,0.225585878609355,
-0.905711933990074));
#70879=CARTESIAN_POINT('Ctrl Pts',(0.0746705783162725,0.22511891886867,
-0.905812795514403));
#70880=CARTESIAN_POINT('Ctrl Pts',(0.0790400158785356,0.223638916805066,
-0.906124905055433));
#70881=CARTESIAN_POINT('Ctrl Pts',(0.0819710668511112,0.222581292584412,
-0.906337611570714));
#70882=CARTESIAN_POINT('Ctrl Pts',(0.101488411795579,0.215100973646811,
-0.907777210647533));
#70883=CARTESIAN_POINT('Ctrl Pts',(0.117324808009818,0.20688882552848,-0.909065324755007));
#70884=CARTESIAN_POINT('Ctrl Pts',(0.135621469890837,0.194619779130859,
-0.91067429562498));
#70885=CARTESIAN_POINT('Ctrl Pts',(0.139086954137596,0.192158428194524,
-0.910984664934843));
#70886=CARTESIAN_POINT('Ctrl Pts',(0.147679127347507,0.18570158644759,-0.911766095433172));
#70887=CARTESIAN_POINT('Ctrl Pts',(0.152711535056764,0.181585798745035,
-0.912235051338868));
#70888=CARTESIAN_POINT('Ctrl Pts',(0.160294678541035,0.17484535251084,-0.912952826428152));
#70889=CARTESIAN_POINT('Ctrl Pts',(0.162964447699258,0.172359721674602,
-0.913207836636389));
#70890=CARTESIAN_POINT('Ctrl Pts',(0.166372684963927,0.169036529986393,
-0.913535263988172));
#70891=CARTESIAN_POINT('Ctrl Pts',(0.167163917661775,0.168254104041823,
-0.913611413858016));
#70892=CARTESIAN_POINT('Ctrl Pts',(0.16844694644382,0.166967370849943,-0.913735075645796));
#70893=CARTESIAN_POINT('Ctrl Pts',(0.16894204322303,0.166466401293174,-0.913782838984906));
#70894=CARTESIAN_POINT('Ctrl Pts',(0.16990534527678,0.16548294850936,-0.91387584529976));
#70895=CARTESIAN_POINT('Ctrl Pts',(0.170373741176174,0.165000669501783,
-0.913921102363046));
#70896=CARTESIAN_POINT('Ctrl Pts',(0.171418677556239,0.163915567834917,
-0.91402215911227));
#70897=CARTESIAN_POINT('Ctrl Pts',(0.171994107212792,0.16331167603736,-0.914077874104222));
#70898=CARTESIAN_POINT('Ctrl Pts',(0.173991247752349,0.161193488010231,
-0.914271525176473));
#70899=CARTESIAN_POINT('Ctrl Pts',(0.17539629169421,0.15966351008791,-0.91440826679957));
#70900=CARTESIAN_POINT('Ctrl Pts',(0.184821377450756,0.149125768850062,
-0.915330640689937));
#70901=CARTESIAN_POINT('Ctrl Pts',(0.192165335529015,0.139534924322692,
-0.916075523251781));
#70902=CARTESIAN_POINT('Ctrl Pts',(0.204583443620507,0.120465475508186,
-0.917472470051787));
#70903=CARTESIAN_POINT('Ctrl Pts',(0.209805753388142,0.111120894624367,
-0.918123937718689));
#70904=CARTESIAN_POINT('Ctrl Pts',(0.21835970768849,0.0930461625228591,
-0.919369718806663));
#70905=CARTESIAN_POINT('Ctrl Pts',(0.221841045827886,0.0844101290063846,
-0.919959286147717));
#70906=CARTESIAN_POINT('Ctrl Pts',(0.225506072521575,0.0735106569322762,
-0.920709382993452));
#70907=CARTESIAN_POINT('Ctrl Pts',(0.226177180205952,0.0714191014263156,
-0.920853563867372));
#70908=CARTESIAN_POINT('Ctrl Pts',(0.227201701447309,0.0680667390380779,
-0.921085185285922));
#70909=CARTESIAN_POINT('Ctrl Pts',(0.227573902725698,0.0668117713085899,
-0.9211720099789));
#70910=CARTESIAN_POINT('Ctrl Pts',(0.228259620095684,0.0644274786626634,
-0.921337217407301));
#70911=CARTESIAN_POINT('Ctrl Pts',(0.228575191833377,0.0632987817128979,
-0.92141553043871));
#70912=CARTESIAN_POINT('Ctrl Pts',(0.229273975268266,0.0607260802248824,
-0.921594296256433));
#70913=CARTESIAN_POINT('Ctrl Pts',(0.229651931151901,0.0592807126738795,
-0.921694915886843));
#70914=CARTESIAN_POINT('Ctrl Pts',(0.230771441123677,0.054828058816994,
-0.922005515179969));
#70915=CARTESIAN_POINT('Ctrl Pts',(0.231467735635185,0.051809843173654,
-0.92221693297017));
#70916=CARTESIAN_POINT('Ctrl Pts',(0.235816328725352,0.0311179605776463,
-0.923672979373517));
#70917=CARTESIAN_POINT('Ctrl Pts',(0.237499412197457,0.0130942003070141,
-0.924980886126771));
#70918=CARTESIAN_POINT('Ctrl Pts',(0.237040731320142,-0.00891359794742625,
-0.926588607967737));
#70919=CARTESIAN_POINT('Ctrl Pts',(0.236858192349084,-0.012882466804857,
-0.926878652492061));
#70920=CARTESIAN_POINT('Ctrl Pts',(0.236112284008601,-0.0233582713521212,
-0.927642309821164));
#70921=CARTESIAN_POINT('Ctrl Pts',(0.235379691727672,-0.0298501543828239,
-0.928113639368944));
#70922=CARTESIAN_POINT('Ctrl Pts',(0.233820005480452,-0.0399195723492457,
-0.928834569811754));
#70923=CARTESIAN_POINT('Ctrl Pts',(0.23317633530627,-0.0435220347792475,
-0.929090421032869));
#70924=CARTESIAN_POINT('Ctrl Pts',(0.232228258072067,-0.04820018402496,
-0.92941875252416));
#70925=CARTESIAN_POINT('Ctrl Pts',(0.23199930031482,-0.0492904287267528,
-0.92949499035349));
#70926=CARTESIAN_POINT('Ctrl Pts',(0.231612997582235,-0.0510675673676237,
-0.929618758705851));
#70927=CARTESIAN_POINT('Ctrl Pts',(0.23146026149432,-0.0517554293574698,
-0.929666541447195));
#70928=CARTESIAN_POINT('Ctrl Pts',(0.231155848484703,-0.0530980796224711,
-0.929759554835466));
#70929=CARTESIAN_POINT('Ctrl Pts',(0.231004450496414,-0.0537529182126418,
-0.929804799778456));
#70930=CARTESIAN_POINT('Ctrl Pts',(0.230659085670137,-0.0552183068566771,
-0.929905797733753));
#70931=CARTESIAN_POINT('Ctrl Pts',(0.230463623988872,-0.0560285042132525,
-0.929961466372759));
#70932=CARTESIAN_POINT('Ctrl Pts',(0.229767125872025,-0.058850195678461,
-0.930154798252433));
#70933=CARTESIAN_POINT('Ctrl Pts',(0.22924397581814,-0.0608562070148542,
-0.930291272187157));
#70934=CARTESIAN_POINT('Ctrl Pts',(0.225526156661754,-0.0743832543932445,
-0.931206576529402));
#70935=CARTESIAN_POINT('Ctrl Pts',(0.22149018180792,-0.0856568064272036,
-0.931945360217781));
#70936=CARTESIAN_POINT('Ctrl Pts',(0.212414385578742,-0.106013231292959,
-0.933313766200487));
#70937=CARTESIAN_POINT('Ctrl Pts',(0.207596432549409,-0.115162452881432,
-0.933943121080449));
#70938=CARTESIAN_POINT('Ctrl Pts',(0.197111836728112,-0.132263289676667,
-0.935190640158037));
#70939=CARTESIAN_POINT('Ctrl Pts',(0.191521031177732,-0.140236636150888,
-0.935806124119797));
#70940=CARTESIAN_POINT('Ctrl Pts',(0.184071548074278,-0.149581365839802,
-0.936585454645904));
#70941=CARTESIAN_POINT('Ctrl Pts',(0.182661874630053,-0.15129956649896,
-0.936731303705609));
#70942=CARTESIAN_POINT('Ctrl Pts',(0.180380265645049,-0.154002170779592,
-0.936964975076122));
#70943=CARTESIAN_POINT('Ctrl Pts',(0.179523906744151,-0.154999598800187,
-0.937052161959542));
#70944=CARTESIAN_POINT('Ctrl Pts',(0.177889168217858,-0.156871908342234,
-0.937217658990402));
#70945=CARTESIAN_POINT('Ctrl Pts',(0.177112512271686,-0.157748247876709,
-0.937295896048207));
#70946=CARTESIAN_POINT('Ctrl Pts',(0.175336643204878,-0.159722402086563,
-0.937473935853399));
#70947=CARTESIAN_POINT('Ctrl Pts',(0.17433355682885,-0.160816650156586,
-0.937573900328392));
#70948=CARTESIAN_POINT('Ctrl Pts',(0.171240014871982,-0.164128379446678,
-0.937880431710378));
#70949=CARTESIAN_POINT('Ctrl Pts',(0.169117106064412,-0.166314973956369,
-0.93808838259582));
#70950=CARTESIAN_POINT('Ctrl Pts',(0.153723388880565,-0.181570961590509,
-0.939580208981506));
#70951=CARTESIAN_POINT('Ctrl Pts',(0.138998050013537,-0.193075566900732,
-0.940932097277406));
#70952=CARTESIAN_POINT('Ctrl Pts',(0.120169865004178,-0.204506227491978,
-0.942540648653914));
#70953=CARTESIAN_POINT('Ctrl Pts',(0.117219085135308,-0.206211736119834,
-0.942789348548752));
#70954=CARTESIAN_POINT('Ctrl Pts',(0.108470413237395,-0.211019858714152,
-0.943515336048037));
#70955=CARTESIAN_POINT('Ctrl Pts',(0.102578675609848,-0.213945876994352,
-0.943990026136453));
#70956=CARTESIAN_POINT('Ctrl Pts',(0.0943143489417772,-0.217630184991644,
-0.944630302189163));
#70957=CARTESIAN_POINT('Ctrl Pts',(0.0920403978783554,-0.218601601234483,
-0.944803888317525));
#70958=CARTESIAN_POINT('Ctrl Pts',(0.0880698977227582,-0.220224827040807,
-0.945102036667528));
#70959=CARTESIAN_POINT('Ctrl Pts',(0.0863803108074465,-0.220893014237281,
-0.945227379437528));
#70960=CARTESIAN_POINT('Ctrl Pts',(0.0838880503226851,-0.221845667501571,
-0.945409861681743));
#70961=CARTESIAN_POINT('Ctrl Pts',(0.0830913053079532,-0.222145313286607,
-0.945467840780107));
#70962=CARTESIAN_POINT('Ctrl Pts',(0.0816767430518859,-0.222668637101217,
-0.945570123309403));
#70963=CARTESIAN_POINT('Ctrl Pts',(0.0810595901001707,-0.222894044771368,
-0.945614526701023));
#70964=CARTESIAN_POINT('Ctrl Pts',(0.0797158809203744,-0.223378499169898,
-0.945710722059338));
#70965=CARTESIAN_POINT('Ctrl Pts',(0.0789889929723276,-0.223636568105714,
-0.94576245659595));
#70966=CARTESIAN_POINT('Ctrl Pts',(0.0769578537991184,-0.224346550219677,
-0.94590620885446));
#70967=CARTESIAN_POINT('Ctrl Pts',(0.0756508718645457,-0.224790639636685,
-0.945997782050744));
#70968=CARTESIAN_POINT('Ctrl Pts',(0.0679709130172216,-0.227325583848626,
-0.946530871254124));
#70969=CARTESIAN_POINT('Ctrl Pts',(0.0615147943001458,-0.229156965023907,
-0.946958932703432));
#70970=CARTESIAN_POINT('Ctrl Pts',(0.0425628447169863,-0.233674064546939,
-0.94818102258841));
#70971=CARTESIAN_POINT('Ctrl Pts',(0.0299170545174869,-0.235627178748956,
-0.948954790919051));
#70972=CARTESIAN_POINT('Ctrl Pts',(0.00455840076217602,-0.23746835211797,
-0.950518932029374));
#70973=CARTESIAN_POINT('Ctrl Pts',(-0.00810964606314755,-0.237373485922798,
-0.951306786860958));
#70974=CARTESIAN_POINT('Ctrl Pts',(-0.0235052764053285,-0.236024073138651,
-0.95230879777316));
#70975=CARTESIAN_POINT('Ctrl Pts',(-0.0262971030402953,-0.235729341411989,
-0.95249223432027));
#70976=CARTESIAN_POINT('Ctrl Pts',(-0.0305093869968351,-0.235208893797576,
-0.952771931227015));
#70977=CARTESIAN_POINT('Ctrl Pts',(-0.0319341677832795,-0.235019691070726,
-0.952867045352051));
#70978=CARTESIAN_POINT('Ctrl Pts',(-0.0345125437591595,-0.234653418693272,
-0.953040132162558));
#70979=CARTESIAN_POINT('Ctrl Pts',(-0.0356667273097581,-0.234480760533774,
-0.953117963171087));
#70980=CARTESIAN_POINT('Ctrl Pts',(-0.0381498545167648,-0.23409054354817,
-0.95328618760446));
#70981=CARTESIAN_POINT('Ctrl Pts',(-0.0394783079627051,-0.233870171353125,
-0.953376667707197));
#70982=CARTESIAN_POINT('Ctrl Pts',(-0.0430791132751796,-0.23324129340404,
-0.953623260599664));
#70983=CARTESIAN_POINT('Ctrl Pts',(-0.0453474429961468,-0.232810909764799,
-0.953780061256431));
#70984=CARTESIAN_POINT('Ctrl Pts',(-0.0579202964877048,-0.230234674793777,
-0.954657577256476));
#70985=CARTESIAN_POINT('Ctrl Pts',(-0.0680779628848821,-0.227438125226631,
-0.955398826434814));
#70986=CARTESIAN_POINT('Ctrl Pts',(-0.0935899451340671,-0.218551838399711,
-0.957341115739239));
#70987=CARTESIAN_POINT('Ctrl Pts',(-0.108555294300177,-0.211517587295821,
-0.958561658576663));
#70988=CARTESIAN_POINT('Ctrl Pts',(-0.127874261312718,-0.199842781203762,
-0.960182906412191));
#70989=CARTESIAN_POINT('Ctrl Pts',(-0.132956690940827,-0.196498082804704,
-0.960613718117229));
#70990=CARTESIAN_POINT('Ctrl Pts',(-0.138969314717727,-0.192200989555981,
-0.96112375663454));
#70991=CARTESIAN_POINT('Ctrl Pts',(-0.140026995637415,-0.191431793357643,
-0.961213490212237));
#70992=CARTESIAN_POINT('Ctrl Pts',(-0.14167898339549,-0.190209370689018,
-0.961353596017911));
#70993=CARTESIAN_POINT('Ctrl Pts',(-0.142277583313108,-0.189762030869195,
-0.961404353337906));
#70994=CARTESIAN_POINT('Ctrl Pts',(-0.143401970381736,-0.18891345352853,
-0.961499659026405));
#70995=CARTESIAN_POINT('Ctrl Pts',(-0.143928190488795,-0.188512848442116,
-0.961544246149591));
#70996=CARTESIAN_POINT('Ctrl Pts',(-0.145146637811149,-0.187577182968247,
-0.961647459769384));
#70997=CARTESIAN_POINT('Ctrl Pts',(-0.145837588595359,-0.187040487199312,
-0.961705970887468));
#70998=CARTESIAN_POINT('Ctrl Pts',(-0.14809659034468,-0.185265679869789,
-0.96189726505498));
#70999=CARTESIAN_POINT('Ctrl Pts',(-0.149652018717732,-0.184011538098165,
-0.962028975795085));
#71000=CARTESIAN_POINT('Ctrl Pts',(-0.163184060984271,-0.172815556800203,
-0.963176686354874));
#71001=CARTESIAN_POINT('Ctrl Pts',(-0.174172574861356,-0.161735307621267,
-0.964123156633538));
#71002=CARTESIAN_POINT('Ctrl Pts',(-0.192878880287221,-0.138736626027903,
-0.965940364174387));
#71003=CARTESIAN_POINT('Ctrl Pts',(-0.200770081893458,-0.127048921675544,
-0.966806396292655));
#71004=CARTESIAN_POINT('Ctrl Pts',(-0.209432803016603,-0.111375851952022,
-0.967957522600417));
#71005=CARTESIAN_POINT('Ctrl Pts',(-0.211205691895818,-0.107976073297876,
-0.968206502517116));
#71006=CARTESIAN_POINT('Ctrl Pts',(-0.213611330031101,-0.103076764245542,
-0.968565082982564));
#71007=CARTESIAN_POINT('Ctrl Pts',(-0.214312315697623,-0.101611272827068,
-0.968672313312657));
#71008=CARTESIAN_POINT('Ctrl Pts',(-0.215500954733855,-0.0990592608693048,
-0.96885905256649));
#71009=CARTESIAN_POINT('Ctrl Pts',(-0.215995587462027,-0.0979760417834671,
-0.968938317680023));
#71010=CARTESIAN_POINT('Ctrl Pts',(-0.21693233594426,-0.0958830396748749,
-0.969091500454952));
#71011=CARTESIAN_POINT('Ctrl Pts',(-0.217375611252159,-0.094873806907852,
-0.969165375882945));
#71012=CARTESIAN_POINT('Ctrl Pts',(-0.218525319312046,-0.0922058341951418,
-0.969360721377472));
#71013=CARTESIAN_POINT('Ctrl Pts',(-0.219219890042996,-0.0905420926222624,
-0.969482590404888));
#71014=CARTESIAN_POINT('Ctrl Pts',(-0.221643848481839,-0.0845444158636322,
-0.969922203026356));
#71015=CARTESIAN_POINT('Ctrl Pts',(-0.223264120855246,-0.0801678291482114,
-0.970243547301865));
#71016=CARTESIAN_POINT('Ctrl Pts',(-0.230550808716873,-0.0585468673434822,
-0.971834709272483));
#71017=CARTESIAN_POINT('Ctrl Pts',(-0.234353117220915,-0.0407409133868043,
-0.973162881150796));
#71018=CARTESIAN_POINT('Ctrl Pts',(-0.236815238704013,-0.0151108211956559,
-0.975040153881166));
#71019=CARTESIAN_POINT('Ctrl Pts',(-0.237177979124535,-0.00751103452780264,
-0.975591560863526));
#71020=CARTESIAN_POINT('Ctrl Pts',(-0.23717341925525,0.00405703612768345,
-0.976412327064179));
#71021=CARTESIAN_POINT('Ctrl Pts',(-0.237072501648943,0.00802021022546458,
-0.976690172081095));
#71022=CARTESIAN_POINT('Ctrl Pts',(-0.23681222175655,0.0131668618294169,
-0.977045118598729));
#71023=CARTESIAN_POINT('Ctrl Pts',(-0.236743229618205,0.0143540239169615,
-0.977126585744526));
#71024=CARTESIAN_POINT('Ctrl Pts',(-0.236618055843411,0.0162602694370274,
-0.977256691299954));
#71025=CARTESIAN_POINT('Ctrl Pts',(-0.236567519063765,0.0169796841155333,
-0.977305630899871));
#71026=CARTESIAN_POINT('Ctrl Pts',(-0.236463665996791,0.0183674944257257,
-0.977399712172109));
#71027=CARTESIAN_POINT('Ctrl Pts',(-0.236410796068062,0.0190359055978749,
-0.977444876293001));
#71028=CARTESIAN_POINT('Ctrl Pts',(-0.236276304141768,0.0206491671213104,
-0.977553542393236));
#71029=CARTESIAN_POINT('Ctrl Pts',(-0.236191847094369,0.0215937825472487,
-0.977616887838891));
#71030=CARTESIAN_POINT('Ctrl Pts',(-0.23587539342549,0.0249088785907314,
-0.977838286255811));
#71031=CARTESIAN_POINT('Ctrl Pts',(-0.235613349289118,0.0272764397316798,
-0.977994767868042));
#71032=CARTESIAN_POINT('Ctrl Pts',(-0.234873154622818,0.0331529851254552,
-0.978379998279816));
#71033=CARTESIAN_POINT('Ctrl Pts',(-0.234351991205659,0.0366560516767475,
-0.978606813908757));
#71034=CARTESIAN_POINT('Ctrl Pts',(-0.231694589361973,0.0521288149137847,
-0.979601275661725));
#71035=CARTESIAN_POINT('Ctrl Pts',(-0.228718167234694,0.0639362140585172,
-0.980341240432557));
#71036=CARTESIAN_POINT('Ctrl Pts',(-0.22029906712413,0.0890213911591812,
-0.98196390218881));
#71037=CARTESIAN_POINT('Ctrl Pts',(-0.214532710494641,0.102137819548313,
-0.982846475214743));
#71038=CARTESIAN_POINT('Ctrl Pts',(-0.206066284837678,0.117469173681874,
-0.983977904960187));
#71039=CARTESIAN_POINT('Ctrl Pts',(-0.204454805785503,0.120252032366676,
-0.984187477297886));
#71040=CARTESIAN_POINT('Ctrl Pts',(-0.202009423067353,0.124283641202035,
-0.984497783625189));
#71041=CARTESIAN_POINT('Ctrl Pts',(-0.201219401356263,0.125558682784296,
-0.984596925679337));
#71042=CARTESIAN_POINT('Ctrl Pts',(-0.199788645343749,0.127819639217326,
-0.984774575967432));
#71043=CARTESIAN_POINT('Ctrl Pts',(-0.199152567878596,0.128808453138365,
-0.984852910233782));
#71044=CARTESIAN_POINT('Ctrl Pts',(-0.197802024741819,0.130874021185105,
-0.985017917780456));
#71045=CARTESIAN_POINT('Ctrl Pts',(-0.197086060533356,0.131949744379605,
-0.985104645390105));
#71046=CARTESIAN_POINT('Ctrl Pts',(-0.19517277257943,0.134774109871154,
-0.985334491345755));
#71047=CARTESIAN_POINT('Ctrl Pts',(-0.193960763210803,0.136512613607017,
-0.985478161702391));
#71048=CARTESIAN_POINT('Ctrl Pts',(-0.187952134022555,0.144889800166391,
-0.98618140782895));
#71049=CARTESIAN_POINT('Ctrl Pts',(-0.182837651666947,0.151292512650184,
-0.986753136973753));
#71050=CARTESIAN_POINT('Ctrl Pts',(-0.171006308713623,0.164625947888223,
-0.988021253903538));
#71051=CARTESIAN_POINT('Ctrl Pts',(-0.164176844776914,0.171437443073787,
-0.988720780043092));
#71052=CARTESIAN_POINT('Ctrl Pts',(-0.146098651911036,0.1873946586456,-0.990480792377981));
#71053=CARTESIAN_POINT('Ctrl Pts',(-0.134389409107557,0.195962074328455,
-0.991543566052026));
#71054=CARTESIAN_POINT('Ctrl Pts',(-0.120206017873164,0.204466939118223,
-0.992696362932122));
#71055=CARTESIAN_POINT('Ctrl Pts',(-0.118427250529332,0.205502318665864,
-0.992838653405654));
#71056=CARTESIAN_POINT('Ctrl Pts',(-0.115933143261656,0.206910939637112,
-0.993034777413625));
#71057=CARTESIAN_POINT('Ctrl Pts',(-0.115229098919506,0.207303848150714,
-0.993089768922433));
#71058=CARTESIAN_POINT('Ctrl Pts',(-0.113940556034504,0.208014357150275,
-0.99318972040096));
#71059=CARTESIAN_POINT('Ctrl Pts',(-0.113356698997806,0.208333103290601,
-0.993234751479036));
#71060=CARTESIAN_POINT('Ctrl Pts',(-0.112141232300572,0.208990042608169,
-0.99332795060113));
#71061=CARTESIAN_POINT('Ctrl Pts',(-0.111509421706876,0.209327835694194,
-0.993376093772336));
#71062=CARTESIAN_POINT('Ctrl Pts',(-0.109843883916734,0.210208622987748,
-0.993502237787409));
#71063=CARTESIAN_POINT('Ctrl Pts',(-0.108807644909484,0.210746863704373,
-0.993579946470265));
#71064=CARTESIAN_POINT('Ctrl Pts',(-0.104029808169605,0.213183921150094,
-0.993934897645398));
#71065=CARTESIAN_POINT('Ctrl Pts',(-0.10024195600675,0.214991024718669,
-0.994206940668382));
#71066=CARTESIAN_POINT('Ctrl Pts',(-0.08901178210802,0.219987301671365,
-0.994992187864485));
#71067=CARTESIAN_POINT('Ctrl Pts',(-0.0814514880749731,0.22289725267806,
-0.995494193889456));
#71068=CARTESIAN_POINT('Ctrl Pts',(-0.0633377977123513,0.228824121685867,
-0.996666873125569));
#71069=CARTESIAN_POINT('Ctrl Pts',(-0.0527062750104053,0.231503131401166,
-0.997332618169306));
#71070=CARTESIAN_POINT('Ctrl Pts',(-0.0419392532630309,0.233437528389801,
-0.998011590250681));
#71071=CARTESIAN_POINT('Ctrl Pts',(-0.0419392742985056,0.233437524610579,
-1.01798096863704));
#71072=CARTESIAN_POINT('Ctrl Pts',(-0.0422632750598508,0.233379314788377,
-1.01796023613685));
#71073=CARTESIAN_POINT('Ctrl Pts',(-0.0425871672563835,0.233320428150497,
-1.01793948734342));
#71074=CARTESIAN_POINT('Ctrl Pts',(-0.0473194747750942,0.232449867177383,
-1.01763598461243));
#71075=CARTESIAN_POINT('Ctrl Pts',(-0.0517039011818453,0.231514095318814,
-1.01735036103975));
#71076=CARTESIAN_POINT('Ctrl Pts',(-0.0592873197805651,0.22966939969849,
-1.01684661972613));
#71077=CARTESIAN_POINT('Ctrl Pts',(-0.0624986542337207,0.228816380287551,
-1.01663021966578));
#71078=CARTESIAN_POINT('Ctrl Pts',(-0.0671663671439948,0.227470916108471,
-1.0163106386793));
#71079=CARTESIAN_POINT('Ctrl Pts',(-0.0686376517744219,0.227031299875507,
-1.01620916568142));
#71080=CARTESIAN_POINT('Ctrl Pts',(-0.0712287148892143,0.226229608063533,
-1.01602910377622));
#71081=CARTESIAN_POINT('Ctrl Pts',(-0.0723502724684468,0.225873423353623,
-1.01595070975655));
#71082=CARTESIAN_POINT('Ctrl Pts',(-0.0746923032457631,0.225110407255202,
-1.01578603468581));
#71083=CARTESIAN_POINT('Ctrl Pts',(-0.0759122066295384,0.224701963476534,
-1.01569970269944));
#71084=CARTESIAN_POINT('Ctrl Pts',(-0.0791090446185606,0.223602605549567,
-1.01547196511786));
#71085=CARTESIAN_POINT('Ctrl Pts',(-0.0810802188927643,0.222895409917599,
-1.01533002530775));
#71086=CARTESIAN_POINT('Ctrl Pts',(-0.0896255789672378,0.219701251374851,
-1.01470788662115));
#71087=CARTESIAN_POINT('Ctrl Pts',(-0.0960961343688778,0.216949071271681,
-1.01421896402477));
#71088=CARTESIAN_POINT('Ctrl Pts',(-0.116885251584624,0.206994033960744,
-1.01258795180993));
#71089=CARTESIAN_POINT('Ctrl Pts',(-0.130596445140514,0.198628173673593,
-1.01141158036202));
#71090=CARTESIAN_POINT('Ctrl Pts',(-0.148937457192227,0.184712392760167,
-1.00973525680361));
#71091=CARTESIAN_POINT('Ctrl Pts',(-0.15432719730745,0.180233635958996,
-1.00922862296121));
#71092=CARTESIAN_POINT('Ctrl Pts',(-0.16234499092282,0.172947240356999,
-1.00846109676939));
#71093=CARTESIAN_POINT('Ctrl Pts',(-0.165116290032456,0.170303431902368,
-1.00819304784337));
#71094=CARTESIAN_POINT('Ctrl Pts',(-0.168622161676673,0.166792768966254,
-1.00785166048578));
#71095=CARTESIAN_POINT('Ctrl Pts',(-0.169416070386828,0.165986313929055,
-1.00777419554823));
#71096=CARTESIAN_POINT('Ctrl Pts',(-0.170697487361878,0.164665874277494,
-1.00764895093927));
#71097=CARTESIAN_POINT('Ctrl Pts',(-0.171188507094944,0.164155345375798,
-1.0076009077662));
#71098=CARTESIAN_POINT('Ctrl Pts',(-0.172139045734287,0.163158136612783,
-1.007507817032));
#71099=CARTESIAN_POINT('Ctrl Pts',(-0.172598801116911,0.162671701525592,
-1.00746275224699));
#71100=CARTESIAN_POINT('Ctrl Pts',(-0.17372603000911,0.161468900399427,
-1.0073521475783));
#71101=CARTESIAN_POINT('Ctrl Pts',(-0.174391148484324,0.160750324147314,
-1.00728678514286));
#71102=CARTESIAN_POINT('Ctrl Pts',(-0.176308383773,0.15865308941284,-1.00709800823569));
#71103=CARTESIAN_POINT('Ctrl Pts',(-0.177548768929553,0.15726374070451,
-1.00697541594042));
#71104=CARTESIAN_POINT('Ctrl Pts',(-0.188198145901443,0.145048807572277,
-1.00591733091284));
#71105=CARTESIAN_POINT('Ctrl Pts',(-0.196624849652758,0.133403456028322,
-1.00504051789584));
#71106=CARTESIAN_POINT('Ctrl Pts',(-0.208910129077674,0.112707710516761,
-1.00356551431451));
#71107=CARTESIAN_POINT('Ctrl Pts',(-0.213353283056393,0.104052072676631,
-1.0029702915832));
#71108=CARTESIAN_POINT('Ctrl Pts',(-0.220553071413563,0.0876128100012291,
-1.00184685787184));
#71109=CARTESIAN_POINT('Ctrl Pts',(-0.223458837487953,0.0799111213121292,
-1.00132325796295));
#71110=CARTESIAN_POINT('Ctrl Pts',(-0.226603190950512,0.0700533768727471,
-1.00064775456286));
#71111=CARTESIAN_POINT('Ctrl Pts',(-0.22722074820045,0.0680236199171196,
-1.0005084062185));
#71112=CARTESIAN_POINT('Ctrl Pts',(-0.228170550501307,0.0647445045977041,
-1.000282741197));
#71113=CARTESIAN_POINT('Ctrl Pts',(-0.228519965163453,0.0635002078815756,
-1.00019698524257));
#71114=CARTESIAN_POINT('Ctrl Pts',(-0.229167638749663,0.0611191865430806,
-1.00003261998377));
#71115=CARTESIAN_POINT('Ctrl Pts',(-0.229467653717758,0.0599829761287445,
-0.999954070378719));
#71116=CARTESIAN_POINT('Ctrl Pts',(-0.230130903694588,0.0573933113487352,
-0.999774754521618));
#71117=CARTESIAN_POINT('Ctrl Pts',(-0.2304888327643,0.0559385628560676,
-0.999673820441227));
#71118=CARTESIAN_POINT('Ctrl Pts',(-0.231569691542354,0.0513589868288608,
-0.999355388131359));
#71119=CARTESIAN_POINT('Ctrl Pts',(-0.232243005732384,0.0482229416530763,
-0.999136318961076));
#71120=CARTESIAN_POINT('Ctrl Pts',(-0.235741875918895,0.0301478970315594,
-0.99786730918976));
#71121=CARTESIAN_POINT('Ctrl Pts',(-0.23718885865161,0.0149807892051603,
-0.99677423853755));
#71122=CARTESIAN_POINT('Ctrl Pts',(-0.237160804066701,-0.0155658577260233,
-0.994546359668472));
#71123=CARTESIAN_POINT('Ctrl Pts',(-0.235656959168687,-0.0308774600742672,
-0.993416922705108));
#71124=CARTESIAN_POINT('Ctrl Pts',(-0.232295131637977,-0.0479059383490672,
-0.99220773276186));
#71125=CARTESIAN_POINT('Ctrl Pts',(-0.231881496679346,-0.0498696228094154,
-0.992069056025991));
#71126=CARTESIAN_POINT('Ctrl Pts',(-0.231251497611235,-0.0526829502750557,
-0.991871702225889));
#71127=CARTESIAN_POINT('Ctrl Pts',(-0.231055282365642,-0.0535369493875011,
-0.991811970958411));
#71128=CARTESIAN_POINT('Ctrl Pts',(-0.230702670997574,-0.055033586171341,
-0.991707625006668));
#71129=CARTESIAN_POINT('Ctrl Pts',(-0.230548313206057,-0.0556766857324453,
-0.991662897021047));
#71130=CARTESIAN_POINT('Ctrl Pts',(-0.230214100137423,-0.0570438896833402,
-0.991568046389226));
#71131=CARTESIAN_POINT('Ctrl Pts',(-0.230033516827469,-0.057767797491483,
-0.991517965559326));
#71132=CARTESIAN_POINT('Ctrl Pts',(-0.229528177706717,-0.0597536114390435,
-0.991380940869361));
#71133=CARTESIAN_POINT('Ctrl Pts',(-0.229196428287493,-0.0610137352814793,
-0.991294386288601));
#71134=CARTESIAN_POINT('Ctrl Pts',(-0.227277292079897,-0.0680668080809355,
-0.990811823552627));
#71135=CARTESIAN_POINT('Ctrl Pts',(-0.225480532240527,-0.0738010928991041,
-0.990426664875811));
#71136=CARTESIAN_POINT('Ctrl Pts',(-0.219501066704819,-0.0906170137375754,
-0.989301710464295));
#71137=CARTESIAN_POINT('Ctrl Pts',(-0.214704342650741,-0.101460542304057,
-0.988581661577075));
#71138=CARTESIAN_POINT('Ctrl Pts',(-0.201993096294056,-0.12521497060818,
-0.9869287246401));
#71139=CARTESIAN_POINT('Ctrl Pts',(-0.193614532709966,-0.13781627147034,
-0.985994080111688));
#71140=CARTESIAN_POINT('Ctrl Pts',(-0.182585173905853,-0.151394769359509,
-0.984855698777855));
#71141=CARTESIAN_POINT('Ctrl Pts',(-0.181046422256745,-0.15323157057933,
-0.984698714351303));
#71142=CARTESIAN_POINT('Ctrl Pts',(-0.178587195222643,-0.156078378414233,
-0.984450462203051));
#71143=CARTESIAN_POINT('Ctrl Pts',(-0.177685342284982,-0.157104314106395,
-0.984359959979965));
#71144=CARTESIAN_POINT('Ctrl Pts',(-0.176005143178681,-0.15898271154365,
-0.984192296755484));
#71145=CARTESIAN_POINT('Ctrl Pts',(-0.17522933475977,-0.15983739597996,
-0.984115243700795));
#71146=CARTESIAN_POINT('Ctrl Pts',(-0.173493757411195,-0.16172160578393,
-0.983943644413476));
#71147=CARTESIAN_POINT('Ctrl Pts',(-0.172531006784746,-0.162748312394476,
-0.98384897256605));
#71148=CARTESIAN_POINT('Ctrl Pts',(-0.169721164621445,-0.165691860892384,
-0.983574104686601));
#71149=CARTESIAN_POINT('Ctrl Pts',(-0.16785091928829,-0.167586199831108,
-0.983392910382637));
#71150=CARTESIAN_POINT('Ctrl Pts',(-0.163543715356715,-0.17180445416408,
-0.982979375615308));
#71151=CARTESIAN_POINT('Ctrl Pts',(-0.16108839611643,-0.174108713060005,
-0.982746248495182));
#71152=CARTESIAN_POINT('Ctrl Pts',(-0.152744288566874,-0.181611838868939,
-0.981962351513645));
#71153=CARTESIAN_POINT('Ctrl Pts',(-0.146646863960116,-0.186569970889694,
-0.981402701759877));
#71154=CARTESIAN_POINT('Ctrl Pts',(-0.126838149790874,-0.201105693858329,
-0.97962899273299));
#71155=CARTESIAN_POINT('Ctrl Pts',(-0.112353844013378,-0.209542397726592,
-0.97839061099793));
#71156=CARTESIAN_POINT('Ctrl Pts',(-0.0928283945638343,-0.218304426649075,
-0.976864740841788));
#71157=CARTESIAN_POINT('Ctrl Pts',(-0.0884974225334974,-0.220095767430514,
-0.976534964445998));
#71158=CARTESIAN_POINT('Ctrl Pts',(-0.0829399755530145,-0.222203786656368,
-0.976125087641337));
#71159=CARTESIAN_POINT('Ctrl Pts',(-0.0817605003251482,-0.222640479497394,
-0.976038845094655));
#71160=CARTESIAN_POINT('Ctrl Pts',(-0.0798852242868947,-0.223317875375292,
-0.975902968521636));
#71161=CARTESIAN_POINT('Ctrl Pts',(-0.0791917009999208,-0.22356474912591,
-0.975852985742669));
#71162=CARTESIAN_POINT('Ctrl Pts',(-0.0778702180974649,-0.224028237013831,
-0.97575826896684));
#71163=CARTESIAN_POINT('Ctrl Pts',(-0.0772425018772638,-0.224245440890856,
-0.975713503234853));
#71164=CARTESIAN_POINT('Ctrl Pts',(-0.0757510904633691,-0.224754497198856,
-0.975607663183514));
#71165=CARTESIAN_POINT('Ctrl Pts',(-0.0748866124927424,-0.225044011374408,
-0.975546725734796));
#71166=CARTESIAN_POINT('Ctrl Pts',(-0.0719713575833915,-0.226001673176092,
-0.975342541745212));
#71167=CARTESIAN_POINT('Ctrl Pts',(-0.0699130701676077,-0.226646853097484,
-0.975200559821209));
#71168=CARTESIAN_POINT('Ctrl Pts',(-0.0648761958635684,-0.228150535336097,
-0.974857748172062));
#71169=CARTESIAN_POINT('Ctrl Pts',(-0.0618889669489348,-0.228978918793727,
-0.974658346055567));
#71170=CARTESIAN_POINT('Ctrl Pts',(-0.0496557984955409,-0.232114368294907,
-0.973854390514675));
#71171=CARTESIAN_POINT('Ctrl Pts',(-0.0402904612524984,-0.233921963185723,
-0.973267805165594));
#71172=CARTESIAN_POINT('Ctrl Pts',(-0.013140511722014,-0.237482649289191,
-0.971588115014542));
#71173=CARTESIAN_POINT('Ctrl Pts',(0.00476343443951824,-0.237798036803507,
-0.970501087327765));
#71174=CARTESIAN_POINT('Ctrl Pts',(0.0256294445630077,-0.235806680392451,
-0.969145752847856));
#71175=CARTESIAN_POINT('Ctrl Pts',(0.0287201338560649,-0.235450231237663,
-0.96894286461842));
#71176=CARTESIAN_POINT('Ctrl Pts',(0.0332855492847619,-0.234832475645031,
-0.968639582100633));
#71177=CARTESIAN_POINT('Ctrl Pts',(0.0347663322284696,-0.234617819825169,
-0.968540652489463));
#71178=CARTESIAN_POINT('Ctrl Pts',(0.0374030827439788,-0.23421008380084,
-0.968363447729816));
#71179=CARTESIAN_POINT('Ctrl Pts',(0.0385598470780688,-0.23402241786087,
-0.968285346194934));
#71180=CARTESIAN_POINT('Ctrl Pts',(0.0410036341392827,-0.233607342956876,
-0.968119563176141));
#71181=CARTESIAN_POINT('Ctrl Pts',(0.0422902588698042,-0.233377853666517,
-0.968031818023431));
#71182=CARTESIAN_POINT('Ctrl Pts',(0.0457259822764512,-0.232735695528596,
-0.967796237429406));
#71183=CARTESIAN_POINT('Ctrl Pts',(0.0478713325317403,-0.2323039052402,
-0.967647799221991));
#71184=CARTESIAN_POINT('Ctrl Pts',(0.0589868929277687,-0.22990618720785,
-0.96687152110211));
#71185=CARTESIAN_POINT('Ctrl Pts',(0.0678422587878289,-0.227450429768159,
-0.966228215971281));
#71186=CARTESIAN_POINT('Ctrl Pts',(0.0867347737370395,-0.221009622340344,
-0.964801699505761));
#71187=CARTESIAN_POINT('Ctrl Pts',(0.096687818041288,-0.216840054389063,
-0.964015046504671));
#71188=CARTESIAN_POINT('Ctrl Pts',(0.117153519969759,-0.206576523521615,
-0.962342996905235));
#71189=CARTESIAN_POINT('Ctrl Pts',(0.127553886433173,-0.20032192077999,
-0.961459783662889));
#71190=CARTESIAN_POINT('Ctrl Pts',(0.139121343601995,-0.192097713732959,
-0.960469725050554));
#71191=CARTESIAN_POINT('Ctrl Pts',(0.140795473045375,-0.190874082495373,
-0.960326260233319));
#71192=CARTESIAN_POINT('Ctrl Pts',(0.143119696163081,-0.189128072120037,
-0.960127077284734));
#71193=CARTESIAN_POINT('Ctrl Pts',(0.14378335307408,-0.188624024252106,
-0.960070201847991));
#71194=CARTESIAN_POINT('Ctrl Pts',(0.144977289078083,-0.187707266119526,
-0.959967900467953));
#71195=CARTESIAN_POINT('Ctrl Pts',(0.145508496235768,-0.187295781229081,
-0.959922391389542));
#71196=CARTESIAN_POINT('Ctrl Pts',(0.14659287862366,-0.186448396449807,
-0.959829517357495));
#71197=CARTESIAN_POINT('Ctrl Pts',(0.147145872341527,-0.186012281550627,
-0.959782168182981));
#71198=CARTESIAN_POINT('Ctrl Pts',(0.148567881318607,-0.184880513690316,
-0.959660420593631));
#71199=CARTESIAN_POINT('Ctrl Pts',(0.149433968766053,-0.184181184713478,
-0.959586278429204));
#71200=CARTESIAN_POINT('Ctrl Pts',(0.153121109439434,-0.181160844395393,
-0.959270519023305));
#71201=CARTESIAN_POINT('Ctrl Pts',(0.155893427207424,-0.178780783684352,
-0.959032801968887));
#71202=CARTESIAN_POINT('Ctrl Pts',(0.163453716880564,-0.171980548463517,
-0.958380054589196));
#71203=CARTESIAN_POINT('Ctrl Pts',(0.168116387363714,-0.167425563167802,
-0.957972226309055));
#71204=CARTESIAN_POINT('Ctrl Pts',(0.175401344259383,-0.15969720461835,
-0.957314605920151));
#71205=CARTESIAN_POINT('Ctrl Pts',(0.178138859186959,-0.156637724683934,
-0.957062307469217));
#71206=CARTESIAN_POINT('Ctrl Pts',(0.192394688370421,-0.139847849756836,
-0.955711128555238));
#71207=CARTESIAN_POINT('Ctrl Pts',(0.202406772513173,-0.124918175022821,
-0.954620202215843));
#71208=CARTESIAN_POINT('Ctrl Pts',(0.212069582634607,-0.106245570056992,
-0.953260683489908));
#71209=CARTESIAN_POINT('Ctrl Pts',(0.213442780007141,-0.103459205666825,
-0.953058102930902));
#71210=CARTESIAN_POINT('Ctrl Pts',(0.215395371141649,-0.0992927528531827,
-0.952755192476975));
#71211=CARTESIAN_POINT('Ctrl Pts',(0.216017098140839,-0.0979327821360431,
-0.952656321932976));
#71212=CARTESIAN_POINT('Ctrl Pts',(0.217103011861908,-0.0954967850498731,
-0.952479182739508));
#71213=CARTESIAN_POINT('Ctrl Pts',(0.21757216621149,-0.0944230168963909,
-0.952401087211313));
#71214=CARTESIAN_POINT('Ctrl Pts',(0.218547916015378,-0.0921439008375314,
-0.952235274611943));
#71215=CARTESIAN_POINT('Ctrl Pts',(0.21905253813811,-0.0909377560345294,
-0.952147493556511));
#71216=CARTESIAN_POINT('Ctrl Pts',(0.220375945279911,-0.0876996160912122,
-0.951911713440981));
#71217=CARTESIAN_POINT('Ctrl Pts',(0.221176575303429,-0.0856603869688508,
-0.95176310982777));
#71218=CARTESIAN_POINT('Ctrl Pts',(0.225199245897759,-0.0749819690119696,
-0.950984097357312));
#71219=CARTESIAN_POINT('Ctrl Pts',(0.227943338882066,-0.0661724373596597,
-0.950338090622313));
#71220=CARTESIAN_POINT('Ctrl Pts',(0.23276215463758,-0.0467909504527406,
-0.948910530272376));
#71221=CARTESIAN_POINT('Ctrl Pts',(0.234643870559066,-0.0361916739412844,
-0.94812573917053));
#71222=CARTESIAN_POINT('Ctrl Pts',(0.237100979435463,-0.0134725561905994,
-0.9464568731755));
#71223=CARTESIAN_POINT('Ctrl Pts',(0.237479669791776,-0.0013598095768279,
-0.945574978278472));
#71224=CARTESIAN_POINT('Ctrl Pts',(0.236838306904382,0.0128023731972036,
-0.944586050413844));
#71225=CARTESIAN_POINT('Ctrl Pts',(0.236717261995422,0.0148735665785085,
-0.94444250902019));
#71226=CARTESIAN_POINT('Ctrl Pts',(0.236509505708998,0.0177743948449892,
-0.944243237905769));
#71227=CARTESIAN_POINT('Ctrl Pts',(0.236445577289121,0.018605494777037,
-0.944186349579088));
#71228=CARTESIAN_POINT('Ctrl Pts',(0.236322200189586,0.0201059659386397,
-0.944084031909984));
#71229=CARTESIAN_POINT('Ctrl Pts',(0.236264285828072,0.0207754530972834,
-0.944038519350998));
#71230=CARTESIAN_POINT('Ctrl Pts',(0.236139855148863,0.0221459998558341,
-0.943945646638725));
#71231=CARTESIAN_POINT('Ctrl Pts',(0.236073060823819,0.0228470235599321,
-0.943898302206605));
#71232=CARTESIAN_POINT('Ctrl Pts',(0.235892659926479,0.0246550594524117,
-0.943776581278541));
#71233=CARTESIAN_POINT('Ctrl Pts',(0.235774381250001,0.0257616038244113,
-0.943702460819372));
#71234=CARTESIAN_POINT('Ctrl Pts',(0.235234841335179,0.0304938122672807,
-0.943386925731097));
#71235=CARTESIAN_POINT('Ctrl Pts',(0.234737678756236,0.0341105393039,-0.943149404421166));
#71236=CARTESIAN_POINT('Ctrl Pts',(0.23312252522281,0.0441384857335257,
-0.942497373591188));
#71237=CARTESIAN_POINT('Ctrl Pts',(0.231823865979681,0.050517572243762,
-0.942090047033668));
#71238=CARTESIAN_POINT('Ctrl Pts',(0.229264014485041,0.0608885851818783,
-0.941428583205499));
#71239=CARTESIAN_POINT('Ctrl Pts',(0.228156772355307,0.0649145333826267,
-0.941172008810144));
#71240=CARTESIAN_POINT('Ctrl Pts',(0.221755992724638,0.0859946927190393,
-0.939820612327463));
#71241=CARTESIAN_POINT('Ctrl Pts',(0.21465613250109,0.102437625490528,-0.938733384620454));
#71242=CARTESIAN_POINT('Ctrl Pts',(0.204232409683695,0.120626615106908,
-0.937377835292395));
#71243=CARTESIAN_POINT('Ctrl Pts',(0.202632798481718,0.123294788816971,
-0.937174962572818));
#71244=CARTESIAN_POINT('Ctrl Pts',(0.200186804129414,0.127198516986609,
-0.936871698809996));
#71245=CARTESIAN_POINT('Ctrl Pts',(0.199380410858223,0.128458829453395,
-0.936772772175208));
#71246=CARTESIAN_POINT('Ctrl Pts',(0.197921256173277,0.130692502828194,
-0.936595570720357));
#71247=CARTESIAN_POINT('Ctrl Pts',(0.19727309747168,0.131668822695496,-0.93651746948908));
#71248=CARTESIAN_POINT('Ctrl Pts',(0.195886822648927,0.133723750608847,
-0.936351684984267));
#71249=CARTESIAN_POINT('Ctrl Pts',(0.195146975242471,0.13480113760411,-0.936263938026059));
#71250=CARTESIAN_POINT('Ctrl Pts',(0.193144556673796,0.137666082180563,
-0.936028347398848));
#71251=CARTESIAN_POINT('Ctrl Pts',(0.19186611102136,0.139442335167609,-0.935879900873936));
#71252=CARTESIAN_POINT('Ctrl Pts',(0.18509513999362,0.148580389047212,-0.935103485643365));
#71253=CARTESIAN_POINT('Ctrl Pts',(0.179203618055949,0.155635367887134,
-0.934460045082522));
#71254=CARTESIAN_POINT('Ctrl Pts',(0.165541784759199,0.170188318229843,
-0.933033475763687));
#71255=CARTESIAN_POINT('Ctrl Pts',(0.157638376022508,0.177533821537695,
-0.932246915570011));
#71256=CARTESIAN_POINT('Ctrl Pts',(0.139847595845537,0.191941230324709,
-0.930575025435195));
#71257=CARTESIAN_POINT('Ctrl Pts',(0.129860184425608,0.198834546880914,
-0.929691878683497));
#71258=CARTESIAN_POINT('Ctrl Pts',(0.117597138135601,0.205978623132566,
-0.928701877267359));
#71259=CARTESIAN_POINT('Ctrl Pts',(0.115791797110284,0.206998890187272,
-0.928558408743856));
#71260=CARTESIAN_POINT('Ctrl Pts',(0.113242403523329,0.208395856851519,
-0.928359221527935));
#71261=CARTESIAN_POINT('Ctrl Pts',(0.112509454963556,0.208792475211763,
-0.928302345467193));
#71262=CARTESIAN_POINT('Ctrl Pts',(0.111181789978038,0.209501889449674,
-0.928200043298646));
#71263=CARTESIAN_POINT('Ctrl Pts',(0.110587806970969,0.209816036316492,
-0.92815453405178));
#71264=CARTESIAN_POINT('Ctrl Pts',(0.109368542918671,0.210454266805773,
-0.928061660083809));
#71265=CARTESIAN_POINT('Ctrl Pts',(0.108743140915312,0.210778096427793,
-0.928014311139019));
#71266=CARTESIAN_POINT('Ctrl Pts',(0.107125553759385,0.211606558021915,
-0.927892564841113));
#71267=CARTESIAN_POINT('Ctrl Pts',(0.106131227891892,0.2121070066123,-0.927818423728058));
#71268=CARTESIAN_POINT('Ctrl Pts',(0.101858944189285,0.214219700527968,
-0.927502675191723));
#71269=CARTESIAN_POINT('Ctrl Pts',(0.0985473039358211,0.215763196712221,
-0.927264967622557));
#71270=CARTESIAN_POINT('Ctrl Pts',(0.0892343110721986,0.219844624805761,
-0.926612254974379));
#71271=CARTESIAN_POINT('Ctrl Pts',(0.0831618549986136,0.222212824765676,
-0.926204451014928));
#71272=CARTESIAN_POINT('Ctrl Pts',(0.0731135138158255,0.225661853215844,
-0.925546634472915));
#71273=CARTESIAN_POINT('Ctrl Pts',(0.0691937742389778,0.226894426384592,
-0.925294119016022));
#71274=CARTESIAN_POINT('Ctrl Pts',(0.0480177070501756,0.232953465762329,
-0.923942931490136));
#71275=CARTESIAN_POINT('Ctrl Pts',(0.0302905814593938,0.235913994694997,
-0.922852194973547));
#71276=CARTESIAN_POINT('Ctrl Pts',(0.00929778192120318,0.237013041345022,
-0.921492879808453));
#71277=CARTESIAN_POINT('Ctrl Pts',(0.00619283613492947,0.237114482550914,
-0.92129028400685));
#71278=CARTESIAN_POINT('Ctrl Pts',(0.00159164458882926,0.237174373576065,
-0.92098735511916));
#71279=CARTESIAN_POINT('Ctrl Pts',(9.62610957998343E-5,0.237179694272432,
-0.920888481647647));
#71280=CARTESIAN_POINT('Ctrl Pts',(-0.00257081801484389,0.237163961471575,
-0.920711339205475));
#71281=CARTESIAN_POINT('Ctrl Pts',(-0.00374250585806567,0.237148365567761,
-0.920633243380491));
#71282=CARTESIAN_POINT('Ctrl Pts',(-0.00622115791677948,0.237096999523045,
-0.920467432251684));
#71283=CARTESIAN_POINT('Ctrl Pts',(-0.00752803400164977,0.237059103545626,
-0.920379652979261));
#71284=CARTESIAN_POINT('Ctrl Pts',(-0.011023597810831,0.23692880721959,
-0.920143882772886));
#71285=CARTESIAN_POINT('Ctrl Pts',(-0.0132113858183241,0.236816887324553,
-0.919995287374625));
#71286=CARTESIAN_POINT('Ctrl Pts',(-0.0242996886663794,0.236095520178203,
-0.919236704472944));
#71287=CARTESIAN_POINT('Ctrl Pts',(-0.0331610130045195,0.235014622843947,
-0.918612203568901));
#71288=CARTESIAN_POINT('Ctrl Pts',(-0.0419392742314872,0.23343752462262,
-0.917975447697368));
#71289=CARTESIAN_POINT('Origin',(0.,0.,-2.1456589891905));
#71290=CARTESIAN_POINT('',(-0.0419215622832511,0.233346034556857,-0.798097588861634));
#71291=CARTESIAN_POINT('',(-0.0419392746656718,0.233437524544614,-0.817620397237267));
#71292=CARTESIAN_POINT('',(-0.0419392741328076,0.233437524640348,-2.1456589891905));
#71293=CARTESIAN_POINT('',(-0.236887575109366,0.0001513332746742,-0.875941010809498));
#71294=CARTESIAN_POINT('Ctrl Pts',(-0.236887575109366,0.0001513332746742,
-0.875941010809498));
#71295=CARTESIAN_POINT('Ctrl Pts',(-0.236597463890264,-0.049544091138451,
-0.872615461822126));
#71296=CARTESIAN_POINT('Ctrl Pts',(-0.197039124271961,-0.178782761335024,
-0.863995269476757));
#71297=CARTESIAN_POINT('Ctrl Pts',(0.0151527372976048,-0.279961252852672,
-0.850080433773393));
#71298=CARTESIAN_POINT('Ctrl Pts',(0.243491146154017,-0.138996295961623,
-0.834196503699405));
#71299=CARTESIAN_POINT('Ctrl Pts',(0.248777094918733,0.129297585399898,
-0.818312573625418));
#71300=CARTESIAN_POINT('Ctrl Pts',(0.0801384244127168,0.242817063678148,
-0.806279602012826));
#71301=CARTESIAN_POINT('Ctrl Pts',(-0.0207684499901398,0.237356879304441,
-0.799541273758231));
#71302=CARTESIAN_POINT('Ctrl Pts',(-0.0419215622832843,0.23334603455685,
-0.798097588861632));
#71303=CARTESIAN_POINT('Ctrl Pts',(-0.237174943862191,0.000163183843552357,
-0.875775716082648));
#71304=CARTESIAN_POINT('Ctrl Pts',(-0.237164001431015,0.0160671510705129,
-0.876898264731405));
#71305=CARTESIAN_POINT('Ctrl Pts',(-0.23555337892694,0.0319287061283791,
-0.878063892272444));
#71306=CARTESIAN_POINT('Ctrl Pts',(-0.230191123282688,0.05815630739297,
-0.880015174976474));
#71307=CARTESIAN_POINT('Ctrl Pts',(-0.227284381721771,0.06864383126262,
-0.880800959270579));
#71308=CARTESIAN_POINT('Ctrl Pts',(-0.22317710950521,0.0802878359840086,
-0.881655268879182));
#71309=CARTESIAN_POINT('Ctrl Pts',(-0.222673166825975,0.0816750871891151,
-0.881756738959431));
#71310=CARTESIAN_POINT('Ctrl Pts',(-0.221881986312466,0.0837912783102711,
-0.881910953095896));
#71311=CARTESIAN_POINT('Ctrl Pts',(-0.221604043232464,0.0845236194126831,
-0.881964215306016));
#71312=CARTESIAN_POINT('Ctrl Pts',(-0.221086712469624,0.0858666196223114,
-0.882061677303563));
#71313=CARTESIAN_POINT('Ctrl Pts',(-0.220848419197361,0.086477665059888,
-0.882105937922297));
#71314=CARTESIAN_POINT('Ctrl Pts',(-0.220300894102182,0.0878646362973995,
-0.882206218569208));
#71315=CARTESIAN_POINT('Ctrl Pts',(-0.219990095949804,0.088639923236142,
-0.882262144307547));
#71316=CARTESIAN_POINT('Ctrl Pts',(-0.219167969423675,0.0906597600180472,
-0.88240754970554));
#71317=CARTESIAN_POINT('Ctrl Pts',(-0.218650126633838,0.0919016498037438,
-0.882496656322477));
#71318=CARTESIAN_POINT('Ctrl Pts',(-0.21346446456841,0.104045911106359,
-0.883365749288355));
#71319=CARTESIAN_POINT('Ctrl Pts',(-0.207994990040098,0.114589673315482,
-0.884102710142617));
#71320=CARTESIAN_POINT('Ctrl Pts',(-0.194505403633626,0.136418491898445,
-0.885681107506964));
#71321=CARTESIAN_POINT('Ctrl Pts',(-0.186242013125466,0.147500012570092,
-0.886517886675148));
#71322=CARTESIAN_POINT('Ctrl Pts',(-0.173704334038675,0.161568122803833,
-0.887701048702306));
#71323=CARTESIAN_POINT('Ctrl Pts',(-0.170227095552165,0.165227675753513,
-0.88802134979542));
#71324=CARTESIAN_POINT('Ctrl Pts',(-0.164856467158617,0.170530288170809,
-0.888507248162344));
#71325=CARTESIAN_POINT('Ctrl Pts',(-0.16304937825703,0.172258914019895,
-0.888669333539511));
#71326=CARTESIAN_POINT('Ctrl Pts',(-0.159694356380409,0.175368165492342,
-0.888968016245174));
#71327=CARTESIAN_POINT('Ctrl Pts',(-0.158154985913881,0.176757689816749,
-0.889104228035403));
#71328=CARTESIAN_POINT('Ctrl Pts',(-0.155655164803658,0.178955371660737,
-0.889324228000585));
#71329=CARTESIAN_POINT('Ctrl Pts',(-0.154706152071789,0.179776421659302,
-0.889407476701386));
#71330=CARTESIAN_POINT('Ctrl Pts',(-0.152858375717605,0.181349582148963,
-0.889569074240294));
#71331=CARTESIAN_POINT('Ctrl Pts',(-0.151960463588417,0.18210263972164,
-0.889647380893023));
#71332=CARTESIAN_POINT('Ctrl Pts',(-0.149905857687856,0.183800011029056,
-0.889826087082309));
#71333=CARTESIAN_POINT('Ctrl Pts',(-0.148745762514662,0.18474010982933,
-0.889926653043626));
#71334=CARTESIAN_POINT('Ctrl Pts',(-0.145155401372374,0.187593864836568,
-0.890236917869707));
#71335=CARTESIAN_POINT('Ctrl Pts',(-0.142696596690058,0.189470917000551,
-0.890448050370114));
#71336=CARTESIAN_POINT('Ctrl Pts',(-0.122424523898745,0.204328175881824,
-0.892178777537975));
#71337=CARTESIAN_POINT('Ctrl Pts',(-0.102920510350732,0.214813236436444,
-0.893797282936546));
#71338=CARTESIAN_POINT('Ctrl Pts',(-0.0761309472811355,0.224719190371577,
-0.895874150753232));
#71339=CARTESIAN_POINT('Ctrl Pts',(-0.0699138555546477,0.226730456611347,
-0.89634557233232));
#71340=CARTESIAN_POINT('Ctrl Pts',(-0.0600961714632879,0.229464203586896,
-0.8970666250601));
#71341=CARTESIAN_POINT('Ctrl Pts',(-0.0565485654291269,0.23036413336333,
-0.897322508838198));
#71342=CARTESIAN_POINT('Ctrl Pts',(-0.0518954407814253,0.231430518562675,
-0.897650875322841));
#71343=CARTESIAN_POINT('Ctrl Pts',(-0.0508077912922736,0.231671729314368,
-0.897727116551379));
#71344=CARTESIAN_POINT('Ctrl Pts',(-0.0490295008634744,0.23205297917948,
-0.897850889022003));
#71345=CARTESIAN_POINT('Ctrl Pts',(-0.0483398795537936,0.232197616651937,
-0.897898672513225));
#71346=CARTESIAN_POINT('Ctrl Pts',(-0.0469912196344658,0.232474208495938,
-0.897991686176618));
#71347=CARTESIAN_POINT('Ctrl Pts',(-0.0463322502967748,0.232606437869259,
-0.898036930652904));
#71348=CARTESIAN_POINT('Ctrl Pts',(-0.0448549261492183,0.232896351987323,
-0.898137926342285));
#71349=CARTESIAN_POINT('Ctrl Pts',(-0.0440362759893075,0.233052529739542,
-0.898193593194436));
#71350=CARTESIAN_POINT('Ctrl Pts',(-0.0427911751582108,0.233283268442541,
-0.898277827287995));
#71351=CARTESIAN_POINT('Ctrl Pts',(-0.0423653301735287,0.233360979615656,
-0.898306560340943));
#71352=CARTESIAN_POINT('Ctrl Pts',(-0.0419392741323876,0.233437524640424,
-0.898335233456629));
#71353=CARTESIAN_POINT('',(-0.237175039616951,9.57688685589552E-5,-0.895455268706531));
#71354=CARTESIAN_POINT('Ctrl Pts',(-0.0419392742314872,0.23343752462262,
-0.917975447697368));
#71355=CARTESIAN_POINT('Ctrl Pts',(-0.0422317674705741,0.23338497542692,
-0.917954230877481));
#71356=CARTESIAN_POINT('Ctrl Pts',(-0.0425241685212188,0.233331875316163,
-0.917933000919219));
#71357=CARTESIAN_POINT('Ctrl Pts',(-0.0533943627192033,0.231336732356517,
-0.917143030107916));
#71358=CARTESIAN_POINT('Ctrl Pts',(-0.0638272696291555,0.228678138260806,
-0.916358145743216));
#71359=CARTESIAN_POINT('Ctrl Pts',(-0.0855467442851248,0.221540880198969,
-0.91468851198947));
#71360=CARTESIAN_POINT('Ctrl Pts',(-0.0967452791403489,0.216884800320748,
-0.913805944742864));
#71361=CARTESIAN_POINT('Ctrl Pts',(-0.10938401095843,0.210455217868708,
-0.912816840148667));
#71362=CARTESIAN_POINT('Ctrl Pts',(-0.111215657362555,0.20949305207031,
-0.912673703246731));
#71363=CARTESIAN_POINT('Ctrl Pts',(-0.113766474859567,0.208110218314762,
-0.912474897913189));
#71364=CARTESIAN_POINT('Ctrl Pts',(-0.114496314222815,0.207709575732239,
-0.912418077737528));
#71365=CARTESIAN_POINT('Ctrl Pts',(-0.115811156719384,0.206978761707875,
-0.912315846172132));
#71366=CARTESIAN_POINT('Ctrl Pts',(-0.116396894586063,0.206649932954719,
-0.912270351996501));
#71367=CARTESIAN_POINT('Ctrl Pts',(-0.117581841461388,0.205978076185156,
-0.912178426812099));
#71368=CARTESIAN_POINT('Ctrl Pts',(-0.118180961532467,0.205634913554832,
-0.912132004748522));
#71369=CARTESIAN_POINT('Ctrl Pts',(-0.119710439793986,0.204749970162841,
-0.912013616531119));
#71370=CARTESIAN_POINT('Ctrl Pts',(-0.120638635615156,0.204204454859977,
-0.911941885861967));
#71371=CARTESIAN_POINT('Ctrl Pts',(-0.122667272340464,0.202993533162125,
-0.911785294841027));
#71372=CARTESIAN_POINT('Ctrl Pts',(-0.12376608829564,0.202325455069047,
-0.911700595303086));
#71373=CARTESIAN_POINT('Ctrl Pts',(-0.126990354928992,0.200329009624858,
-0.911452243230933));
#71374=CARTESIAN_POINT('Ctrl Pts',(-0.129100309564777,0.198975811340943,
-0.911289958096488));
#71375=CARTESIAN_POINT('Ctrl Pts',(-0.136784929296316,0.193873645076855,
-0.910698238012091));
#71376=CARTESIAN_POINT('Ctrl Pts',(-0.142221386774673,0.189921556086763,
-0.910278270154202));
#71377=CARTESIAN_POINT('Ctrl Pts',(-0.159571933858356,0.176144982267166,
-0.908907836013511));
#71378=CARTESIAN_POINT('Ctrl Pts',(-0.170694589517402,0.165389283027187,
-0.907977124595711));
#71379=CARTESIAN_POINT('Ctrl Pts',(-0.185794422945062,0.147629369350368,
-0.906516310329683));
#71380=CARTESIAN_POINT('Ctrl Pts',(-0.190593045301499,0.141379876733652,
-0.906014762462898));
#71381=CARTESIAN_POINT('Ctrl Pts',(-0.196306168349518,0.133118667085378,
-0.905359382638094));
#71382=CARTESIAN_POINT('Ctrl Pts',(-0.19751608245608,0.131316746517983,
-0.905216887022205));
#71383=CARTESIAN_POINT('Ctrl Pts',(-0.199412528136862,0.128406861776938,
-0.904987355298596));
#71384=CARTESIAN_POINT('Ctrl Pts',(-0.200114970670058,0.127309374862874,
-0.904900915670784));
#71385=CARTESIAN_POINT('Ctrl Pts',(-0.201432334216918,0.125213300194608,
-0.904736041753284));
#71386=CARTESIAN_POINT('Ctrl Pts',(-0.202048963888699,0.124215827976891,
-0.90465767375895));
#71387=CARTESIAN_POINT('Ctrl Pts',(-0.203439091119634,0.121929391396564,
-0.90447822155915));
#71388=CARTESIAN_POINT('Ctrl Pts',(-0.20420777564749,0.120637574850504,
-0.904376965374131));
#71389=CARTESIAN_POINT('Ctrl Pts',(-0.20654799872374,0.116618239176673,
-0.904062273333156));
#71390=CARTESIAN_POINT('Ctrl Pts',(-0.208077500133248,0.113866771990018,
-0.903847343333906));
#71391=CARTESIAN_POINT('Ctrl Pts',(-0.215474078728602,0.0999139000285166,
-0.902759367325248));
#71392=CARTESIAN_POINT('Ctrl Pts',(-0.220492620940013,0.0882880516295587,
-0.901857447206898));
#71393=CARTESIAN_POINT('Ctrl Pts',(-0.229261579111557,0.0624864779643527,
-0.899878788967944));
#71394=CARTESIAN_POINT('Ctrl Pts',(-0.232674680326883,0.0482487333022393,
-0.898800453416702));
#71395=CARTESIAN_POINT('Ctrl Pts',(-0.235411728918039,0.0292315402947884,
-0.897431290780465));
#71396=CARTESIAN_POINT('Ctrl Pts',(-0.235934711108775,0.0246573299949662,
-0.897107475104667));
#71397=CARTESIAN_POINT('Ctrl Pts',(-0.23643022784052,0.0188227514627737,
-0.896703719396755));
#71398=CARTESIAN_POINT('Ctrl Pts',(-0.236526312246819,0.017574196914112,
-0.896617858352744));
#71399=CARTESIAN_POINT('Ctrl Pts',(-0.236663091987083,0.0155917170641874,
-0.896482443259699));
#71400=CARTESIAN_POINT('Ctrl Pts',(-0.236710270532387,0.0148582842783356,
-0.896432544350279));
#71401=CARTESIAN_POINT('Ctrl Pts',(-0.236791755443785,0.0134924516889735,
-0.896340005136011));
#71402=CARTESIAN_POINT('Ctrl Pts',(-0.236826938044166,0.0128601370356045,
-0.896297319035144));
#71403=CARTESIAN_POINT('Ctrl Pts',(-0.236893394091507,0.0115728309164111,
-0.896210721248901));
#71404=CARTESIAN_POINT('Ctrl Pts',(-0.236924484243125,0.0109178464712578,
-0.896166820274818));
#71405=CARTESIAN_POINT('Ctrl Pts',(-0.236990819385654,0.00938625604526191,
-0.896064520674928));
#71406=CARTESIAN_POINT('Ctrl Pts',(-0.237023918043973,0.00850955986828271,
-0.896006236543748));
#71407=CARTESIAN_POINT('Ctrl Pts',(-0.237133017466511,0.00512120341351875,
-0.89578195832203));
#71408=CARTESIAN_POINT('Ctrl Pts',(-0.237173968865591,0.00260849225459629,
-0.895617730207301));
#71409=CARTESIAN_POINT('Ctrl Pts',(-0.237174980771817,9.55033420706099E-5,
-0.895455149390825));
#71410=CARTESIAN_POINT('Ctrl Pts',(-0.237174980662101,9.5775424050204E-5,
-0.8954551669935));
#71411=CARTESIAN_POINT('Ctrl Pts',(-0.2371833279887,-0.0205752583428094,
-0.89411782880804));
#71412=CARTESIAN_POINT('Ctrl Pts',(-0.234489360101835,-0.041162614077105,
-0.892892067334419));
#71413=CARTESIAN_POINT('Ctrl Pts',(-0.226502289821164,-0.0710973627577832,
-0.890969390586061));
#71414=CARTESIAN_POINT('Ctrl Pts',(-0.223200885745565,-0.0808668486431776,
-0.890319190464305));
#71415=CARTESIAN_POINT('Ctrl Pts',(-0.218416242996458,-0.0924738090747347,
-0.889500763002097));
#71416=CARTESIAN_POINT('Ctrl Pts',(-0.217527632660627,-0.0945451692293766,
-0.889352888167248));
#71417=CARTESIAN_POINT('Ctrl Pts',(-0.21607154873807,-0.0978100806068398,
-0.889116746347139));
#71418=CARTESIAN_POINT('Ctrl Pts',(-0.215523372865828,-0.0990121289090137,
-0.889029139052045));
#71419=CARTESIAN_POINT('Ctrl Pts',(-0.214471084072819,-0.101269454115096,
-0.888863328947414));
#71420=CARTESIAN_POINT('Ctrl Pts',(-0.213969151054201,-0.102325708171585,
-0.888785203332076));
#71421=CARTESIAN_POINT('Ctrl Pts',(-0.212817548923232,-0.104703582438074,
-0.888608079379626));
#71422=CARTESIAN_POINT('Ctrl Pts',(-0.212163345773567,-0.106022940182293,
-0.888508925476395));
#71423=CARTESIAN_POINT('Ctrl Pts',(-0.210144695538564,-0.110000523779266,
-0.88820727898241));
#71424=CARTESIAN_POINT('Ctrl Pts',(-0.208742308037355,-0.11263905054928,
-0.888003465609751));
#71425=CARTESIAN_POINT('Ctrl Pts',(-0.19796257661731,-0.132027601974797,
-0.886477268126378));
#71426=CARTESIAN_POINT('Ctrl Pts',(-0.186633985986837,-0.147607381284134,
-0.885081975229611));
#71427=CARTESIAN_POINT('Ctrl Pts',(-0.171297000813657,-0.164074074110974,
-0.883438992480977));
#71428=CARTESIAN_POINT('Ctrl Pts',(-0.168987590417036,-0.166451672001164,
-0.883197267798034));
#71429=CARTESIAN_POINT('Ctrl Pts',(-0.162136577340472,-0.173215371798461,
-0.882497743174002));
#71430=CARTESIAN_POINT('Ctrl Pts',(-0.157468459187152,-0.177469799783668,
-0.882042539813931));
#71431=CARTESIAN_POINT('Ctrl Pts',(-0.15079225631944,-0.183083253596495,
-0.881425790475272));
#71432=CARTESIAN_POINT('Ctrl Pts',(-0.148925079541231,-0.184605265342825,
-0.88125679631911));
#71433=CARTESIAN_POINT('Ctrl Pts',(-0.146053459246999,-0.186874108374204,
-0.881002533941513));
#71434=CARTESIAN_POINT('Ctrl Pts',(-0.145065810896337,-0.187641829050827,
-0.880916073844857));
#71435=CARTESIAN_POINT('Ctrl Pts',(-0.143253360462092,-0.189027822546557,
-0.880759272098043));
#71436=CARTESIAN_POINT('Ctrl Pts',(-0.142430519645353,-0.189648596493712,
-0.880688774197995));
#71437=CARTESIAN_POINT('Ctrl Pts',(-0.141052432602468,-0.190674235289257,
-0.880571883656095));
#71438=CARTESIAN_POINT('Ctrl Pts',(-0.140499436805848,-0.191082079311968,
-0.880525290836942));
#71439=CARTESIAN_POINT('Ctrl Pts',(-0.139402358511907,-0.191883856139328,
-0.880433485513471));
#71440=CARTESIAN_POINT('Ctrl Pts',(-0.138858363857907,-0.192277889028762,
-0.880388267233697));
#71441=CARTESIAN_POINT('Ctrl Pts',(-0.137636427864242,-0.193155086334715,
-0.880287357921831));
#71442=CARTESIAN_POINT('Ctrl Pts',(-0.136957594889835,-0.193637008100672,
-0.880231750910971));
#71443=CARTESIAN_POINT('Ctrl Pts',(-0.134583351586567,-0.195303815536937,
-0.880038778703969));
#71444=CARTESIAN_POINT('Ctrl Pts',(-0.132874932123937,-0.196470130081977,
-0.879902597292944));
#71445=CARTESIAN_POINT('Ctrl Pts',(-0.120926123331054,-0.204400251875899,
-0.878966866343392));
#71446=CARTESIAN_POINT('Ctrl Pts',(-0.110188147934243,-0.210383555639259,
-0.878209602267129));
#71447=CARTESIAN_POINT('Ctrl Pts',(-0.0889697948786052,-0.220134127059846,
-0.876776498883495));
#71448=CARTESIAN_POINT('Ctrl Pts',(-0.0785941490472483,-0.224048224029627,
-0.876101581428695));
#71449=CARTESIAN_POINT('Ctrl Pts',(-0.0595644883586007,-0.2297417577492,
-0.874861369663294));
#71450=CARTESIAN_POINT('Ctrl Pts',(-0.0510129591517752,-0.231790541007762,
-0.87430336439305));
#71451=CARTESIAN_POINT('Ctrl Pts',(-0.040240880356109,-0.233746286773871,
-0.873588939578593));
#71452=CARTESIAN_POINT('Ctrl Pts',(-0.0381084973051501,-0.234103389461559,
-0.873446983013624));
#71453=CARTESIAN_POINT('Ctrl Pts',(-0.0346854202018894,-0.234628632998662,
-0.873218113645547));
#71454=CARTESIAN_POINT('Ctrl Pts',(-0.0333976735292816,-0.234815393630019,
-0.873131791133101));
#71455=CARTESIAN_POINT('Ctrl Pts',(-0.0309462015268082,-0.235150354752359,
-0.872967006604323));
#71456=CARTESIAN_POINT('Ctrl Pts',(-0.0297827825134924,-0.235300536568753,
-0.872888609765996));
#71457=CARTESIAN_POINT('Ctrl Pts',(-0.0271227830617879,-0.23562386323407,
-0.872708901944158));
#71458=CARTESIAN_POINT('Ctrl Pts',(-0.0256255838670595,-0.235791389909411,
-0.87260741719276));
#71459=CARTESIAN_POINT('Ctrl Pts',(-0.0209778235715432,-0.236266654534565,
-0.872291286249288));
#71460=CARTESIAN_POINT('Ctrl Pts',(-0.0178227363863988,-0.236525578968084,
-0.872075126129018));
#71461=CARTESIAN_POINT('Ctrl Pts',(0.0021219000778639,-0.237761036115639,
-0.870698229641039));
#71462=CARTESIAN_POINT('Ctrl Pts',(0.0189673367611407,-0.237012354393224,
-0.869483519007522));
#71463=CARTESIAN_POINT('Ctrl Pts',(0.0495866263073657,-0.232365231578005,
-0.867222016049639));
#71464=CARTESIAN_POINT('Ctrl Pts',(0.0633675483631206,-0.228991414833525,
-0.866184927746579));
#71465=CARTESIAN_POINT('Ctrl Pts',(0.0784383708613653,-0.223835934910005,
-0.865078497175109));
#71466=CARTESIAN_POINT('Ctrl Pts',(0.0801041033765616,-0.223245239295858,
-0.864956629477448));
#71467=CARTESIAN_POINT('Ctrl Pts',(0.0825531662542952,-0.222345820042513,
-0.864778236736914));
#71468=CARTESIAN_POINT('Ctrl Pts',(0.0833416595325406,-0.222051473290209,
-0.864720922990878));
#71469=CARTESIAN_POINT('Ctrl Pts',(0.0847419942105739,-0.221520214585848,
-0.86461937278853));
#71470=CARTESIAN_POINT('Ctrl Pts',(0.0853544366467714,-0.22128495482819,
-0.864575041685921));
#71471=CARTESIAN_POINT('Ctrl Pts',(0.0866908465595962,-0.220765220878756,
-0.864478489163186));
#71472=CARTESIAN_POINT('Ctrl Pts',(0.0874143955017434,-0.22047972498516,
-0.864426329192201));
#71473=CARTESIAN_POINT('Ctrl Pts',(0.0894455470287741,-0.219666708394509,
-0.864280193266529));
#71474=CARTESIAN_POINT('Ctrl Pts',(0.0907498953274171,-0.219131068992247,
-0.864186685863723));
#71475=CARTESIAN_POINT('Ctrl Pts',(0.0987440397171926,-0.215764596382242,
-0.863615211447208));
#71476=CARTESIAN_POINT('Ctrl Pts',(0.105306345368305,-0.212638996443293,
-0.86315305719111));
#71477=CARTESIAN_POINT('Ctrl Pts',(0.125148109955444,-0.202044089890315,
-0.861746542527685));
#71478=CARTESIAN_POINT('Ctrl Pts',(0.137859132259978,-0.193594320187097,
-0.860830153603925));
#71479=CARTESIAN_POINT('Ctrl Pts',(0.157835757106226,-0.177343140849288,
-0.859233297960712));
#71480=CARTESIAN_POINT('Ctrl Pts',(0.165546872520648,-0.170167291408317,
-0.858569765083902));
#71481=CARTESIAN_POINT('Ctrl Pts',(0.174307683228324,-0.160853796874688,
-0.857736316400822));
#71482=CARTESIAN_POINT('Ctrl Pts',(0.175836049154033,-0.1591816435297,-0.857587702763485));
#71483=CARTESIAN_POINT('Ctrl Pts',(0.178219093141709,-0.156498202685523,
-0.857350653165804));
#71484=CARTESIAN_POINT('Ctrl Pts',(0.179089683945134,-0.155501181950484,
-0.857262885786001));
#71485=CARTESIAN_POINT('Ctrl Pts',(0.180713421334071,-0.153609917489975,
-0.857096941533867));
#71486=CARTESIAN_POINT('Ctrl Pts',(0.181468392684931,-0.152717287081412,
-0.857018843319827));
#71487=CARTESIAN_POINT('Ctrl Pts',(0.183156911309922,-0.150690689120273,
-0.856842010223158));
#71488=CARTESIAN_POINT('Ctrl Pts',(0.18408657883312,-0.149553566566187,
-0.856743121844801));
#71489=CARTESIAN_POINT('Ctrl Pts',(0.186802034108475,-0.146168474290219,
-0.856449668282114));
#71490=CARTESIAN_POINT('Ctrl Pts',(0.188557579829598,-0.143896701320385,
-0.856253914229598));
#71491=CARTESIAN_POINT('Ctrl Pts',(0.20213780965615,-0.125647802440641,
-0.854690062659708));
#71492=CARTESIAN_POINT('Ctrl Pts',(0.211950444148434,-0.108276300980372,
-0.853242877107898));
#71493=CARTESIAN_POINT('Ctrl Pts',(0.222615336530566,-0.0822362210983325,
-0.851189165810966));
#71494=CARTESIAN_POINT('Ctrl Pts',(0.225347647827582,-0.0744233774972007,
-0.850587838837127));
#71495=CARTESIAN_POINT('Ctrl Pts',(0.228857953258422,-0.0624026419056772,
-0.849697986252965));
#71496=CARTESIAN_POINT('Ctrl Pts',(0.229939759067294,-0.0582903524159181,
-0.84939968204986));
#71497=CARTESIAN_POINT('Ctrl Pts',(0.231178202201684,-0.0530093784162907,
-0.849026176563722));
#71498=CARTESIAN_POINT('Ctrl Pts',(0.23143744068887,-0.0518658516146378,
-0.848945866513497));
#71499=CARTESIAN_POINT('Ctrl Pts',(0.231841600007677,-0.0500196732296625,
-0.848817173739897));
#71500=CARTESIAN_POINT('Ctrl Pts',(0.231991827861597,-0.0493182222347262,
-0.848768500860114));
#71501=CARTESIAN_POINT('Ctrl Pts',(0.232275057373258,-0.0479658185022591,
-0.848675103592373));
#71502=CARTESIAN_POINT('Ctrl Pts',(0.232408508817347,-0.0473149771561448,
-0.848630355573465));
#71503=CARTESIAN_POINT('Ctrl Pts',(0.232697317105471,-0.045875754963413,
-0.848531827302156));
#71504=CARTESIAN_POINT('Ctrl Pts',(0.232851407355918,-0.0450871203437479,
-0.848478118062628));
#71505=CARTESIAN_POINT('Ctrl Pts',(0.233382838095572,-0.0422918478131074,
-0.848288690510409));
#71506=CARTESIAN_POINT('Ctrl Pts',(0.233738284786237,-0.0402810678347254,
-0.848154141446342));
#71507=CARTESIAN_POINT('Ctrl Pts',(0.236453887863799,-0.0236700479544012,
-0.847054862999609));
#71508=CARTESIAN_POINT('Ctrl Pts',(0.237469927377849,-0.00888087333447466,
-0.846152508716175));
#71509=CARTESIAN_POINT('Ctrl Pts',(0.236815643676436,0.0173756426311385,
-0.844542863002117));
#71510=CARTESIAN_POINT('Ctrl Pts',(0.235698359733893,0.0288065878120799,
-0.843839540075188));
#71511=CARTESIAN_POINT('Ctrl Pts',(0.233039238763601,0.0443033384358003,
-0.842845799544846));
#71512=CARTESIAN_POINT('Ctrl Pts',(0.232207282796865,0.0484752224073258,
-0.842574303528889));
#71513=CARTESIAN_POINT('Ctrl Pts',(0.230555508365567,0.0557344136510711,
-0.842093256594152));
#71514=CARTESIAN_POINT('Ctrl Pts',(0.229784653622529,0.0588317829199541,
-0.84188521201821));
#71515=CARTESIAN_POINT('Ctrl Pts',(0.228557015864354,0.0633715674101596,
-0.841575700214298));
#71516=CARTESIAN_POINT('Ctrl Pts',(0.228148538908001,0.064826762013574,
-0.841475788334233));
#71517=CARTESIAN_POINT('Ctrl Pts',(0.227398212510716,0.0674048296048628,
-0.8412974877106));
#71518=CARTESIAN_POINT('Ctrl Pts',(0.227061880769916,0.0685292661815689,
-0.841219280777512));
#71519=CARTESIAN_POINT('Ctrl Pts',(0.226335864440256,0.0708924780171649,
-0.84105396276005));
#71520=CARTESIAN_POINT('Ctrl Pts',(0.225944324798897,0.0721306380538118,
-0.840966793114157));
#71521=CARTESIAN_POINT('Ctrl Pts',(0.224877595502658,0.0754100125288046,
-0.840734408415306));
#71522=CARTESIAN_POINT('Ctrl Pts',(0.224184798069977,0.0774453273721836,
-0.840588618926588));
#71523=CARTESIAN_POINT('Ctrl Pts',(0.220944960016308,0.0865554387302815,
-0.839928819321502));
#71524=CARTESIAN_POINT('Ctrl Pts',(0.21809026665488,0.0935154180634417,
-0.839404751213831));
#71525=CARTESIAN_POINT('Ctrl Pts',(0.208295972394384,0.114495646493638,
-0.837761968967058));
#71526=CARTESIAN_POINT('Ctrl Pts',(0.200297381014247,0.127973940981892,
-0.836613311660793));
#71527=CARTESIAN_POINT('Ctrl Pts',(0.186969679747982,0.146086642333035,
-0.834976586780541));
#71528=CARTESIAN_POINT('Ctrl Pts',(0.182669372368285,0.151429459658708,
-0.83448106533778));
#71529=CARTESIAN_POINT('Ctrl Pts',(0.17565028083982,0.159415245438648,-0.833728148827456));
#71530=CARTESIAN_POINT('Ctrl Pts',(0.173089616222914,0.162191955302024,
-0.833463886762648));
#71531=CARTESIAN_POINT('Ctrl Pts',(0.169680542239703,0.165715908868075,
-0.833126549843501));
#71532=CARTESIAN_POINT('Ctrl Pts',(0.1688917528536,0.166519743009972,-0.833049464633647));
#71533=CARTESIAN_POINT('Ctrl Pts',(0.167598402441187,0.167819117331175,
-0.832924680193496));
#71534=CARTESIAN_POINT('Ctrl Pts',(0.167097309497062,0.168318061523262,
-0.832876720949228));
#71535=CARTESIAN_POINT('Ctrl Pts',(0.166117052787265,0.169285422822658,
-0.832783665329727));
#71536=CARTESIAN_POINT('Ctrl Pts',(0.165638125573272,0.16975406027289,-0.832738552611137));
#71537=CARTESIAN_POINT('Ctrl Pts',(0.164564218738812,0.170796022240532,
-0.832638160610473));
#71538=CARTESIAN_POINT('Ctrl Pts',(0.163968210096285,0.17136828595456,-0.832582962528883));
#71539=CARTESIAN_POINT('Ctrl Pts',(0.161896021252461,0.173337210642539,
-0.832392783827761));
#71540=CARTESIAN_POINT('Ctrl Pts',(0.160404840309692,0.174718053373907,
-0.832258942536074));
#71541=CARTESIAN_POINT('Ctrl Pts',(0.148502535299551,0.185458814417964,
-0.831212371159709));
#71542=CARTESIAN_POINT('Ctrl Pts',(0.137297497147454,0.193900696884352,
-0.830355239188223));
#71543=CARTESIAN_POINT('Ctrl Pts',(0.11200086852914,0.209660297054008,-0.828528525171795));
#71544=CARTESIAN_POINT('Ctrl Pts',(0.0977902934622816,0.216653231324984,
-0.827561605299581));
#71545=CARTESIAN_POINT('Ctrl Pts',(0.0795799210739103,0.223455306973142,
-0.826310146657614));
#71546=CARTESIAN_POINT('Ctrl Pts',(0.076140300878525,0.224650596085608,
-0.826073434051857));
#71547=CARTESIAN_POINT('Ctrl Pts',(0.0711594475923189,0.226253944631179,
-0.825729499993171));
#71548=CARTESIAN_POINT('Ctrl Pts',(0.0696393805797029,0.226726423048257,
-0.825624386809163));
#71549=CARTESIAN_POINT('Ctrl Pts',(0.0669795384547398,0.227523903116119,
-0.825440141227738));
#71550=CARTESIAN_POINT('Ctrl Pts',(0.0658418566889726,0.227855732605556,
-0.825361234559976));
#71551=CARTESIAN_POINT('Ctrl Pts',(0.0634870072887151,0.228523466593681,
-0.825197678987938));
#71552=CARTESIAN_POINT('Ctrl Pts',(0.0622695509014142,0.2288582045767,-0.825112995027067));
#71553=CARTESIAN_POINT('Ctrl Pts',(0.0591322035722137,0.229693926764797,
-0.824894414979077));
#71554=CARTESIAN_POINT('Ctrl Pts',(0.0572086265134711,0.230180559836876,
-0.824760060662697));
#71555=CARTESIAN_POINT('Ctrl Pts',(0.0494064273457805,0.23205054724841,
-0.824213606799371));
#71556=CARTESIAN_POINT('Ctrl Pts',(0.0434825218316268,0.23323316758651,
-0.823795197737063));
#71557=CARTESIAN_POINT('Ctrl Pts',(0.0208489583708216,0.236859393391516,
-0.822182413451291));
#71558=CARTESIAN_POINT('Ctrl Pts',(0.00394170992783503,0.23774223495821,
-0.82094419783548));
#71559=CARTESIAN_POINT('Ctrl Pts',(-0.0226485214267444,0.236292375576695,
-0.819004074324007));
#71560=CARTESIAN_POINT('Ctrl Pts',(-0.0323423762680234,0.235161698747638,
-0.818299570554947));
#71561=CARTESIAN_POINT('Ctrl Pts',(-0.0419392746656718,0.233437524544614,
-0.817620397237267));
#71562=CARTESIAN_POINT('Origin',(0.,0.,-2.1456589891905));
#71563=CARTESIAN_POINT('',(-0.0419392741328079,0.233437524640348,-0.698115075114807));
#71564=CARTESIAN_POINT('',(-0.0419393227885566,0.233437515898874,-0.717844391575082));
#71565=CARTESIAN_POINT('',(-0.0419392741328076,0.233437524640348,-2.1456589891905));
#71566=CARTESIAN_POINT('',(-0.237174928456985,-0.000184218414099613,-0.775941010809497));
#71567=CARTESIAN_POINT('Ctrl Pts',(-0.237174928456985,-0.000184218414099613,
-0.775941010809497));
#71568=CARTESIAN_POINT('Ctrl Pts',(-0.237162061016635,-0.0167506092354838,
-0.774832628374937));
#71569=CARTESIAN_POINT('Ctrl Pts',(-0.235409393017015,-0.0332436070647559,
-0.773724245940377));
#71570=CARTESIAN_POINT('Ctrl Pts',(-0.23198655433952,-0.0493378073152505,
-0.772615863505817));
#71571=CARTESIAN_POINT('Ctrl Pts',(-0.229974034838635,-0.0588006815278866,
-0.771964170138362));
#71572=CARTESIAN_POINT('Ctrl Pts',(-0.227385071187055,-0.0681260551951133,
-0.771312476770907));
#71573=CARTESIAN_POINT('Ctrl Pts',(-0.224241480738865,-0.077251142004771,
-0.770660783403453));
#71574=CARTESIAN_POINT('Ctrl Pts',(-0.219669392181079,-0.0905228151692113,
-0.76971295007795));
#71575=CARTESIAN_POINT('Ctrl Pts',(-0.213899560933309,-0.103431980680553,
-0.768765116752448));
#71576=CARTESIAN_POINT('Ctrl Pts',(-0.207011145932222,-0.115751311374119,
-0.767817283426946));
#71577=CARTESIAN_POINT('Ctrl Pts',(-0.200136684144792,-0.128045687959483,
-0.766871370038164));
#71578=CARTESIAN_POINT('Ctrl Pts',(-0.192148477163569,-0.139751845841727,
-0.765925456649382));
#71579=CARTESIAN_POINT('Ctrl Pts',(-0.183172969367591,-0.150664010029136,
-0.764979543260599));
#71580=CARTESIAN_POINT('Ctrl Pts',(-0.174198898800311,-0.161574426875236,
-0.764033781338887));
#71581=CARTESIAN_POINT('Ctrl Pts',(-0.164238331879677,-0.171690427447469,
-0.763088019417175));
#71582=CARTESIAN_POINT('Ctrl Pts',(-0.153459453442516,-0.180837431894296,
-0.762142257495463));
#71583=CARTESIAN_POINT('Ctrl Pts',(-0.142682378474369,-0.189982905909254,
-0.761196653813992));
#71584=CARTESIAN_POINT('Ctrl Pts',(-0.131087912400795,-0.198159179364291,
-0.76025105013252));
#71585=CARTESIAN_POINT('Ctrl Pts',(-0.118877396065784,-0.20523193058006,
-0.759305446451049));
#71586=CARTESIAN_POINT('Ctrl Pts',(-0.10663829229987,-0.212321240619481,
-0.758357628909069));
#71587=CARTESIAN_POINT('Ctrl Pts',(-0.0937810050099268,-0.21830148975904,
-0.757409811367089));
#71588=CARTESIAN_POINT('Ctrl Pts',(-0.0805311358005377,-0.223084550768706,
-0.756461993825109));
#71589=CARTESIAN_POINT('Ctrl Pts',(-0.0726787485432168,-0.225919178547271,
-0.755900280326561));
#71590=CARTESIAN_POINT('Ctrl Pts',(-0.0646888594965764,-0.228334261078944,
-0.755338566828013));
#71591=CARTESIAN_POINT('Ctrl Pts',(-0.0566104850057974,-0.230319850669473,
-0.754776853329465));
#71592=CARTESIAN_POINT('Ctrl Pts',(-0.0429790651128494,-0.23367032736184,
-0.753829020003963));
#71593=CARTESIAN_POINT('Ctrl Pts',(-0.029003155145229,-0.235817755452354,
-0.752881186678461));
#71594=CARTESIAN_POINT('Ctrl Pts',(-0.0149167021231715,-0.236705455414041,
-0.751933353352959));
#71595=CARTESIAN_POINT('Ctrl Pts',(-0.000858782702629119,-0.237591357245501,
-0.750987439964177));
#71596=CARTESIAN_POINT('Ctrl Pts',(0.0133084155970279,-0.237222473148615,
-0.750041526575395));
#71597=CARTESIAN_POINT('Ctrl Pts',(0.0273434308589045,-0.235593542810206,
-0.749095613186613));
#71598=CARTESIAN_POINT('Ctrl Pts',(0.0413761987240736,-0.233964873308897,
-0.748149851264901));
#71599=CARTESIAN_POINT('Ctrl Pts',(0.0552759924229695,-0.231076604608448,
-0.747204089343188));
#71600=CARTESIAN_POINT('Ctrl Pts',(0.0688049442860343,-0.226975461816461,
-0.746258327421476));
#71601=CARTESIAN_POINT('Ctrl Pts',(0.0823316325513042,-0.222875005207548,
-0.745312723740004));
#71602=CARTESIAN_POINT('Ctrl Pts',(0.0954868083391503,-0.217562337221152,
-0.744367120058533));
#71603=CARTESIAN_POINT('Ctrl Pts',(0.108048467294751,-0.211133865924572,
-0.743421516377061));
#71604=CARTESIAN_POINT('Ctrl Pts',(0.120639535781249,-0.204690344201461,
-0.742473698835081));
#71605=CARTESIAN_POINT('Ctrl Pts',(0.132633588921921,-0.197126224590689,
-0.741525881293101));
#71606=CARTESIAN_POINT('Ctrl Pts',(0.14383429546831,-0.188583339858363,
-0.740578063751121));
#71607=CARTESIAN_POINT('Ctrl Pts',(0.150472269320576,-0.183520494470776,
-0.740016350252573));
#71608=CARTESIAN_POINT('Ctrl Pts',(0.156832180133812,-0.178114711913168,
-0.739454636754024));
#71609=CARTESIAN_POINT('Ctrl Pts',(0.162879102495285,-0.172401794060649,
-0.738892923255476));
#71610=CARTESIAN_POINT('Ctrl Pts',(0.173082657413835,-0.162761837142276,
-0.737945089929974));
#71611=CARTESIAN_POINT('Ctrl Pts',(0.182461876269478,-0.152180355181562,
-0.736997256604472));
#71612=CARTESIAN_POINT('Ctrl Pts',(0.190842333428052,-0.140823238127577,
-0.73604942327897));
#71613=CARTESIAN_POINT('Ctrl Pts',(0.199205815083659,-0.129489126116228,
-0.735103509890188));
#71614=CARTESIAN_POINT('Ctrl Pts',(0.206574003311319,-0.11738311994654,
-0.734157596501406));
#71615=CARTESIAN_POINT('Ctrl Pts',(0.212811612220942,-0.104705292745512,
-0.733211683112624));
#71616=CARTESIAN_POINT('Ctrl Pts',(0.21904822231571,-0.0920294956175973,
-0.732265921190912));
#71617=CARTESIAN_POINT('Ctrl Pts',(0.224154200017897,-0.0787827846045709,
-0.731320159269199));
#71618=CARTESIAN_POINT('Ctrl Pts',(0.228039895844241,-0.0651903867786343,
-0.730374397347487));
#71619=CARTESIAN_POINT('Ctrl Pts',(0.231924941535039,-0.0516002631659596,
-0.729428793666016));
#71620=CARTESIAN_POINT('Ctrl Pts',(0.234589898825739,-0.0376653755172719,
-0.728483189984544));
#71621=CARTESIAN_POINT('Ctrl Pts',(0.235995469124175,-0.0236245460879286,
-0.727537586303073));
#71622=CARTESIAN_POINT('Ctrl Pts',(0.237404330163369,-0.00955084407317458,
-0.726589768761093));
#71623=CARTESIAN_POINT('Ctrl Pts',(0.237547878768334,0.00462845809672525,
-0.725641951219113));
#71624=CARTESIAN_POINT('Ctrl Pts',(0.236438905218546,0.01867149496038,-0.724694133677133));
#71625=CARTESIAN_POINT('Ctrl Pts',(0.235781684408782,0.0269939441845676,
-0.724132420178585));
#71626=CARTESIAN_POINT('Ctrl Pts',(0.234685558114345,0.0352685715332205,
-0.723570706680036));
#71627=CARTESIAN_POINT('Ctrl Pts',(0.233161685622907,0.0434466222218101,
-0.723008993181488));
#71628=CARTESIAN_POINT('Ctrl Pts',(0.230590308693327,0.0572462353703723,
-0.722061159855986));
#71629=CARTESIAN_POINT('Ctrl Pts',(0.226780910724152,0.0708633567232648,
-0.721113326530485));
#71630=CARTESIAN_POINT('Ctrl Pts',(0.221778371785606,0.0840614919753727,
-0.720165493204983));
#71631=CARTESIAN_POINT('Ctrl Pts',(0.216785966019151,0.0972328930076286,
-0.719219579816201));
#71632=CARTESIAN_POINT('Ctrl Pts',(0.210605442854837,0.10998619518997,-0.718273666427419));
#71633=CARTESIAN_POINT('Ctrl Pts',(0.203331622400047,0.122099270911684,
-0.717327753038637));
#71634=CARTESIAN_POINT('Ctrl Pts',(0.19605896668643,0.13421040699272,-0.716381991116925));
#71635=CARTESIAN_POINT('Ctrl Pts',(0.187693747281197,0.145680780363284,
-0.715436229195212));
#71636=CARTESIAN_POINT('Ctrl Pts',(0.178376657178569,0.156312983462025,
-0.7144904672735));
#71637=CARTESIAN_POINT('Ctrl Pts',(0.169061125965707,0.166943407632751,
-0.713544863592029));
#71638=CARTESIAN_POINT('Ctrl Pts',(0.158794604413171,0.176735324010771,
-0.712599259910558));
#71639=CARTESIAN_POINT('Ctrl Pts',(0.147756499553455,0.185526271629411,
-0.711653656229086));
#71640=CARTESIAN_POINT('Ctrl Pts',(0.13669255212891,0.194337800737049,-0.710705838687106));
#71641=CARTESIAN_POINT('Ctrl Pts',(0.124854097086247,0.20214319620622,-0.709758021145126));
#71642=CARTESIAN_POINT('Ctrl Pts',(0.11245132957152,0.208822123115817,-0.708810203603146));
#71643=CARTESIAN_POINT('Ctrl Pts',(0.105100967688763,0.212780314681992,
-0.708248490104597));
#71644=CARTESIAN_POINT('Ctrl Pts',(0.0975529215632221,0.21634373302667,
-0.707686776606049));
#71645=CARTESIAN_POINT('Ctrl Pts',(0.0898542126077082,0.219495332755958,
-0.707125063107501));
#71646=CARTESIAN_POINT('Ctrl Pts',(0.0768636571902303,0.224813241404485,
-0.706177245704115));
#71647=CARTESIAN_POINT('Ctrl Pts',(0.0633555145593011,0.228991853235572,
-0.705229428300729));
#71648=CARTESIAN_POINT('Ctrl Pts',(0.0495528462405892,0.231940716680915,
-0.704281610897343));
#71649=CARTESIAN_POINT('Ctrl Pts',(0.0357780041000708,0.234883635217795,
-0.703335704293765));
#71650=CARTESIAN_POINT('Ctrl Pts',(0.0217106075155237,0.236601484212659,
-0.702389797690186));
#71651=CARTESIAN_POINT('Ctrl Pts',(0.00758871636857107,0.237053563586117,
-0.701443891086607));
#71652=CARTESIAN_POINT('Ctrl Pts',(-0.0065210615412059,0.237505255182569,
-0.700498795846812));
#71653=CARTESIAN_POINT('Ctrl Pts',(-0.0206844113366518,0.236693274397738,
-0.699553700607018));
#71654=CARTESIAN_POINT('Ctrl Pts',(-0.0346596912665034,0.234628826929494,
-0.698608605367223));
#71655=CARTESIAN_POINT('Ctrl Pts',(-0.0370923291428906,0.234269474334751,
-0.698444095283084));
#71656=CARTESIAN_POINT('Ctrl Pts',(-0.039519276226885,0.233872300307772,
-0.698279585198946));
#71657=CARTESIAN_POINT('Ctrl Pts',(-0.0419392741328079,0.233437524640348,
-0.698115075114807));
#71658=CARTESIAN_POINT('Ctrl Pts',(-0.0419215622832843,0.23334603455685,
-0.798097588861632));
#71659=CARTESIAN_POINT('Ctrl Pts',(-0.0983464490172812,0.2226473034456,
-0.794246630400235));
#71660=CARTESIAN_POINT('Ctrl Pts',(-0.200199235814832,0.163360521026062,
-0.786861104382857));
#71661=CARTESIAN_POINT('Ctrl Pts',(-0.236573687440461,0.0525967050833675,
-0.779475578365479));
#71662=CARTESIAN_POINT('Ctrl Pts',(-0.236955669095664,-0.000184048111057593,
-0.775941010809497));
#71663=CARTESIAN_POINT('Ctrl Pts',(-0.0419392746656718,0.233437524544614,
-0.817620397237267));
#71664=CARTESIAN_POINT('Ctrl Pts',(-0.0427439480341241,0.233292957309841,
-0.817563450434388));
#71665=CARTESIAN_POINT('Ctrl Pts',(-0.0435479399485291,0.233144217572963,
-0.817506684327751));
#71666=CARTESIAN_POINT('Ctrl Pts',(-0.0457952628982983,0.232716426896028,
-0.817348411761257));
#71667=CARTESIAN_POINT('Ctrl Pts',(-0.0472367674736412,0.232428116896829,
-0.81724735352858));
#71668=CARTESIAN_POINT('Ctrl Pts',(-0.0494407928101261,0.231965945750991,
-0.817093643268754));
#71669=CARTESIAN_POINT('Ctrl Pts',(-0.0502052580879215,0.231801691293878,
-0.817040477952749));
#71670=CARTESIAN_POINT('Ctrl Pts',(-0.0516093200306797,0.231492740042138,
-0.816943123131538));
#71671=CARTESIAN_POINT('Ctrl Pts',(-0.0522491310536985,0.231349171016976,
-0.816898873505168));
#71672=CARTESIAN_POINT('Ctrl Pts',(-0.0537036484141713,0.231016445826355,
-0.816798531125211));
#71673=CARTESIAN_POINT('Ctrl Pts',(-0.0545179561465916,0.23082563247276,
-0.816742533375943));
#71674=CARTESIAN_POINT('Ctrl Pts',(-0.0566436695176156,0.230315646246639,
-0.81659678032813));
#71675=CARTESIAN_POINT('Ctrl Pts',(-0.0579534118856586,0.229989574678711,
-0.816507401155402));
#71676=CARTESIAN_POINT('Ctrl Pts',(-0.0689112921291509,0.227161962753133,
-0.81576263758787));
#71677=CARTESIAN_POINT('Ctrl Pts',(-0.0783969782197981,0.224065367249695,
-0.815137441683313));
#71678=CARTESIAN_POINT('Ctrl Pts',(-0.101823092521564,0.214747169635626,
-0.813578980107706));
#71679=CARTESIAN_POINT('Ctrl Pts',(-0.115409133106069,0.207761930697755,
-0.812659435693295));
#71680=CARTESIAN_POINT('Ctrl Pts',(-0.134955309620725,0.19519973824423,
-0.811203347655245));
#71681=CARTESIAN_POINT('Ctrl Pts',(-0.141456188803627,0.190541332177932,
-0.810694120162893));
#71682=CARTESIAN_POINT('Ctrl Pts',(-0.149354899955749,0.184253953979465,
-0.810034902534873));
#71683=CARTESIAN_POINT('Ctrl Pts',(-0.150983182973067,0.182922069986648,
-0.80989671526072));
#71684=CARTESIAN_POINT('Ctrl Pts',(-0.153579910783673,0.180739735242425,
-0.809672476306788));
#71685=CARTESIAN_POINT('Ctrl Pts',(-0.154559540091236,0.179902721900582,
-0.809586972385282));
#71686=CARTESIAN_POINT('Ctrl Pts',(-0.156420261271962,0.178286471474932,
-0.809422786141139));
#71687=CARTESIAN_POINT('Ctrl Pts',(-0.157302474240647,0.177508578832443,
-0.809344161038006));
#71688=CARTESIAN_POINT('Ctrl Pts',(-0.159300830895344,0.175719928401452,
-0.809164248558111));
#71689=CARTESIAN_POINT('Ctrl Pts',(-0.160413198509322,0.174705047217267,
-0.809062789319625));
#71690=CARTESIAN_POINT('Ctrl Pts',(-0.163895048885713,0.171467052294824,
-0.808740974528823));
#71691=CARTESIAN_POINT('Ctrl Pts',(-0.166228466807851,0.169205886629669,
-0.808519000051947));
#71692=CARTESIAN_POINT('Ctrl Pts',(-0.18587961973296,0.149364341245727,
-0.806593439920735));
#71693=CARTESIAN_POINT('Ctrl Pts',(-0.200399580666512,0.129230042450441,
-0.804762652866216));
#71694=CARTESIAN_POINT('Ctrl Pts',(-0.213645103211607,0.103098002229832,
-0.802650700491467));
#71695=CARTESIAN_POINT('Ctrl Pts',(-0.215617582829886,0.0989064786785701,
-0.802319892744766));
#71696=CARTESIAN_POINT('Ctrl Pts',(-0.218249638930465,0.0928597287886012,
-0.801856286021236));
#71697=CARTESIAN_POINT('Ctrl Pts',(-0.21901076420458,0.0910500953094566,
-0.80171923952589));
#71698=CARTESIAN_POINT('Ctrl Pts',(-0.220320986606933,0.0878234136081048,
-0.801478129327539));
#71699=CARTESIAN_POINT('Ctrl Pts',(-0.220879090816275,0.0864101652535897,
-0.801373618372736));
#71700=CARTESIAN_POINT('Ctrl Pts',(-0.221707476869052,0.0842520201662678,
-0.801215781523344));
#71701=CARTESIAN_POINT('Ctrl Pts',(-0.221987658619029,0.0835110032798849,
-0.801161900226131));
#71702=CARTESIAN_POINT('Ctrl Pts',(-0.222492744930583,0.0821546605187406,
-0.801063866257287));
#71703=CARTESIAN_POINT('Ctrl Pts',(-0.222718814786106,0.0815398022730665,
-0.80101964736757));
#71704=CARTESIAN_POINT('Ctrl Pts',(-0.223223458488964,0.0801495291375546,
-0.800920158752538));
#71705=CARTESIAN_POINT('Ctrl Pts',(-0.223500541595484,0.079373593837259,
-0.800864977050514));
#71706=CARTESIAN_POINT('Ctrl Pts',(-0.224207063465765,0.07736203479027,
-0.800722773509264));
#71707=CARTESIAN_POINT('Ctrl Pts',(-0.224630340348941,0.0761242544753688,
-0.800636098483587));
#71708=CARTESIAN_POINT('Ctrl Pts',(-0.227522305359091,0.0674331292638725,
-0.800032864484715));
#71709=CARTESIAN_POINT('Ctrl Pts',(-0.229630071510987,0.0598638830467814,
-0.799534926892895));
#71710=CARTESIAN_POINT('Ctrl Pts',(-0.235212554831166,0.0351229649092346,
-0.797953706516104));
#71711=CARTESIAN_POINT('Ctrl Pts',(-0.237163286780622,0.0176685248323082,
-0.796904759483021));
#71712=CARTESIAN_POINT('Ctrl Pts',(-0.237180144425426,-0.00764632315616661,
-0.795317854475676));
#71713=CARTESIAN_POINT('Ctrl Pts',(-0.23680014498452,-0.0154453587996077,
-0.794820676130295));
#71714=CARTESIAN_POINT('Ctrl Pts',(-0.235824625894277,-0.0253656065722973,
-0.794170228461875));
#71715=CARTESIAN_POINT('Ctrl Pts',(-0.235583254857002,-0.0275172254358308,
-0.794028076089512));
#71716=CARTESIAN_POINT('Ctrl Pts',(-0.235149632666643,-0.0309568372463856,
-0.793798966127605));
#71717=CARTESIAN_POINT('Ctrl Pts',(-0.234976167756467,-0.0322471081999229,
-0.793712601073455));
#71718=CARTESIAN_POINT('Ctrl Pts',(-0.234626242819097,-0.0346970110183,
-0.793547784177764));
#71719=CARTESIAN_POINT('Ctrl Pts',(-0.234451785053246,-0.0358568932435544,
-0.79346939792067));
#71720=CARTESIAN_POINT('Ctrl Pts',(-0.23403380056031,-0.0385022963889381,
-0.793289783459555));
#71721=CARTESIAN_POINT('Ctrl Pts',(-0.233784721948673,-0.0399868757635025,
-0.793188382140547));
#71722=CARTESIAN_POINT('Ctrl Pts',(-0.232969186852884,-0.0445793476358548,
-0.792872776912732));
#71723=CARTESIAN_POINT('Ctrl Pts',(-0.232354777014379,-0.0476782568799442,
-0.792657066319692));
#71724=CARTESIAN_POINT('Ctrl Pts',(-0.230780367643786,-0.0548636285042661,
-0.792150248702046));
#71725=CARTESIAN_POINT('Ctrl Pts',(-0.22977343644788,-0.0589386120441784,
-0.791857745655845));
#71726=CARTESIAN_POINT('Ctrl Pts',(-0.225682199945196,-0.0737914333972743,
-0.790772796770028));
#71727=CARTESIAN_POINT('Ctrl Pts',(-0.221943348726598,-0.0843725728000726,
-0.789962176969947));
#71728=CARTESIAN_POINT('Ctrl Pts',(-0.21140519444329,-0.108585723379124,
-0.788035927796551));
#71729=CARTESIAN_POINT('Ctrl Pts',(-0.204013255533633,-0.121908505732966,
-0.786917862671433));
#71730=CARTESIAN_POINT('Ctrl Pts',(-0.194254849949772,-0.136092212219059,
-0.785718376341118));
#71731=CARTESIAN_POINT('Ctrl Pts',(-0.193092140386242,-0.137736933875552,
-0.785579177629066));
#71732=CARTESIAN_POINT('Ctrl Pts',(-0.191392931678547,-0.140076751716148,
-0.785381220564546));
#71733=CARTESIAN_POINT('Ctrl Pts',(-0.190873343445992,-0.140783939039688,
-0.785321399383733));
#71734=CARTESIAN_POINT('Ctrl Pts',(-0.189955189132845,-0.142019169039291,
-0.785216950935694));
#71735=CARTESIAN_POINT('Ctrl Pts',(-0.189558321272216,-0.142548451881185,
-0.785172209657846));
#71736=CARTESIAN_POINT('Ctrl Pts',(-0.188709587452447,-0.14367055299265,
-0.785077392645125));
#71737=CARTESIAN_POINT('Ctrl Pts',(-0.1882571376529,-0.144262907065752,
-0.78502735826662));
#71738=CARTESIAN_POINT('Ctrl Pts',(-0.187008078339073,-0.145882310860354,
-0.784890594596281));
#71739=CARTESIAN_POINT('Ctrl Pts',(-0.186205792651359,-0.146904979354377,
-0.784804252124217));
#71740=CARTESIAN_POINT('Ctrl Pts',(-0.181682688967277,-0.152573959247149,
-0.784325439745302));
#71741=CARTESIAN_POINT('Ctrl Pts',(-0.177796047330419,-0.15708593701531,
-0.783943621767476));
#71742=CARTESIAN_POINT('Ctrl Pts',(-0.16565224695839,-0.17015462988163,
-0.782818741546131));
#71743=CARTESIAN_POINT('Ctrl Pts',(-0.156917501334763,-0.178241965996434,
-0.782095878856134));
#71744=CARTESIAN_POINT('Ctrl Pts',(-0.135783087408427,-0.195047055222898,
-0.780439296513251));
#71745=CARTESIAN_POINT('Ctrl Pts',(-0.123083164659989,-0.203299894677737,
-0.779503880942169));
#71746=CARTESIAN_POINT('Ctrl Pts',(-0.107560955247797,-0.211396223314265,
-0.778364632025009));
#71747=CARTESIAN_POINT('Ctrl Pts',(-0.10541980478391,-0.212472083811336,
-0.778207642154079));
#71748=CARTESIAN_POINT('Ctrl Pts',(-0.102033058506635,-0.214110022020128,
-0.777959383267467));
#71749=CARTESIAN_POINT('Ctrl Pts',(-0.100798240656284,-0.214694110552981,
-0.777868879819812));
#71750=CARTESIAN_POINT('Ctrl Pts',(-0.0985108045338502,-0.215752020577913,
-0.777701215433239));
#71751=CARTESIAN_POINT('Ctrl Pts',(-0.0974596344063058,-0.216228889313234,
-0.777624162451613));
#71752=CARTESIAN_POINT('Ctrl Pts',(-0.0951190938234653,-0.217270153421073,
-0.777452564706434));
#71753=CARTESIAN_POINT('Ctrl Pts',(-0.0938281044018087,-0.217830778939077,
-0.777357894339669));
#71754=CARTESIAN_POINT('Ctrl Pts',(-0.0900813404126108,-0.21941836303876,
-0.777083035097977));
#71755=CARTESIAN_POINT('Ctrl Pts',(-0.0876132378049596,-0.220415483766243,
-0.776901848048038));
#71756=CARTESIAN_POINT('Ctrl Pts',(-0.0819864812091353,-0.222579273663771,
-0.776488332456942));
#71757=CARTESIAN_POINT('Ctrl Pts',(-0.0788187701944008,-0.223720619645481,
-0.776255217364598));
#71758=CARTESIAN_POINT('Ctrl Pts',(-0.068183827309296,-0.227298556717051,
-0.775471375879996));
#71759=CARTESIAN_POINT('Ctrl Pts',(-0.0606205702085482,-0.229431457529129,
-0.774911770987888));
#71760=CARTESIAN_POINT('Ctrl Pts',(-0.0366642910276418,-0.234920003276817,
-0.773137545533251));
#71761=CARTESIAN_POINT('Ctrl Pts',(-0.0200138367804017,-0.236920051691439,
-0.771898566770572));
#71762=CARTESIAN_POINT('Ctrl Pts',(0.00138735010707077,-0.237217102158682,
-0.77037261576576));
#71763=CARTESIAN_POINT('Ctrl Pts',(0.00606768302189341,-0.237143561159798,
-0.770043264992721));
#71764=CARTESIAN_POINT('Ctrl Pts',(0.0119989879116246,-0.236874619439597,
-0.769633834273039));
#71765=CARTESIAN_POINT('Ctrl Pts',(0.0132544077875595,-0.236807689686453,
-0.769547627852372));
#71766=CARTESIAN_POINT('Ctrl Pts',(0.0152439140481402,-0.236685752503537,
-0.769411794975062));
#71767=CARTESIAN_POINT('Ctrl Pts',(0.0159783568812277,-0.236637305813183,
-0.769361820135098));
#71768=CARTESIAN_POINT('Ctrl Pts',(0.0173752056995839,-0.236538631353395,
-0.769267108875787));
#71769=CARTESIAN_POINT('Ctrl Pts',(0.018037622085949,-0.236489040117381,
-0.769222340795759));
#71770=CARTESIAN_POINT('Ctrl Pts',(0.0196088924895617,-0.23636476788746,
-0.76911648222918));
#71771=CARTESIAN_POINT('Ctrl Pts',(0.020517537455653,-0.236287627455589,
-0.769055528749612));
#71772=CARTESIAN_POINT('Ctrl Pts',(0.0235752021646285,-0.236010272441571,
-0.768851233137706));
#71773=CARTESIAN_POINT('Ctrl Pts',(0.025722002965479,-0.235785958505809,
-0.768709157500939));
#71774=CARTESIAN_POINT('Ctrl Pts',(0.0309463351775337,-0.235167874391955,
-0.768366076001241));
#71775=CARTESIAN_POINT('Ctrl Pts',(0.0340198437549295,-0.234742959341649,
-0.768166500696405));
#71776=CARTESIAN_POINT('Ctrl Pts',(0.0465105498680658,-0.232765613220388,
-0.767361448000405));
#71777=CARTESIAN_POINT('Ctrl Pts',(0.0558389099304648,-0.230705669643688,
-0.76677398915997));
#71778=CARTESIAN_POINT('Ctrl Pts',(0.0821653963619249,-0.223201121231705,
-0.765094776298149));
#71779=CARTESIAN_POINT('Ctrl Pts',(0.0987045106109589,-0.216395996570317,
-0.764009004681878));
#71780=CARTESIAN_POINT('Ctrl Pts',(0.117051434692432,-0.206302278211669,
-0.762655019819878));
#71781=CARTESIAN_POINT('Ctrl Pts',(0.119748577671364,-0.204748492142824,
-0.762452034871108));
#71782=CARTESIAN_POINT('Ctrl Pts',(0.123696065740999,-0.2023697200352,-0.76214863539994));
#71783=CARTESIAN_POINT('Ctrl Pts',(0.12497050124483,-0.201585202613731,
-0.762049687231038));
#71784=CARTESIAN_POINT('Ctrl Pts',(0.127229534549637,-0.200164930909991,
-0.761872461863766));
#71785=CARTESIAN_POINT('Ctrl Pts',(0.128217013836075,-0.199533834991098,
-0.76179435843368));
#71786=CARTESIAN_POINT('Ctrl Pts',(0.130295619607261,-0.198183601191193,
-0.761628584669387));
#71787=CARTESIAN_POINT('Ctrl Pts',(0.131385557361585,-0.197462714121037,
-0.761540850765289));
#71788=CARTESIAN_POINT('Ctrl Pts',(0.13428402856137,-0.195511037583469,
-0.76130533267886));
#71789=CARTESIAN_POINT('Ctrl Pts',(0.136081547192064,-0.194264196644445,
-0.761156946289835));
#71790=CARTESIAN_POINT('Ctrl Pts',(0.145324380039627,-0.187661714471184,
-0.760381521457689));
#71791=CARTESIAN_POINT('Ctrl Pts',(0.15247079473486,-0.181903031942176,
-0.759739059063353));
#71792=CARTESIAN_POINT('Ctrl Pts',(0.167258594018503,-0.168501960438982,
-0.758312872807955));
#71793=CARTESIAN_POINT('Ctrl Pts',(0.174747960349115,-0.160721707881131,
-0.757525643633148));
#71794=CARTESIAN_POINT('Ctrl Pts',(0.189473955934466,-0.143173183720772,
-0.755852602057995));
#71795=CARTESIAN_POINT('Ctrl Pts',(0.196543959832642,-0.133302179247616,
-0.754968974044639));
#71796=CARTESIAN_POINT('Ctrl Pts',(0.203903224972589,-0.12116003208253,
-0.753978558229908));
#71797=CARTESIAN_POINT('Ctrl Pts',(0.204954532321896,-0.119373024341003,
-0.75383511614973));
#71798=CARTESIAN_POINT('Ctrl Pts',(0.206395395817321,-0.116848686716007,
-0.753635959380549));
#71799=CARTESIAN_POINT('Ctrl Pts',(0.206804666710838,-0.116122800866511,
-0.75357908777217));
#71800=CARTESIAN_POINT('Ctrl Pts',(0.207537019219195,-0.114807742493401,
-0.753476791229729));
#71801=CARTESIAN_POINT('Ctrl Pts',(0.207861438405948,-0.114219326504537,
-0.753431283184742));
#71802=CARTESIAN_POINT('Ctrl Pts',(0.208520776711208,-0.113011337095497,
-0.753338408759164));
#71803=CARTESIAN_POINT('Ctrl Pts',(0.208855443643762,-0.112391638148354,
-0.753291058174916));
#71804=CARTESIAN_POINT('Ctrl Pts',(0.209711971748914,-0.110788577148183,
-0.753169302660511));
#71805=CARTESIAN_POINT('Ctrl Pts',(0.210229686168149,-0.109803001310291,
-0.753095154044283));
#71806=CARTESIAN_POINT('Ctrl Pts',(0.212416881293943,-0.105567044785309,
-0.752779327927861));
#71807=CARTESIAN_POINT('Ctrl Pts',(0.214018166330394,-0.102281769879419,
-0.752541552658432));
#71808=CARTESIAN_POINT('Ctrl Pts',(0.218262422481726,-0.0930374869733026,
-0.751888592095682));
#71809=CARTESIAN_POINT('Ctrl Pts',(0.220736748892215,-0.0870043621872726,
-0.751480614530072));
#71810=CARTESIAN_POINT('Ctrl Pts',(0.224351678549712,-0.0770387673838556,
-0.75082422009093));
#71811=CARTESIAN_POINT('Ctrl Pts',(0.225644509273265,-0.0731655928764686,
-0.750573275346606));
#71812=CARTESIAN_POINT('Ctrl Pts',(0.23207617779094,-0.0521012059392833,
-0.749222144811371));
#71813=CARTESIAN_POINT('Ctrl Pts',(0.235351080179665,-0.0344045320088943,
-0.748130029713232));
#71814=CARTESIAN_POINT('Ctrl Pts',(0.236815860574844,-0.0134114833652199,
-0.746769236584495));
#71815=CARTESIAN_POINT('Ctrl Pts',(0.236971119992029,-0.0103105061208107,
-0.746566752093371));
#71816=CARTESIAN_POINT('Ctrl Pts',(0.237110894074801,-0.00571311970649749,
-0.746263957822327));
#71817=CARTESIAN_POINT('Ctrl Pts',(0.237142195492225,-0.00421838483763519,
-0.746165105732175));
#71818=CARTESIAN_POINT('Ctrl Pts',(0.237172817898998,-0.00155180218573925,
-0.745987987014976));
#71819=CARTESIAN_POINT('Ctrl Pts',(0.237177589818882,-0.000380056957058218,
-0.745909893355406));
#71820=CARTESIAN_POINT('Ctrl Pts',(0.237169314132987,0.00209926562713611,
-0.745744071475447));
#71821=CARTESIAN_POINT('Ctrl Pts',(0.237154135813141,0.00340679178762933,
-0.745656279172044));
#71822=CARTESIAN_POINT('Ctrl Pts',(0.237084588507573,0.00690515043165489,
-0.745420436544233));
#71823=CARTESIAN_POINT('Ctrl Pts',(0.237010666314697,0.00909542197051881,
-0.745271781106377));
#71824=CARTESIAN_POINT('Ctrl Pts',(0.236467160639718,0.0205059716707322,
-0.74449190855852));
#71825=CARTESIAN_POINT('Ctrl Pts',(0.23548992133616,0.0296929439342925,
-0.743845051711116));
#71826=CARTESIAN_POINT('Ctrl Pts',(0.232222271285833,0.0493989180236857,
-0.742417167169648));
#71827=CARTESIAN_POINT('Ctrl Pts',(0.229746314823503,0.0598668264034082,
-0.741632966265385));
#71828=CARTESIAN_POINT('Ctrl Pts',(0.222993397439967,0.0816835169848657,
-0.739965103043221));
#71829=CARTESIAN_POINT('Ctrl Pts',(0.218538399404636,0.0929477197894774,
-0.739083619651619));
#71830=CARTESIAN_POINT('Ctrl Pts',(0.212334754689178,0.105689345775776,
-0.738095043383589));
#71831=CARTESIAN_POINT('Ctrl Pts',(0.211401979785314,0.107542965995895,
-0.737951476823557));
#71832=CARTESIAN_POINT('Ctrl Pts',(0.210060509430596,0.110123829765267,
-0.737752176735345));
#71833=CARTESIAN_POINT('Ctrl Pts',(0.20967215492571,0.110861458613419,-0.737695284173697));
#71834=CARTESIAN_POINT('Ctrl Pts',(0.208963725047883,0.112189989770339,
-0.737592961152486));
#71835=CARTESIAN_POINT('Ctrl Pts',(0.208645012611117,0.112781607292701,
-0.737547447449598));
#71836=CARTESIAN_POINT('Ctrl Pts',(0.20798718759458,0.113990377936833,-0.737454575169175));
#71837=CARTESIAN_POINT('Ctrl Pts',(0.207647834352599,0.114607388013562,
-0.737407232293775));
#71838=CARTESIAN_POINT('Ctrl Pts',(0.20676516858516,0.116195455081041,-0.737285520117831));
#71839=CARTESIAN_POINT('Ctrl Pts',(0.206217753878216,0.117164230158201,
-0.737211406783946));
#71840=CARTESIAN_POINT('Ctrl Pts',(0.203846083520035,0.121293322195744,
-0.736895945296159));
#71841=CARTESIAN_POINT('Ctrl Pts',(0.201955735872948,0.12441535305541,-0.736658488209435));
#71842=CARTESIAN_POINT('Ctrl Pts',(0.196497789346405,0.132977068637876,
-0.736006692388246));
#71843=CARTESIAN_POINT('Ctrl Pts',(0.192777233486394,0.138315698649986,
-0.735599530363658));
#71844=CARTESIAN_POINT('Ctrl Pts',(0.186302966032496,0.146835937303549,
-0.734936899362414));
#71845=CARTESIAN_POINT('Ctrl Pts',(0.183676008044094,0.150109003713227,
-0.73467901485996));
#71846=CARTESIAN_POINT('Ctrl Pts',(0.169434227018847,0.166919593031269,
-0.733327529406232));
#71847=CARTESIAN_POINT('Ctrl Pts',(0.156408104585745,0.179182944241944,
-0.732241415382019));
#71848=CARTESIAN_POINT('Ctrl Pts',(0.139639943991141,0.191735108537672,
-0.730887062536924));
#71849=CARTESIAN_POINT('Ctrl Pts',(0.137112189406538,0.193550799147673,
-0.730684103838247));
#71850=CARTESIAN_POINT('Ctrl Pts',(0.133317178915064,0.196165108620653,
-0.730380736108378));
#71851=CARTESIAN_POINT('Ctrl Pts',(0.132076840821975,0.197002355264635,
-0.730281792975631));
#71852=CARTESIAN_POINT('Ctrl Pts',(0.129851192166905,0.198474234852637,
-0.730104573201188));
#71853=CARTESIAN_POINT('Ctrl Pts',(0.128868935627575,0.199113413292776,
-0.730026470285796));
#71854=CARTESIAN_POINT('Ctrl Pts',(0.126781418701622,0.200449894630835,
-0.729860694011883));
#71855=CARTESIAN_POINT('Ctrl Pts',(0.125675054844796,0.201145392332424,
-0.729772957056639));
#71856=CARTESIAN_POINT('Ctrl Pts',(0.122701251540261,0.202980713135329,
-0.729537422015438));
#71857=CARTESIAN_POINT('Ctrl Pts',(0.120823731666818,0.20410387634948,-0.729389021571073));
#71858=CARTESIAN_POINT('Ctrl Pts',(0.110993313989625,0.209801422119215,
-0.728613365447377));
#71859=CARTESIAN_POINT('Ctrl Pts',(0.102796405199097,0.213936937621227,
-0.727970674637133));
#71860=CARTESIAN_POINT('Ctrl Pts',(0.0844870568284945,0.221878881640529,
-0.72654439865347));
#71861=CARTESIAN_POINT('Ctrl Pts',(0.0743120169870806,0.225490563302023,
-0.725757325414621));
#71862=CARTESIAN_POINT('Ctrl Pts',(0.0522547619520863,0.23166429202892,
-0.724084552656099));
#71863=CARTESIAN_POINT('Ctrl Pts',(0.0403476740833811,0.234032109241221,
-0.723201037244923));
#71864=CARTESIAN_POINT('Ctrl Pts',(0.0262523252851681,0.235726736509283,
-0.722210718470013));
#71865=CARTESIAN_POINT('Ctrl Pts',(0.0241906777440488,0.235947220220347,
-0.722067270279137));
#71866=CARTESIAN_POINT('Ctrl Pts',(0.0212966450340585,0.236218390344216,
-0.721868106474055));
#71867=CARTESIAN_POINT('Ctrl Pts',(0.0204665518706763,0.236291758920337,
-0.721811233836736));
#71868=CARTESIAN_POINT('Ctrl Pts',(0.0189664703592798,0.236416380756957,
-0.721708935994121));
#71869=CARTESIAN_POINT('Ctrl Pts',(0.0182966193840366,0.236469164686944,
-0.721663427671397));
#71870=CARTESIAN_POINT('Ctrl Pts',(0.0169242129664499,0.236571442992661,
-0.721570553351657));
#71871=CARTESIAN_POINT('Ctrl Pts',(0.016221647217112,0.236620655942528,
-0.721523203146354));
#71872=CARTESIAN_POINT('Ctrl Pts',(0.0144080362414379,0.236739579187792,
-0.721401449762246));
#71873=CARTESIAN_POINT('Ctrl Pts',(0.0132966850958709,0.236804599088722,
-0.721327302880291));
#71874=CARTESIAN_POINT('Ctrl Pts',(0.00853595339270665,0.237049505589593,
-0.721011494697443));
#71875=CARTESIAN_POINT('Ctrl Pts',(0.00488291993516837,0.237152885832268,
-0.720773735077856));
#71876=CARTESIAN_POINT('Ctrl Pts',(-0.00528807153497601,0.237205578827938,
-0.720120831828304));
#71877=CARTESIAN_POINT('Ctrl Pts',(-0.0118039747893253,0.236970734068871,
-0.71971289439808));
#71878=CARTESIAN_POINT('Ctrl Pts',(-0.0195876596812752,0.236368284890876,
-0.719229498985646));
#71879=CARTESIAN_POINT('Ctrl Pts',(-0.0208721358349881,0.236258325801489,
-0.719149858254532));
#71880=CARTESIAN_POINT('Ctrl Pts',(-0.0287900959476827,0.235515422430361,
-0.718659407888492));
#71881=CARTESIAN_POINT('Ctrl Pts',(-0.0353904170704665,0.234614090579963,
-0.718252580103505));
#71882=CARTESIAN_POINT('Ctrl Pts',(-0.04193932278856,0.233437515898874,
-0.717844391575082));
#71883=CARTESIAN_POINT('Origin',(0.,0.,-2.1456589891905));
#71884=CARTESIAN_POINT('',(-0.0419766262164045,0.23365534329502,-0.598123480850464));
#71885=CARTESIAN_POINT('',(-0.0418741542966648,0.233068851607476,-0.617833934840082));
#71886=CARTESIAN_POINT('',(-0.0419392741328076,0.233437524640348,-2.1456589891905));
#71887=CARTESIAN_POINT('',(-0.237249110971816,-5.32523605593984E-5,-0.675941014918504));
#71888=CARTESIAN_POINT('Ctrl Pts',(-0.237550249404384,-5.3380897644477E-5,
-0.675941010809497));
#71889=CARTESIAN_POINT('Ctrl Pts',(-0.237559050867073,-0.00294060675479713,
-0.675746408192839));
#71890=CARTESIAN_POINT('Ctrl Pts',(-0.236202859689124,-0.084373458259399,
-0.670257162218186));
#71891=CARTESIAN_POINT('Ctrl Pts',(-0.143209357946364,-0.241037317324593,
-0.659473272885537));
#71892=CARTESIAN_POINT('Ctrl Pts',(0.124952039551137,-0.250987841057003,
-0.643589342811547));
#71893=CARTESIAN_POINT('Ctrl Pts',(0.278649891841477,-0.0310184835734619,
-0.62770541273756));
#71894=CARTESIAN_POINT('Ctrl Pts',(0.181746723461027,0.20597154716017,-0.612550125417199));
#71895=CARTESIAN_POINT('Ctrl Pts',(0.0249201733156075,0.245060147532978,
-0.602689481454833));
#71896=CARTESIAN_POINT('Ctrl Pts',(-0.0419766262164012,0.23365534329502,
-0.598123480850464));
#71897=CARTESIAN_POINT('Ctrl Pts',(-0.0419392741328079,0.233437524640348,
-0.698115075114807));
#71898=CARTESIAN_POINT('Ctrl Pts',(-0.0558502647186398,0.230938282718824,
-0.697169413870174));
#71899=CARTESIAN_POINT('Ctrl Pts',(-0.0695303812972798,0.227192518435731,
-0.696223752625541));
#71900=CARTESIAN_POINT('Ctrl Pts',(-0.0827484893710936,0.222271608919812,
-0.695278091380908));
#71901=CARTESIAN_POINT('Ctrl Pts',(-0.0959969028860838,0.217339417128622,
-0.694330261998364));
#71902=CARTESIAN_POINT('Ctrl Pts',(-0.108780430948953,0.211227046017747,
-0.69338243261582));
#71903=CARTESIAN_POINT('Ctrl Pts',(-0.120888672191277,0.204053692838012,
-0.692434603233277));
#71904=CARTESIAN_POINT('Ctrl Pts',(-0.125970748973033,0.201042889624525,
-0.692036779833355));
#71905=CARTESIAN_POINT('Ctrl Pts',(-0.130934198668081,0.197845717141427,
-0.691638956433434));
#71906=CARTESIAN_POINT('Ctrl Pts',(-0.135765095923163,0.194473184151375,
-0.691241133033512));
#71907=CARTESIAN_POINT('Ctrl Pts',(-0.147207302363418,0.186485181786356,
-0.690298869675731));
#71908=CARTESIAN_POINT('Ctrl Pts',(-0.157982935539225,0.177455254709155,
-0.689356606317951));
#71909=CARTESIAN_POINT('Ctrl Pts',(-0.167896362767565,0.167519527203315,
-0.68841434296017));
#71910=CARTESIAN_POINT('Ctrl Pts',(-0.177789727932494,0.157603906890545,
-0.687473986485529));
#71911=CARTESIAN_POINT('Ctrl Pts',(-0.186823707031258,0.146786664065463,
-0.686533630010888));
#71912=CARTESIAN_POINT('Ctrl Pts',(-0.194836192693097,0.135243626991657,
-0.685593273536246));
#71913=CARTESIAN_POINT('Ctrl Pts',(-0.202847293896005,0.123702584412623,
-0.684653079543633));
#71914=CARTESIAN_POINT('Ctrl Pts',(-0.209836731309494,0.111436662316105,
-0.683712885551019));
#71915=CARTESIAN_POINT('Ctrl Pts',(-0.215683815247096,0.0986532942453341,
-0.682772691558406));
#71916=CARTESIAN_POINT('Ctrl Pts',(-0.221530259604519,0.085871324476509,
-0.681832600408414));
#71917=CARTESIAN_POINT('Ctrl Pts',(-0.226234267631766,0.0725727996398668,
-0.680892509258422));
#71918=CARTESIAN_POINT('Ctrl Pts',(-0.22972296895733,0.0589859149155935,
-0.67995241810843));
#71919=CARTESIAN_POINT('Ctrl Pts',(-0.233219408844369,0.0453688920588515,
-0.679010241668677));
#71920=CARTESIAN_POINT('Ctrl Pts',(-0.235495005835672,0.031463065700045,
-0.678068065228924));
#71921=CARTESIAN_POINT('Ctrl Pts',(-0.236527988038831,0.0175068986203395,
-0.677125888789171));
#71922=CARTESIAN_POINT('Ctrl Pts',(-0.236961011170192,0.0116565140230217,
-0.676730931169388));
#71923=CARTESIAN_POINT('Ctrl Pts',(-0.237176306855964,0.0057973155111871,
-0.676335973549606));
#71924=CARTESIAN_POINT('Ctrl Pts',(-0.237174994028786,-5.32207246910343E-5,
-0.675941015929823));
#71925=CARTESIAN_POINT('',(-0.236922073620166,-0.000171722348330205,-0.695658869404682));
#71926=CARTESIAN_POINT('Ctrl Pts',(-0.0419393227885598,0.233437515898874,
-0.717844391575082));
#71927=CARTESIAN_POINT('Ctrl Pts',(-0.0525772381988217,0.231526310810564,
-0.717181338047711));
#71928=CARTESIAN_POINT('Ctrl Pts',(-0.0630794614327931,0.228888870292117,
-0.716514194660857));
#71929=CARTESIAN_POINT('Ctrl Pts',(-0.0784769135198977,0.223879812165597,
-0.715485132150475));
#71930=CARTESIAN_POINT('Ctrl Pts',(-0.0835234147063496,0.222046455704396,
-0.715139446381879));
#71931=CARTESIAN_POINT('Ctrl Pts',(-0.0902667636855455,0.219334232894479,
-0.714663706665366));
#71932=CARTESIAN_POINT('Ctrl Pts',(-0.0920217966268213,0.218603712097245,
-0.714538598478205));
#71933=CARTESIAN_POINT('Ctrl Pts',(-0.094911247513511,0.217360036274781,
-0.714330382191779));
#71934=CARTESIAN_POINT('Ctrl Pts',(-0.096050766332457,0.216858895275677,
-0.714247684029168));
#71935=CARTESIAN_POINT('Ctrl Pts',(-0.0982536957775581,0.215869315121601,
-0.714086649331944));
#71936=CARTESIAN_POINT('Ctrl Pts',(-0.0993175423839966,0.215381929685326,
-0.714008350839327));
#71937=CARTESIAN_POINT('Ctrl Pts',(-0.101816139978379,0.214214786549096,
-0.713823177228744));
#71938=CARTESIAN_POINT('Ctrl Pts',(-0.103247743320399,0.213528462791111,
-0.713716077567042));
#71939=CARTESIAN_POINT('Ctrl Pts',(-0.106274126753787,0.212040036360264,
-0.713487490500992));
#71940=CARTESIAN_POINT('Ctrl Pts',(-0.107866950573482,0.211234201083342,
-0.713365878117769));
#71941=CARTESIAN_POINT('Ctrl Pts',(-0.112194423789506,0.208983153241751,
-0.713031836171442));
#71942=CARTESIAN_POINT('Ctrl Pts',(-0.114910058565981,0.20750234689232,
-0.712818188320758));
#71943=CARTESIAN_POINT('Ctrl Pts',(-0.12359230955118,0.202545304209228,
-0.712121831197764));
#71944=CARTESIAN_POINT('Ctrl Pts',(-0.129435881053669,0.198861753509653,
-0.711632298097665));
#71945=CARTESIAN_POINT('Ctrl Pts',(-0.146848509522171,0.18679262807147,
-0.710110421114418));
#71946=CARTESIAN_POINT('Ctrl Pts',(-0.157827755137984,0.177612865934884,
-0.709058205538637));
#71947=CARTESIAN_POINT('Ctrl Pts',(-0.173745697236007,0.161655828076908,
-0.707424676793536));
#71948=CARTESIAN_POINT('Ctrl Pts',(-0.179269133818743,0.15550814152815,
-0.706833561518333));
#71949=CARTESIAN_POINT('Ctrl Pts',(-0.185293390317587,0.148054359499175,
-0.706170516244241));
#71950=CARTESIAN_POINT('Ctrl Pts',(-0.186117081652261,0.147017570306768,
-0.706079431164925));
#71951=CARTESIAN_POINT('Ctrl Pts',(-0.18744211413612,0.145320752922566,
-0.70593227814894));
#71952=CARTESIAN_POINT('Ctrl Pts',(-0.187948741383397,0.144664916433839,
-0.705875860986625));
#71953=CARTESIAN_POINT('Ctrl Pts',(-0.188849815647416,0.143485738603242,
-0.705775263015471));
#71954=CARTESIAN_POINT('Ctrl Pts',(-0.189245540363652,0.142963406288722,
-0.70573099489097));
#71955=CARTESIAN_POINT('Ctrl Pts',(-0.190112414923563,0.141809278297383,
-0.70563382567623));
#71956=CARTESIAN_POINT('Ctrl Pts',(-0.190582583682373,0.141176770615792,
-0.705580992101311));
#71957=CARTESIAN_POINT('Ctrl Pts',(-0.191938226311698,0.139333939792885,
-0.705428233490907));
#71958=CARTESIAN_POINT('Ctrl Pts',(-0.192815404662887,0.138117520644432,
-0.705328858763159));
#71959=CARTESIAN_POINT('Ctrl Pts',(-0.201067174873499,0.126442612019581,
-0.70438802949425));
#71960=CARTESIAN_POINT('Ctrl Pts',(-0.20759658571956,0.115410124225476,
-0.703596580294805));
#71961=CARTESIAN_POINT('Ctrl Pts',(-0.217379569366901,0.0953358954136322,
-0.702225297712208));
#71962=CARTESIAN_POINT('Ctrl Pts',(-0.221034511834627,0.0865248539457959,
-0.701644391304448));
#71963=CARTESIAN_POINT('Ctrl Pts',(-0.226821574066829,0.0697911174599313,
-0.700546583455936));
#71964=CARTESIAN_POINT('Ctrl Pts',(-0.229092241183086,0.0619318411730688,
-0.70003312872163));
#71965=CARTESIAN_POINT('Ctrl Pts',(-0.231791079607705,0.0503830929441907,
-0.699270354435328));
#71966=CARTESIAN_POINT('Ctrl Pts',(-0.232545876430116,0.0467757801607365,
-0.69903099573463));
#71967=CARTESIAN_POINT('Ctrl Pts',(-0.233485612826743,0.0416970049545228,
-0.698691768909176));
#71968=CARTESIAN_POINT('Ctrl Pts',(-0.233741289376611,0.0402390493665929,
-0.698594133513378));
#71969=CARTESIAN_POINT('Ctrl Pts',(-0.234162304802007,0.0376987304661087,
-0.69842352928938));
#71970=CARTESIAN_POINT('Ctrl Pts',(-0.234333828634087,0.0366174269717644,
-0.698350757995416));
#71971=CARTESIAN_POINT('Ctrl Pts',(-0.234664109538308,0.0344378804321751,
-0.698203750531822));
#71972=CARTESIAN_POINT('Ctrl Pts',(-0.234822657843481,0.0333396341469533,
-0.698129509741804));
#71973=CARTESIAN_POINT('Ctrl Pts',(-0.235132043495524,0.0310847743760905,
-0.69797672650977));
#71974=CARTESIAN_POINT('Ctrl Pts',(-0.235282066727623,0.0299280815974099,
-0.697898160479516));
#71975=CARTESIAN_POINT('Ctrl Pts',(-0.235611435984668,0.0272329010515647,
-0.697714631259476));
#71976=CARTESIAN_POINT('Ctrl Pts',(-0.23578425320844,0.0256936841795304,
-0.69760946604402));
#71977=CARTESIAN_POINT('Ctrl Pts',(-0.236260645939362,0.0210399586476515,
-0.697290399551302));
#71978=CARTESIAN_POINT('Ctrl Pts',(-0.236517661084166,0.0179211345203719,
-0.697075070043448));
#71979=CARTESIAN_POINT('Ctrl Pts',(-0.237024664985002,0.00981110428418152,
-0.696511086020329));
#71980=CARTESIAN_POINT('Ctrl Pts',(-0.237178732709955,0.00481571997640742,
-0.696159699629818));
#71981=CARTESIAN_POINT('Ctrl Pts',(-0.237174931349867,-0.000180455495009113,
-0.695804408402709));
#71982=CARTESIAN_POINT('Ctrl Pts',(-0.236922073620166,-0.000171722348330205,
-0.695658869404682));
#71983=CARTESIAN_POINT('Ctrl Pts',(-0.23710552994315,-0.0279230387667656,
-0.693801110963438));
#71984=CARTESIAN_POINT('Ctrl Pts',(-0.219763942386725,-0.134543724728559,
-0.686648709164199));
#71985=CARTESIAN_POINT('Ctrl Pts',(-0.0618944900249994,-0.273453815725051,
-0.674201664006962));
#71986=CARTESIAN_POINT('Ctrl Pts',(0.196265018423904,-0.200219778676104,
-0.658317733932975));
#71987=CARTESIAN_POINT('Ctrl Pts',(0.274634025736058,0.056427556548666,
-0.642433803858986));
#71988=CARTESIAN_POINT('Ctrl Pts',(0.127477169071532,0.230553445971132,
-0.628939204161356));
#71989=CARTESIAN_POINT('Ctrl Pts',(0.000916701292335384,0.240640926964646,
-0.620739247821721));
#71990=CARTESIAN_POINT('Ctrl Pts',(-0.0418741542966648,0.233068851607476,
-0.617833934840082));
#71991=CARTESIAN_POINT('Origin',(0.,0.,-2.1456589891905));
#71992=CARTESIAN_POINT('',(-0.0419392658597717,0.233437526126678,-0.498199055407226));
#71993=CARTESIAN_POINT('',(-0.0419392867764624,0.233437522368795,-0.517737946518584));
#71994=CARTESIAN_POINT('',(-0.0419392741328076,0.233437524640348,-2.1456589891905));
#71995=CARTESIAN_POINT('',(-0.237113469260214,0.000216662027683377,-0.575941048797587));
#71996=CARTESIAN_POINT('Ctrl Pts',(-0.0419392658597717,0.233437526126678,
-0.498199055407226));
#71997=CARTESIAN_POINT('Ctrl Pts',(-0.0330765815721231,0.235029791426685,
-0.498854438470705));
#71998=CARTESIAN_POINT('Ctrl Pts',(-0.0241272490857351,0.236116612807205,
-0.499504144402303));
#71999=CARTESIAN_POINT('Ctrl Pts',(-0.0130677217538534,0.236823784124591,
-0.500277172715157));
#72000=CARTESIAN_POINT('Ctrl Pts',(-0.0109991115124832,0.236928871929854,
-0.500420471355373));
#72001=CARTESIAN_POINT('Ctrl Pts',(-0.00809678705350146,0.237038217874467,
-0.500619474195118));
#72002=CARTESIAN_POINT('Ctrl Pts',(-0.00726409450755453,0.23706519710254,
-0.500676332777726));
#72003=CARTESIAN_POINT('Ctrl Pts',(-0.00575949653870239,0.237106010941874,
-0.500778623293592));
#72004=CARTESIAN_POINT('Ctrl Pts',(-0.00508764283983578,0.237121378530362,
-0.500824138186445));
#72005=CARTESIAN_POINT('Ctrl Pts',(-0.00371111637288122,0.237147011101855,
-0.500917049062407));
#72006=CARTESIAN_POINT('Ctrl Pts',(-0.00300644900677803,0.237156991372071,
-0.500964429082569));
#72007=CARTESIAN_POINT('Ctrl Pts',(-0.00118724318088404,0.237174647232239,
-0.501086300569577));
#72008=CARTESIAN_POINT('Ctrl Pts',(-7.26606088802279E-5,0.237177607877993,
-0.501160534952242));
#72009=CARTESIAN_POINT('Ctrl Pts',(0.00470589197833913,0.23715661511272,
-0.501477101949923));
#72010=CARTESIAN_POINT('Ctrl Pts',(0.00836923808759544,0.23705561574805,
-0.501715510301296));
#72011=CARTESIAN_POINT('Ctrl Pts',(0.0185645961743475,0.236537862562508,
-0.50237074909836));
#72012=CARTESIAN_POINT('Ctrl Pts',(0.0250841369162542,0.235935591099632,
-0.502780312100465));
#72013=CARTESIAN_POINT('Ctrl Pts',(0.0353272638051378,0.234559864942448,
-0.503420156542185));
#72014=CARTESIAN_POINT('Ctrl Pts',(0.0390711110489085,0.233965371524756,
-0.503653233582996));
#72015=CARTESIAN_POINT('Ctrl Pts',(0.0607299183943161,0.229991720981356,
-0.505004501675264));
#72016=CARTESIAN_POINT('Ctrl Pts',(0.0782194597970318,0.224646267754523,
-0.506112968106125));
#72017=CARTESIAN_POINT('Ctrl Pts',(0.0977486194251004,0.216117307995706,
-0.507491241025893));
#72018=CARTESIAN_POINT('Ctrl Pts',(0.100549184772378,0.214828637353469,
-0.507692316454647));
#72019=CARTESIAN_POINT('Ctrl Pts',(0.104665970453112,0.212836178430527,
-0.50799342611889));
#72020=CARTESIAN_POINT('Ctrl Pts',(0.106002020615916,0.212173927885199,
-0.508092027097791));
#72021=CARTESIAN_POINT('Ctrl Pts',(0.10837654992391,0.210968900284615,-0.508268891060408));
#72022=CARTESIAN_POINT('Ctrl Pts',(0.109417427998987,0.210430938376974,
-0.508346983331399));
#72023=CARTESIAN_POINT('Ctrl Pts',(0.111614078733411,0.209274928684104,
-0.508513008840907));
#72024=CARTESIAN_POINT('Ctrl Pts',(0.11276879609338,0.208654970837369,-0.508601007747302));
#72025=CARTESIAN_POINT('Ctrl Pts',(0.115851424522281,0.206966871045782,
-0.508837912523622));
#72026=CARTESIAN_POINT('Ctrl Pts',(0.117769643695447,0.205881394802806,
-0.508987432739999));
#72027=CARTESIAN_POINT('Ctrl Pts',(0.127808849002608,0.200014229300171,
-0.509781371131358));
#72028=CARTESIAN_POINT('Ctrl Pts',(0.135653579611324,0.194778999945319,
-0.510442120254722));
#72029=CARTESIAN_POINT('Ctrl Pts',(0.151622159419223,0.182688849587316,
-0.511875072709876));
#72030=CARTESIAN_POINT('Ctrl Pts',(0.159639408522314,0.175726280999964,
-0.512649399976805));
#72031=CARTESIAN_POINT('Ctrl Pts',(0.175680572604679,0.159788836753034,
-0.514300754108403));
#72032=CARTESIAN_POINT('Ctrl Pts',(0.183543925188247,0.150691144616251,
-0.515175619417615));
#72033=CARTESIAN_POINT('Ctrl Pts',(0.191922873303588,0.139362565664156,
-0.516158618663595));
#72034=CARTESIAN_POINT('Ctrl Pts',(0.193138709285569,0.137672632432337,
-0.516302662351488));
#72035=CARTESIAN_POINT('Ctrl Pts',(0.194810822616322,0.1352827449943,-0.516502522896911));
#72036=CARTESIAN_POINT('Ctrl Pts',(0.195285851047047,0.134596114859929,
-0.516559506804667));
#72037=CARTESIAN_POINT('Ctrl Pts',(0.196136935793519,0.133351922700136,
-0.51666195571733));
#72038=CARTESIAN_POINT('Ctrl Pts',(0.196514264588357,0.132795243604197,
-0.516707504473968));
#72039=CARTESIAN_POINT('Ctrl Pts',(0.197281753623912,0.131652519729256,
-0.516800402628193));
#72040=CARTESIAN_POINT('Ctrl Pts',(0.197671680390599,0.131066330796504,
-0.516847736625924));
#72041=CARTESIAN_POINT('Ctrl Pts',(0.198670378150646,0.129550362863303,
-0.516969349353387));
#72042=CARTESIAN_POINT('Ctrl Pts',(0.199275243310086,0.128618012725329,
-0.517043373072305));
#72043=CARTESIAN_POINT('Ctrl Pts',(0.201829928385638,0.124618887732487,
-0.517357764837771));
#72044=CARTESIAN_POINT('Ctrl Pts',(0.203715794467464,0.121511586970772,
-0.517594275163542));
#72045=CARTESIAN_POINT('Ctrl Pts',(0.208754956328711,0.112761335227541,
-0.518242569833834));
#72046=CARTESIAN_POINT('Ctrl Pts',(0.211750261286401,0.107030787268048,
-0.51864727141038));
#72047=CARTESIAN_POINT('Ctrl Pts',(0.216390444679063,0.0971937611344773,
-0.519320912665028));
#72048=CARTESIAN_POINT('Ctrl Pts',(0.2181612670776,0.0931510321216165,-0.519592032955327));
#72049=CARTESIAN_POINT('Ctrl Pts',(0.226449597120232,0.0726940099749962,
-0.52094576261472));
#72050=CARTESIAN_POINT('Ctrl Pts',(0.231231490981726,0.0556394799885956,
-0.522021834560969));
#72051=CARTESIAN_POINT('Ctrl Pts',(0.234579677202807,0.0351299650828139,
-0.523365391825341));
#72052=CARTESIAN_POINT('Ctrl Pts',(0.235022011279658,0.0320373552576627,
-0.523569105033863));
#72053=CARTESIAN_POINT('Ctrl Pts',(0.235586009968098,0.0274492176768213,
-0.523873405027875));
#72054=CARTESIAN_POINT('Ctrl Pts',(0.235754786569311,0.0259597395952857,
-0.523972512983669));
#72055=CARTESIAN_POINT('Ctrl Pts',(0.236030398466981,0.023302499674537,
-0.524149939243159));
#72056=CARTESIAN_POINT('Ctrl Pts',(0.236142714969529,0.0221353467022232,
-0.524228082607621));
#72057=CARTESIAN_POINT('Ctrl Pts',(0.236361838665955,0.0196664133929033,
-0.524393851976311));
#72058=CARTESIAN_POINT('Ctrl Pts',(0.23646655560621,0.018364491675914,-0.524481540928238));
#72059=CARTESIAN_POINT('Ctrl Pts',(0.236717574604468,0.0148841317712658,
-0.524716722914501));
#72060=CARTESIAN_POINT('Ctrl Pts',(0.236844555280886,0.012704470974011,
-0.524864814833499));
#72061=CARTESIAN_POINT('Ctrl Pts',(0.237345114623906,0.00143407289938757,
-0.52563492584933));
#72062=CARTESIAN_POINT('Ctrl Pts',(0.237225412815,-0.00766982049385359,
-0.526272111051324));
#72063=CARTESIAN_POINT('Ctrl Pts',(0.235818250233654,-0.0275529582367287,
-0.527696140702168));
#72064=CARTESIAN_POINT('Ctrl Pts',(0.234313348873809,-0.038296678014635,
-0.528486886555703));
#72065=CARTESIAN_POINT('Ctrl Pts',(0.229573013052809,-0.0607947583794694,
-0.530166035018932));
#72066=CARTESIAN_POINT('Ctrl Pts',(0.22615542981611,-0.0724813868646703,
-0.531052247248237));
#72067=CARTESIAN_POINT('Ctrl Pts',(0.221123967869649,-0.0857931398776052,
-0.532044922880732));
#72068=CARTESIAN_POINT('Ctrl Pts',(0.220366158560588,-0.0877213138711721,
-0.532188254462476));
#72069=CARTESIAN_POINT('Ctrl Pts',(0.219268250830519,-0.0904107792497356,
-0.532387295237444));
#72070=CARTESIAN_POINT('Ctrl Pts',(0.218949282083269,-0.0911805174071922,
-0.532444159372446));
#72071=CARTESIAN_POINT('Ctrl Pts',(0.218365722168895,-0.0925680486739769,
-0.532546456902546));
#72072=CARTESIAN_POINT('Ctrl Pts',(0.218102549405499,-0.093186427322411,
-0.53259197329234));
#72073=CARTESIAN_POINT('Ctrl Pts',(0.217558037187035,-0.0944509273126081,
-0.53268488358847));
#72074=CARTESIAN_POINT('Ctrl Pts',(0.217276441023691,-0.095096926469615,
-0.532732261556894));
#72075=CARTESIAN_POINT('Ctrl Pts',(0.216542108726632,-0.0967612405080249,
-0.532854121511781));
#72076=CARTESIAN_POINT('Ctrl Pts',(0.216085060948707,-0.097777651195761,
-0.532928346506588));
#72077=CARTESIAN_POINT('Ctrl Pts',(0.214095241944681,-0.102120630047286,
-0.533244816225979));
#72078=CARTESIAN_POINT('Ctrl Pts',(0.212492598056775,-0.105414871175082,
-0.533483139675793));
#72079=CARTESIAN_POINT('Ctrl Pts',(0.20781746220006,-0.114484319665278,
-0.534138067029002));
#72080=CARTESIAN_POINT('Ctrl Pts',(0.204581327868328,-0.120171750972739,
-0.534547411826224));
#72081=CARTESIAN_POINT('Ctrl Pts',(0.199082745057949,-0.128967926221641,
-0.535189638321337));
#72082=CARTESIAN_POINT('Ctrl Pts',(0.196973004602218,-0.132167703478062,
-0.535425278661488));
#72083=CARTESIAN_POINT('Ctrl Pts',(0.18440992919682,-0.150252313283444,
-0.536776473569577));
#72084=CARTESIAN_POINT('Ctrl Pts',(0.17235087217781,-0.163944720201064,
-0.537882550175804));
#72085=CARTESIAN_POINT('Ctrl Pts',(0.156554702582462,-0.178191273166644,
-0.539258278720561));
#72086=CARTESIAN_POINT('Ctrl Pts',(0.154222944574336,-0.180213170068991,
-0.539459575203072));
#72087=CARTESIAN_POINT('Ctrl Pts',(0.150706516611133,-0.1831440745308,-0.539760952344966));
#72088=CARTESIAN_POINT('Ctrl Pts',(0.14955158437768,-0.184088374493874,
-0.539859595955209));
#72089=CARTESIAN_POINT('Ctrl Pts',(0.147473751419888,-0.185754801471623,
-0.540036507088638));
#72090=CARTESIAN_POINT('Ctrl Pts',(0.146554254562996,-0.18648110899634,
-0.540114603543847));
#72091=CARTESIAN_POINT('Ctrl Pts',(0.144595268238482,-0.188005068398782,
-0.540280606967812));
#72092=CARTESIAN_POINT('Ctrl Pts',(0.143554478672965,-0.188800976888037,
-0.540368579372874));
#72093=CARTESIAN_POINT('Ctrl Pts',(0.140746784991828,-0.190911427082562,
-0.540605336787589));
#72094=CARTESIAN_POINT('Ctrl Pts',(0.138968113812755,-0.192210023798749,
-0.54075473481482));
#72095=CARTESIAN_POINT('Ctrl Pts',(0.12950697511722,-0.198917569042661,
-0.541546585609574));
#72096=CARTESIAN_POINT('Ctrl Pts',(0.121527177528542,-0.203890558957619,
-0.542205265320451));
#72097=CARTESIAN_POINT('Ctrl Pts',(0.10393694681623,-0.213452675600637,
-0.543637474943252));
#72098=CARTESIAN_POINT('Ctrl Pts',(0.094269428020421,-0.217894882670642,
-0.544413284230555));
#72099=CARTESIAN_POINT('Ctrl Pts',(0.0731037286647757,-0.225947531162459,
-0.546067082627708));
#72100=CARTESIAN_POINT('Ctrl Pts',(0.0615602883400919,-0.229361789742797,
-0.546942907743081));
#72101=CARTESIAN_POINT('Ctrl Pts',(0.0477724683100303,-0.232323268520589,
-0.547926714424495));
#72102=CARTESIAN_POINT('Ctrl Pts',(0.045732441818632,-0.232733440503412,
-0.548070687355907));
#72103=CARTESIAN_POINT('Ctrl Pts',(0.0428667395150199,-0.233270486902231,
-0.548270466471568));
#72104=CARTESIAN_POINT('Ctrl Pts',(0.0420454607585319,-0.233419914957443,
-0.548327438500273));
#72105=CARTESIAN_POINT('Ctrl Pts',(0.0405611836494176,-0.233681884599432,
-0.548429872392408));
#72106=CARTESIAN_POINT('Ctrl Pts',(0.0398984643800055,-0.233795948188677,
-0.548475417932497));
#72107=CARTESIAN_POINT('Ctrl Pts',(0.0385408714947916,-0.234023668850306,
-0.548568317259998));
#72108=CARTESIAN_POINT('Ctrl Pts',(0.0378459627371746,-0.234137052802743,
-0.548615655594351));
#72109=CARTESIAN_POINT('Ctrl Pts',(0.0360526393801527,-0.234421465614031,
-0.548737292711659));
#72110=CARTESIAN_POINT('Ctrl Pts',(0.034953493370299,-0.234587872170292,
-0.548811336288614));
#72111=CARTESIAN_POINT('Ctrl Pts',(0.0302535385970015,-0.235265660484166,
-0.549125932414795));
#72112=CARTESIAN_POINT('Ctrl Pts',(0.0266421799854468,-0.235701941794512,
-0.549362621017553));
#72113=CARTESIAN_POINT('Ctrl Pts',(0.0165819887027716,-0.236683092486534,
-0.550011566300828));
#72114=CARTESIAN_POINT('Ctrl Pts',(0.010118507675001,-0.237047414070391,
-0.550416723019095));
#72115=CARTESIAN_POINT('Ctrl Pts',(-0.00957069677091684,-0.237350273078646,
-0.551636279247605));
#72116=CARTESIAN_POINT('Ctrl Pts',(-0.0227830231040275,-0.236448076564223,
-0.552435791141741));
#72117=CARTESIAN_POINT('Ctrl Pts',(-0.0459051610031064,-0.23291229393427,
-0.553887449154942));
#72118=CARTESIAN_POINT('Ctrl Pts',(-0.0558483846699635,-0.230730015998957,
-0.554529220835882));
#72119=CARTESIAN_POINT('Ctrl Pts',(-0.0678216978028471,-0.22728274623486,
-0.555340918633542));
#72120=CARTESIAN_POINT('Ctrl Pts',(-0.0700139261114413,-0.226617031526893,
-0.55549114269021));
#72121=CARTESIAN_POINT('Ctrl Pts',(-0.0734749932579312,-0.225510994345337,
-0.555731041137378));
#72122=CARTESIAN_POINT('Ctrl Pts',(-0.0747503648296774,-0.22509146149307,
-0.555820034219674));
#72123=CARTESIAN_POINT('Ctrl Pts',(-0.0771278627139591,-0.224286950524391,
-0.555987075459408));
#72124=CARTESIAN_POINT('Ctrl Pts',(-0.0782308465766714,-0.223904617956588,
-0.556065034150252));
#72125=CARTESIAN_POINT('Ctrl Pts',(-0.0806904646445958,-0.223031636016509,
-0.556239941390695));
#72126=CARTESIAN_POINT('Ctrl Pts',(-0.0820455254802655,-0.222536723570224,
-0.556337029223204));
#72127=CARTESIAN_POINT('Ctrl Pts',(-0.0859849170769581,-0.221057058186752,
-0.556621454261435));
#72128=CARTESIAN_POINT('Ctrl Pts',(-0.0885565659622792,-0.220039456542911,
-0.556809879573585));
#72129=CARTESIAN_POINT('Ctrl Pts',(-0.0944132911535427,-0.21760265114447,
-0.557245527579756));
#72130=CARTESIAN_POINT('Ctrl Pts',(-0.0976851517166901,-0.216153630798189,
-0.557493703058731));
#72131=CARTESIAN_POINT('Ctrl Pts',(-0.108734227334932,-0.210958188725723,
-0.55834848157885));
#72132=CARTESIAN_POINT('Ctrl Pts',(-0.116338508787639,-0.206861824114568,
-0.558965835322636));
#72133=CARTESIAN_POINT('Ctrl Pts',(-0.138958359613599,-0.193034423024834,
-0.560886196524469));
#72134=CARTESIAN_POINT('Ctrl Pts',(-0.153111160632558,-0.182012956809431,
-0.562213018963176));
#72135=CARTESIAN_POINT('Ctrl Pts',(-0.167866838853847,-0.167571916874691,
-0.563663435178786));
#72136=CARTESIAN_POINT('Ctrl Pts',(-0.16980871577917,-0.16560381822515,
-0.56385572847679));
#72137=CARTESIAN_POINT('Ctrl Pts',(-0.172430200082915,-0.162852323353281,
-0.564116745960032));
#72138=CARTESIAN_POINT('Ctrl Pts',(-0.17313965985942,-0.162097845161331,
-0.56418753390917));
#72139=CARTESIAN_POINT('Ctrl Pts',(-0.174265468734213,-0.16088477428329,
-0.564300067336537));
#72140=CARTESIAN_POINT('Ctrl Pts',(-0.174684992697594,-0.160429166731407,
-0.564342047856977));
#72141=CARTESIAN_POINT('Ctrl Pts',(-0.175561550639008,-0.15946970024006,
-0.564429849036139));
#72142=CARTESIAN_POINT('Ctrl Pts',(-0.176018209194962,-0.158965510118756,
-0.564475639678436));
#72143=CARTESIAN_POINT('Ctrl Pts',(-0.177140667371284,-0.157715453158685,
-0.56458833418918));
#72144=CARTESIAN_POINT('Ctrl Pts',(-0.177803942013721,-0.156967316647778,
-0.564655051727945));
#72145=CARTESIAN_POINT('Ctrl Pts',(-0.18020055206605,-0.154229391363479,
-0.564896677840784));
#72146=CARTESIAN_POINT('Ctrl Pts',(-0.181905453860643,-0.152214819940171,
-0.565069637428765));
#72147=CARTESIAN_POINT('Ctrl Pts',(-0.18997951233834,-0.142344764301913,
-0.565896395197436));
#72148=CARTESIAN_POINT('Ctrl Pts',(-0.195876118778367,-0.134115015891556,
-0.566524180511667));
#72149=CARTESIAN_POINT('Ctrl Pts',(-0.206845864889663,-0.116530495209853,
-0.567799129845046));
#72150=CARTESIAN_POINT('Ctrl Pts',(-0.21185140795199,-0.107161308260448,
-0.568444489340571));
#72151=CARTESIAN_POINT('Ctrl Pts',(-0.220469427169856,-0.0880480228350329,
-0.569744813863598));
#72152=CARTESIAN_POINT('Ctrl Pts',(-0.224102724212719,-0.0783399758487367,
-0.57039779297285));
#72153=CARTESIAN_POINT('Ctrl Pts',(-0.227753542249212,-0.0662238350929426,
-0.571222082154118));
#72154=CARTESIAN_POINT('Ctrl Pts',(-0.228385114451004,-0.0640118053968531,
-0.571372907803587));
#72155=CARTESIAN_POINT('Ctrl Pts',(-0.229334731862316,-0.0604927239157919,
-0.571613551645852));
#72156=CARTESIAN_POINT('Ctrl Pts',(-0.229674015584425,-0.0591915139546034,
-0.571702681224881));
#72157=CARTESIAN_POINT('Ctrl Pts',(-0.230287086205016,-0.0567556241761504,
-0.571869845054797));
#72158=CARTESIAN_POINT('Ctrl Pts',(-0.230563598619468,-0.0556216671463706,
-0.571947788629566));
#72159=CARTESIAN_POINT('Ctrl Pts',(-0.231089283680852,-0.0533945742143698,
-0.572101134728435));
#72160=CARTESIAN_POINT('Ctrl Pts',(-0.231339097560891,-0.0523016199777244,
-0.572176514314871));
#72161=CARTESIAN_POINT('Ctrl Pts',(-0.231885217019687,-0.0498318191477032,
-0.572347150390873));
#72162=CARTESIAN_POINT('Ctrl Pts',(-0.232177024488392,-0.0484540320528138,
-0.572442547989112));
#72163=CARTESIAN_POINT('Ctrl Pts',(-0.232885067724556,-0.0449576191226075,
-0.572685194325873));
#72164=CARTESIAN_POINT('Ctrl Pts',(-0.233284668193528,-0.0428357950472687,
-0.572832961562156));
#72165=CARTESIAN_POINT('Ctrl Pts',(-0.236010352359248,-0.027191284116254,
-0.57392646661218));
#72166=CARTESIAN_POINT('Ctrl Pts',(-0.237187548041389,-0.0134974807389825,
-0.574907807761886));
#72167=CARTESIAN_POINT('Ctrl Pts',(-0.237174899149993,0.00021871943419613,
-0.575905717570473));
#72168=CARTESIAN_POINT('Ctrl Pts',(-0.0419766262164012,0.23365534329502,
-0.598123480850464));
#72169=CARTESIAN_POINT('Ctrl Pts',(-0.0526520230118338,0.231835363692615,
-0.597394838096837));
#72170=CARTESIAN_POINT('Ctrl Pts',(-0.139695025652084,0.210579474520431,
-0.591371551985214));
#72171=CARTESIAN_POINT('Ctrl Pts',(-0.225519033105649,0.119811949965669,
-0.583977407967588));
#72172=CARTESIAN_POINT('Ctrl Pts',(-0.237296177544911,0.0206528429717354,
-0.57731190670359));
#72173=CARTESIAN_POINT('Ctrl Pts',(-0.237113469260214,0.000216662027683377,
-0.575941048797587));
#72174=CARTESIAN_POINT('',(-0.237522045222027,-7.70250957813517E-5,-0.595652851074302));
#72175=CARTESIAN_POINT('Ctrl Pts',(-0.0418741542966648,0.233068851607476,
-0.617833934840082));
#72176=CARTESIAN_POINT('Ctrl Pts',(-0.0770653683707668,0.226841574278908,
-0.615444604463725));
#72177=CARTESIAN_POINT('Ctrl Pts',(-0.181642156144958,0.184255516872655,
-0.608052990951751));
#72178=CARTESIAN_POINT('Ctrl Pts',(-0.237210808141337,0.0741535263668472,
-0.60066137743978));
#72179=CARTESIAN_POINT('Ctrl Pts',(-0.237532922930967,-7.74222378633504E-5,
-0.595659094304164));
#72180=CARTESIAN_POINT('Ctrl Pts',(-0.237174991269168,-6.43542539559139E-5,
-0.595453660452978));
#72181=CARTESIAN_POINT('Ctrl Pts',(-0.237174364967726,-0.00237256280265978,
-0.595291666791208));
#72182=CARTESIAN_POINT('Ctrl Pts',(-0.237140043091288,-0.00468075615503481,
-0.59513102131791));
#72183=CARTESIAN_POINT('Ctrl Pts',(-0.237046058216446,-0.0078691605257938,
-0.594911300655702));
#72184=CARTESIAN_POINT('Ctrl Pts',(-0.237015178994657,-0.0087499936839357,
-0.594850831062905));
#72185=CARTESIAN_POINT('Ctrl Pts',(-0.236952705462167,-0.0102872666538859,
-0.59474572287562));
#72186=CARTESIAN_POINT('Ctrl Pts',(-0.236923291848027,-0.0109437784665437,
-0.594700970890158));
#72187=CARTESIAN_POINT('Ctrl Pts',(-0.236860251490791,-0.0122311478259143,
-0.594613493078634));
#72188=CARTESIAN_POINT('Ctrl Pts',(-0.236826832148373,-0.0128620110159745,
-0.594570756598602));
#72189=CARTESIAN_POINT('Ctrl Pts',(-0.23674925025568,-0.0142235333722509,
-0.594478813958949));
#72190=CARTESIAN_POINT('Ctrl Pts',(-0.236704225687466,-0.0149541290827802,
-0.594429656067645));
#72191=CARTESIAN_POINT('Ctrl Pts',(-0.236573901414612,-0.0169205267247753,
-0.594297800630824));
#72192=CARTESIAN_POINT('Ctrl Pts',(-0.236482299953095,-0.0181559089434672,
-0.594215444896435));
#72193=CARTESIAN_POINT('Ctrl Pts',(-0.236015912577266,-0.0238414168202966,
-0.59383841107224));
#72194=CARTESIAN_POINT('Ctrl Pts',(-0.23552513848384,-0.0282814329169275,
-0.593549575711258));
#72195=CARTESIAN_POINT('Ctrl Pts',(-0.232875735959759,-0.0473110602734093,
-0.59232562791775));
#72196=CARTESIAN_POINT('Ctrl Pts',(-0.229484309769027,-0.0616966295445551,
-0.591434318300533));
#72197=CARTESIAN_POINT('Ctrl Pts',(-0.220737362157619,-0.0876777794383515,
-0.589749526966357));
#72198=CARTESIAN_POINT('Ctrl Pts',(-0.21574207370356,-0.0993361845106995,
-0.588962803570763));
#72199=CARTESIAN_POINT('Ctrl Pts',(-0.208372266667843,-0.113326533785409,
-0.587940689071195));
#72200=CARTESIAN_POINT('Ctrl Pts',(-0.206848709372263,-0.116084084546745,
-0.587735290429501));
#72201=CARTESIAN_POINT('Ctrl Pts',(-0.204517489273079,-0.120111773947784,
-0.587428973656753));
#72202=CARTESIAN_POINT('Ctrl Pts',(-0.203751895292275,-0.12140595804614,
-0.587329564014937));
#72203=CARTESIAN_POINT('Ctrl Pts',(-0.202367393829763,-0.123696377689382,
-0.587151824987848));
#72204=CARTESIAN_POINT('Ctrl Pts',(-0.201753300158513,-0.124695475977623,
-0.587073673219476));
#72205=CARTESIAN_POINT('Ctrl Pts',(-0.200441425995232,-0.126794765732958,
-0.586908123675633));
#72206=CARTESIAN_POINT('Ctrl Pts',(-0.199741941561339,-0.127893840883713,
-0.586820664759316));
#72207=CARTESIAN_POINT('Ctrl Pts',(-0.197853713350675,-0.130807470514853,
-0.586586674194169));
#72208=CARTESIAN_POINT('Ctrl Pts',(-0.196649093645901,-0.132611536646144,
-0.586439553943037));
#72209=CARTESIAN_POINT('Ctrl Pts',(-0.190966132320522,-0.14087473634893,
-0.585755062407461));
#72210=CARTESIAN_POINT('Ctrl Pts',(-0.186193677998158,-0.147124589577071,
-0.585206631042645));
#72211=CARTESIAN_POINT('Ctrl Pts',(-0.17114287346141,-0.164927022395434,
-0.583549892348229));
#72212=CARTESIAN_POINT('Ctrl Pts',(-0.160036533161969,-0.175724292345416,
-0.582414087636772));
#72213=CARTESIAN_POINT('Ctrl Pts',(-0.142709880293066,-0.189554765978345,
-0.580801134905494));
#72214=CARTESIAN_POINT('Ctrl Pts',(-0.137282941452883,-0.193521382241397,
-0.58031576124169));
#72215=CARTESIAN_POINT('Ctrl Pts',(-0.129609936051608,-0.198644224259631,
-0.579662659841458));
#72216=CARTESIAN_POINT('Ctrl Pts',(-0.127503286264467,-0.20000294111581,
-0.579486622933222));
#72217=CARTESIAN_POINT('Ctrl Pts',(-0.124283778770851,-0.202007863038646,
-0.579222939517429));
#72218=CARTESIAN_POINT('Ctrl Pts',(-0.123186615034183,-0.202678791308846,
-0.579134000849986));
#72219=CARTESIAN_POINT('Ctrl Pts',(-0.121160912232504,-0.203895005494751,
-0.578971551820555));
#72220=CARTESIAN_POINT('Ctrl Pts',(-0.120234018939932,-0.204442952238364,
-0.578897888497295));
#72221=CARTESIAN_POINT('Ctrl Pts',(-0.118706689585987,-0.20533187564164,
-0.578777638569231));
#72222=CARTESIAN_POINT('Ctrl Pts',(-0.118108451580459,-0.205676568921734,
-0.578730820474705));
#72223=CARTESIAN_POINT('Ctrl Pts',(-0.11692522724356,-0.206351455208957,
-0.578638790191275));
#72224=CARTESIAN_POINT('Ctrl Pts',(-0.116340331267228,-0.206681782386678,
-0.578593570604684));
#72225=CARTESIAN_POINT('Ctrl Pts',(-0.115027364560979,-0.207415956911952,
-0.5784926549391));
#72226=CARTESIAN_POINT('Ctrl Pts',(-0.114298547382574,-0.207818468615713,
-0.578437042915983));
#72227=CARTESIAN_POINT('Ctrl Pts',(-0.111751363888757,-0.209207775685885,
-0.578244036259951));
#72228=CARTESIAN_POINT('Ctrl Pts',(-0.1099221556088,-0.210174644424576,
-0.578107825966146));
#72229=CARTESIAN_POINT('Ctrl Pts',(-0.0972579440298088,-0.216658018774652,
-0.577179510633432));
#72230=CARTESIAN_POINT('Ctrl Pts',(-0.0860239447449395,-0.221358898838197,
-0.576428885493879));
#72231=CARTESIAN_POINT('Ctrl Pts',(-0.0641930178298191,-0.228579488531291,
-0.575017512308011));
#72232=CARTESIAN_POINT('Ctrl Pts',(-0.0536875482153833,-0.231272487607986,
-0.574357478384001));
#72233=CARTESIAN_POINT('Ctrl Pts',(-0.0340823292735756,-0.234889885050145,
-0.573114415965014));
#72234=CARTESIAN_POINT('Ctrl Pts',(-0.0250427285420628,-0.2360247780673,
-0.572537068560617));
#72235=CARTESIAN_POINT('Ctrl Pts',(-0.0137826979678303,-0.236784256940236,
-0.571800795587073));
#72236=CARTESIAN_POINT('Ctrl Pts',(-0.0116025592820808,-0.236901091583059,
-0.571657473194882));
#72237=CARTESIAN_POINT('Ctrl Pts',(-0.00811638441949301,-0.237039680438405,
-0.57142692553729));
#72238=CARTESIAN_POINT('Ctrl Pts',(-0.00681120873066814,-0.237080773404782,
-0.571340306293188));
#72239=CARTESIAN_POINT('Ctrl Pts',(-0.00433398712852715,-0.237138295145103,
-0.571175293579186));
#72240=CARTESIAN_POINT('Ctrl Pts',(-0.0031620251166205,-0.237156817276737,
-0.571096968108943));
#72241=CARTESIAN_POINT('Ctrl Pts',(-0.000491829408069863,-0.237179222061253,
-0.570917899582971));
#72242=CARTESIAN_POINT('Ctrl Pts',(0.00100638775418432,-0.237177596492656,
-0.570816987236155));
#72243=CARTESIAN_POINT('Ctrl Pts',(0.00562563048261394,-0.23712881668216,
-0.570504452008143));
#72244=CARTESIAN_POINT('Ctrl Pts',(0.00874570960937807,-0.23703424723826,
-0.570291364391872));
#72245=CARTESIAN_POINT('Ctrl Pts',(0.0295370486453282,-0.235993014212989,
-0.568857507091995));
#72246=CARTESIAN_POINT('Ctrl Pts',(0.0470534520428524,-0.23313276472498,
-0.56757621241717));
#72247=CARTESIAN_POINT('Ctrl Pts',(0.0682747558833584,-0.227177181415122,
-0.56596639182474));
#72248=CARTESIAN_POINT('Ctrl Pts',(0.0724310583169615,-0.225886380055069,
-0.565648588912877));
#72249=CARTESIAN_POINT('Ctrl Pts',(0.0826869346882144,-0.222389071818803,
-0.564860800502041));
#72250=CARTESIAN_POINT('Ctrl Pts',(0.088736352147564,-0.22004522166057,
-0.564392851018951));
#72251=CARTESIAN_POINT('Ctrl Pts',(0.0980214519375577,-0.216002402829693,
-0.563676433286827));
#72252=CARTESIAN_POINT('Ctrl Pts',(0.10132674335912,-0.214471764436723,
-0.563421798239548));
#72253=CARTESIAN_POINT('Ctrl Pts',(0.105593635895879,-0.21237514225777,
-0.563094790851715));
#72254=CARTESIAN_POINT('Ctrl Pts',(0.106588152603565,-0.21187775446711,
-0.563018696561857));
#72255=CARTESIAN_POINT('Ctrl Pts',(0.108206562668344,-0.21105405947461,
-0.562895112779373));
#72256=CARTESIAN_POINT('Ctrl Pts',(0.108832552105023,-0.210731943142361,
-0.562847372297404));
#72257=CARTESIAN_POINT('Ctrl Pts',(0.110053363718528,-0.210096857406963,
-0.562754401041409));
#72258=CARTESIAN_POINT('Ctrl Pts',(0.110648302977808,-0.209784140066978,
-0.562709156252696));
#72259=CARTESIAN_POINT('Ctrl Pts',(0.111978512731564,-0.20907771023795,
-0.562608118283999));
#72260=CARTESIAN_POINT('Ctrl Pts',(0.112713059494938,-0.208682635845613,
-0.562552409826735));
#72261=CARTESIAN_POINT('Ctrl Pts',(0.115269921669376,-0.207289994087695,
-0.562358739375872));
#72262=CARTESIAN_POINT('Ctrl Pts',(0.117081264603381,-0.206272331378097,
-0.56222197242369));
#72263=CARTESIAN_POINT('Ctrl Pts',(0.12930782146226,-0.199190155230564,
-0.561300133642804));
#72264=CARTESIAN_POINT('Ctrl Pts',(0.139262362439573,-0.192362417569494,
-0.560555750398351));
#72265=CARTESIAN_POINT('Ctrl Pts',(0.156976219061154,-0.178113655481915,
-0.559160198717179));
#72266=CARTESIAN_POINT('Ctrl Pts',(0.164835156615894,-0.170866526968388,
-0.558509614241831));
#72267=CARTESIAN_POINT('Ctrl Pts',(0.178592068984296,-0.156345167960695,
-0.557263537882503));
#72268=CARTESIAN_POINT('Ctrl Pts',(0.184599822741478,-0.149203931271848,
-0.556672697092615));
#72269=CARTESIAN_POINT('Ctrl Pts',(0.191484311341427,-0.139966308808759,
-0.555921193740991));
#72270=CARTESIAN_POINT('Ctrl Pts',(0.192772807237123,-0.138186299424059,
-0.555776959208841));
#72271=CARTESIAN_POINT('Ctrl Pts',(0.194789037651535,-0.135317865206395,
-0.555545290683498));
#72272=CARTESIAN_POINT('Ctrl Pts',(0.195532834493481,-0.134240844572613,
-0.55545847331205));
#72273=CARTESIAN_POINT('Ctrl Pts',(0.1969253908652,-0.132188288050696,-0.555293305184091));
#72274=CARTESIAN_POINT('Ctrl Pts',(0.197575913415688,-0.131213990939206,
-0.555215024294645));
#72275=CARTESIAN_POINT('Ctrl Pts',(0.199038908679309,-0.128987293962221,
-0.555036367636241));
#72276=CARTESIAN_POINT('Ctrl Pts',(0.199846821728958,-0.127731972658824,
-0.554935825468488));
#72277=CARTESIAN_POINT('Ctrl Pts',(0.202292085954818,-0.123852569943335,
-0.554625601978909));
#72278=CARTESIAN_POINT('Ctrl Pts',(0.203889944341918,-0.121204109427891,
-0.554414487113187));
#72279=CARTESIAN_POINT('Ctrl Pts',(0.214480468748191,-0.102847942259788,
-0.552955172454069));
#72280=CARTESIAN_POINT('Ctrl Pts',(0.221699529875901,-0.0861896030936155,
-0.551643272546658));
#72281=CARTESIAN_POINT('Ctrl Pts',(0.228091379389882,-0.0651279471798013,
-0.55003573205021));
#72282=CARTESIAN_POINT('Ctrl Pts',(0.229135979823658,-0.0613516934154544,
-0.549749713353507));
#72283=CARTESIAN_POINT('Ctrl Pts',(0.231672747531028,-0.0512098446968167,
-0.548989532873781));
#72284=CARTESIAN_POINT('Ctrl Pts',(0.232996187252141,-0.0448051156460757,
-0.548517688347433));
#72285=CARTESIAN_POINT('Ctrl Pts',(0.234645422208803,-0.0347406092982293,
-0.547796092467409));
#72286=CARTESIAN_POINT('Ctrl Pts',(0.235153761598731,-0.031114243509007,
-0.547540077025534));
#72287=CARTESIAN_POINT('Ctrl Pts',(0.235707023331009,-0.0263708316703005,
-0.547211585599379));
#72288=CARTESIAN_POINT('Ctrl Pts',(0.235828288448366,-0.0252634142876844,
-0.547135346919539));
#72289=CARTESIAN_POINT('Ctrl Pts',(0.236013493612088,-0.0234543748584933,
-0.547011588205249));
#72290=CARTESIAN_POINT('Ctrl Pts',(0.236082116669978,-0.0227532654514893,
-0.546963815873332));
#72291=CARTESIAN_POINT('Ctrl Pts',(0.236210078324722,-0.0213829567942696,
-0.546870833003076));
#72292=CARTESIAN_POINT('Ctrl Pts',(0.236269698846107,-0.0207137965562993,
-0.546825608107873));
#72293=CARTESIAN_POINT('Ctrl Pts',(0.236396864353383,-0.0192144950637545,
-0.546724666644068));
#72294=CARTESIAN_POINT('Ctrl Pts',(0.236462882146181,-0.0183842246462954,
-0.546669034272001));
#72295=CARTESIAN_POINT('Ctrl Pts',(0.236677778227756,-0.0154886265795101,
-0.546475887705503));
#72296=CARTESIAN_POINT('Ctrl Pts',(0.236803987621979,-0.0134216400827039,
-0.546339560101602));
#72297=CARTESIAN_POINT('Ctrl Pts',(0.237485492057007,0.000799090680145227,
-0.545410630885345));
#72298=CARTESIAN_POINT('Ctrl Pts',(0.23713202746367,0.0129798120500622,
-0.544659554214914));
#72299=CARTESIAN_POINT('Ctrl Pts',(0.234697959336753,0.0358682352331096,
-0.543246762281554));
#72300=CARTESIAN_POINT('Ctrl Pts',(0.232812051046232,0.0465639499299556,
-0.542585776208153));
#72301=CARTESIAN_POINT('Ctrl Pts',(0.228014886848421,0.0659063916198067,
-0.541343071473364));
#72302=CARTESIAN_POINT('Ctrl Pts',(0.225324834881934,0.0745863989112967,
-0.540767142030793));
#72303=CARTESIAN_POINT('Ctrl Pts',(0.221379776316486,0.0851336309306886,
-0.540032470055647));
#72304=CARTESIAN_POINT('Ctrl Pts',(0.220587314807362,0.0871663725392257,
-0.539889245432231));
#72305=CARTESIAN_POINT('Ctrl Pts',(0.219276024223611,0.0903975117953189,
-0.539658817914129));
#72306=CARTESIAN_POINT('Ctrl Pts',(0.218775132656203,0.0916030903061705,
-0.539572219909044));
#72307=CARTESIAN_POINT('Ctrl Pts',(0.217805659725784,0.0938831679032894,
-0.539407223712777));
#72308=CARTESIAN_POINT('Ctrl Pts',(0.217339013978693,0.0949584516607608,
-0.539328893320299));
#72309=CARTESIAN_POINT('Ctrl Pts',(0.216257571748591,0.0974006657528809,
-0.539149779944029));
#72310=CARTESIAN_POINT('Ctrl Pts',(0.215637755235712,0.098765304459563,
-0.539048827354598));
#72311=CARTESIAN_POINT('Ctrl Pts',(0.213686070078126,0.102956331492917,
-0.53873604017328));
#72312=CARTESIAN_POINT('Ctrl Pts',(0.212311299652096,0.105762248255869,
-0.538522737426246));
#72313=CARTESIAN_POINT('Ctrl Pts',(0.202805864629077,0.124230274180054,
-0.537092059582729));
#72314=CARTESIAN_POINT('Ctrl Pts',(0.193005765026251,0.138967368594582,
-0.53581454406287));
#72315=CARTESIAN_POINT('Ctrl Pts',(0.178826985613105,0.155860119530935,
-0.534203750671509));
#72316=CARTESIAN_POINT('Ctrl Pts',(0.17589509967971,0.159161497979249,-0.533881320985099));
#72317=CARTESIAN_POINT('Ctrl Pts',(0.168441890771932,0.167096363333458,
-0.533089889086122));
#72318=CARTESIAN_POINT('Ctrl Pts',(0.163819491191561,0.17163056488607,-0.532622876747621));
#72319=CARTESIAN_POINT('Ctrl Pts',(0.156318594807358,0.178408817208816,
-0.531907705975132));
#72320=CARTESIAN_POINT('Ctrl Pts',(0.153564149282636,0.180785134275456,
-0.531653404069181));
#72321=CARTESIAN_POINT('Ctrl Pts',(0.149897948038343,0.183803756890842,
-0.531326754984067));
#72322=CARTESIAN_POINT('Ctrl Pts',(0.14903496577768,0.184504186867197,-0.531250695658668));
#72323=CARTESIAN_POINT('Ctrl Pts',(0.147617445664233,0.185638266005345,
-0.531127154235261));
#72324=CARTESIAN_POINT('Ctrl Pts',(0.147065856878645,0.186075548752318,
-0.531079421464324));
#72325=CARTESIAN_POINT('Ctrl Pts',(0.145983724702753,0.186925612426653,
-0.530986452984858));
#72326=CARTESIAN_POINT('Ctrl Pts',(0.145453361590474,0.187338602745772,
-0.53094120334465));
#72327=CARTESIAN_POINT('Ctrl Pts',(0.144260796322612,0.188259128192028,
-0.530840141881582));
#72328=CARTESIAN_POINT('Ctrl Pts',(0.143597650706156,0.188765440341301,
-0.530784414909541));
#72329=CARTESIAN_POINT('Ctrl Pts',(0.141272670167787,0.190521222044709,
-0.530590616793896));
#72330=CARTESIAN_POINT('Ctrl Pts',(0.139597031901368,0.191752373634479,
-0.53045374275603));
#72331=CARTESIAN_POINT('Ctrl Pts',(0.128117934878563,0.199956237479907,
-0.529533246987873));
#72332=CARTESIAN_POINT('Ctrl Pts',(0.117811186178973,0.206197237749492,
-0.528790152173273));
#72333=CARTESIAN_POINT('Ctrl Pts',(0.0975772066812585,0.216434628539015,
-0.527398064029015));
#72334=CARTESIAN_POINT('Ctrl Pts',(0.0877677526280537,0.220594815865414,
-0.526749624709212));
#72335=CARTESIAN_POINT('Ctrl Pts',(0.0688559372362668,0.227153497815084,
-0.525502942794627));
#72336=CARTESIAN_POINT('Ctrl Pts',(0.0598261243365684,0.229696876582851,
-0.52490912582114));
#72337=CARTESIAN_POINT('Ctrl Pts',(0.0485206003293139,0.232169278467857,
-0.524154264256176));
#72338=CARTESIAN_POINT('Ctrl Pts',(0.0463645962284942,0.232609428446374,
-0.524009832921641));
#72339=CARTESIAN_POINT('Ctrl Pts',(0.0429162240681387,0.233263570410312,
-0.523777922555877));
#72340=CARTESIAN_POINT('Ctrl Pts',(0.0416276330411383,0.233496971328214,
-0.523691062443543));
#72341=CARTESIAN_POINT('Ctrl Pts',(0.0391828750733199,0.233918907047026,
-0.523525860479693));
#72342=CARTESIAN_POINT('Ctrl Pts',(0.0380271115126804,0.234109571521905,
-0.523447588896423));
#72343=CARTESIAN_POINT('Ctrl Pts',(0.0353964468609779,0.234523553845564,
-0.523269019571817));
#72344=CARTESIAN_POINT('Ctrl Pts',(0.0339207683405629,0.234741532449766,
-0.523168556045875));
#72345=CARTESIAN_POINT('Ctrl Pts',(0.0293852098264478,0.235367838586018,
-0.522858822306003));
#72346=CARTESIAN_POINT('Ctrl Pts',(0.0263194391213415,0.235730345002672,
-0.522648125112458));
#72347=CARTESIAN_POINT('Ctrl Pts',(0.00515981982593997,0.237814419393502,
-0.521184077497259));
#72348=CARTESIAN_POINT('Ctrl Pts',(-0.0130695234560479,0.237510557714901,
-0.51986641709386));
#72349=CARTESIAN_POINT('Ctrl Pts',(-0.0347144503614342,0.234649349495437,
-0.518271817473785));
#72350=CARTESIAN_POINT('Ctrl Pts',(-0.0383347093569048,0.234085119227144,
-0.518004355068976));
#72351=CARTESIAN_POINT('Ctrl Pts',(-0.0419392867764624,0.233437522368795,
-0.517737946518584));
#72352=CARTESIAN_POINT('Origin',(0.,0.,-2.1456589891905));
#72353=CARTESIAN_POINT('',(-0.0419392740612461,0.233437524653205,-0.397890210729054));
#72354=CARTESIAN_POINT('',(-0.041939274266712,0.233437524616291,-0.417694787181515));
#72355=CARTESIAN_POINT('',(-0.0419392741328076,0.233437524640348,-2.1456589891905));
#72356=CARTESIAN_POINT('Ctrl Pts',(-0.0419392740612461,0.233437524653205,
-0.397890210729054));
#72357=CARTESIAN_POINT('Ctrl Pts',(-0.0402008843706342,0.233749842913811,
-0.398010601581905));
#72358=CARTESIAN_POINT('Ctrl Pts',(-0.0384590613533141,0.234042732781722,
-0.398131602917604));
#72359=CARTESIAN_POINT('Ctrl Pts',(-0.0186066639421137,0.237153331412323,
-0.39951511916644));
#72360=CARTESIAN_POINT('Ctrl Pts',(-0.000234620402447351,0.237881494207574,
-0.400844414765493));
#72361=CARTESIAN_POINT('Ctrl Pts',(0.0217149774632429,0.236207682940379,
-0.402452128909572));
#72362=CARTESIAN_POINT('Ctrl Pts',(0.0253890361293069,0.235841063358142,
-0.402721619783982));
#72363=CARTESIAN_POINT('Ctrl Pts',(0.0355580255649566,0.23458594681924,
-0.403466707445045));
#72364=CARTESIAN_POINT('Ctrl Pts',(0.0420273580620156,0.233513709194453,
-0.403939857560636));
#72365=CARTESIAN_POINT('Ctrl Pts',(0.0520347969310622,0.231425610210343,
-0.404663206288373));
#72366=CARTESIAN_POINT('Ctrl Pts',(0.0556076302153558,0.230593209523418,
-0.404919700847363));
#72367=CARTESIAN_POINT('Ctrl Pts',(0.0602396563793955,0.229400103609189,
-0.405248723717678));
#72368=CARTESIAN_POINT('Ctrl Pts',(0.0613174160332498,0.229114378316452,
-0.405325028635298));
#72369=CARTESIAN_POINT('Ctrl Pts',(0.0630731333764691,0.228635642957073,
-0.405448878267782));
#72370=CARTESIAN_POINT('Ctrl Pts',(0.0637523010832571,0.228447196358497,
-0.405496675809539));
#72371=CARTESIAN_POINT('Ctrl Pts',(0.0650773210398278,0.228073177824649,
-0.405589694652314));
#72372=CARTESIAN_POINT('Ctrl Pts',(0.0657232388445533,0.227887884824202,
-0.405634930408187));
#72373=CARTESIAN_POINT('Ctrl Pts',(0.0671679766557816,0.227466782698395,
-0.405735883728774));
#72374=CARTESIAN_POINT('Ctrl Pts',(0.0679663677772369,0.227229503415424,
-0.405791517163645));
#72375=CARTESIAN_POINT('Ctrl Pts',(0.070744392289104,0.226387931645108,
-0.405984606915277));
#72376=CARTESIAN_POINT('Ctrl Pts',(0.0727174200606783,0.225761914790316,
-0.40612087782565));
#72377=CARTESIAN_POINT('Ctrl Pts',(0.086258118429489,0.221269679973657,
-0.407051732514566));
#72378=CARTESIAN_POINT('Ctrl Pts',(0.097522249466343,0.216541502009419,
-0.407804574319244));
#72379=CARTESIAN_POINT('Ctrl Pts',(0.116166878108451,0.206963754168709,
-0.409091080310384));
#72380=CARTESIAN_POINT('Ctrl Pts',(0.123732078996018,0.202531745948396,
-0.409625618141897));
#72381=CARTESIAN_POINT('Ctrl Pts',(0.13939916052274,0.192147233529331,-0.410789473634976));
#72382=CARTESIAN_POINT('Ctrl Pts',(0.147402540302711,0.186078321364228,
-0.411420256346053));
#72383=CARTESIAN_POINT('Ctrl Pts',(0.157127667175876,0.177681739833076,
-0.412253228564104));
#72384=CARTESIAN_POINT('Ctrl Pts',(0.159225334355741,0.175804426178106,
-0.412437159364938));
#72385=CARTESIAN_POINT('Ctrl Pts',(0.162343934824314,0.172911820551287,
-0.412717458118383));
#72386=CARTESIAN_POINT('Ctrl Pts',(0.16338990116483,0.171923793885699,-0.412812672211412));
#72387=CARTESIAN_POINT('Ctrl Pts',(0.165267913119384,0.170117194016267,
-0.412985864782996));
#72388=CARTESIAN_POINT('Ctrl Pts',(0.166103035186032,0.169301873660903,
-0.41306370075071));
#72389=CARTESIAN_POINT('Ctrl Pts',(0.167887839869451,0.167533471406042,
-0.413231849910912));
#72390=CARTESIAN_POINT('Ctrl Pts',(0.168835494180268,0.166578409743422,
-0.413322249113473));
#72391=CARTESIAN_POINT('Ctrl Pts',(0.171383487121962,0.163966421324328,
-0.41356840591792));
#72392=CARTESIAN_POINT('Ctrl Pts',(0.172967859910619,0.16229419510503,-0.413724847319821));
#72393=CARTESIAN_POINT('Ctrl Pts',(0.181583586867232,0.152931247570632,
-0.414594776761866));
#72394=CARTESIAN_POINT('Ctrl Pts',(0.188125582841696,0.1448077200227,-0.415328368871273));
#72395=CARTESIAN_POINT('Ctrl Pts',(0.203644990521002,0.122702748566535,
-0.417269428085389));
#72396=CARTESIAN_POINT('Ctrl Pts',(0.211726561384617,0.10816221640806,-0.418497393025293));
#72397=CARTESIAN_POINT('Ctrl Pts',(0.220612248233739,0.0872890464152246,
-0.420126884760523));
#72398=CARTESIAN_POINT('Ctrl Pts',(0.222783065238373,0.0815895945170851,
-0.420558761122068));
#72399=CARTESIAN_POINT('Ctrl Pts',(0.225150298159732,0.0745723561417519,
-0.42106987370135));
#72400=CARTESIAN_POINT('Ctrl Pts',(0.225558331637648,0.0733289321285298,
-0.421159667051202));
#72401=CARTESIAN_POINT('Ctrl Pts',(0.226183230348393,0.0713700611089194,
-0.421299845011767));
#72402=CARTESIAN_POINT('Ctrl Pts',(0.226407033041811,0.0706568803577203,
-0.421350615350519));
#72403=CARTESIAN_POINT('Ctrl Pts',(0.226822487521583,0.069310728799461,
-0.421445931070812));
#72404=CARTESIAN_POINT('Ctrl Pts',(0.22701486249877,0.068678018234242,-0.421490515325779));
#72405=CARTESIAN_POINT('Ctrl Pts',(0.227455498332989,0.0672067089610365,
-0.421593703890249));
#72406=CARTESIAN_POINT('Ctrl Pts',(0.227701770405727,0.0663675317168976,
-0.421652193003436));
#72407=CARTESIAN_POINT('Ctrl Pts',(0.228494851880888,0.0636087040252514,
-0.421843339050414));
#72408=CARTESIAN_POINT('Ctrl Pts',(0.229022088873881,0.06168345013147,-0.421974925963065));
#72409=CARTESIAN_POINT('Ctrl Pts',(0.233456489299866,0.0446495281187777,
-0.423125177904624));
#72410=CARTESIAN_POINT('Ctrl Pts',(0.235888469034036,0.0291939203176684,
-0.424073933576794));
#72411=CARTESIAN_POINT('Ctrl Pts',(0.237589924520497,-0.000408606105287425,
-0.425891524116123));
#72412=CARTESIAN_POINT('Ctrl Pts',(0.23714916268035,-0.0144690854275087,
-0.426755543941157));
#72413=CARTESIAN_POINT('Ctrl Pts',(0.235008687643185,-0.0322114963700264,
-0.427904329174176));
#72414=CARTESIAN_POINT('Ctrl Pts',(0.234457629580041,-0.036003902824007,
-0.428153179623342));
#72415=CARTESIAN_POINT('Ctrl Pts',(0.233542553792801,-0.0413822923748594,
-0.428511606046887));
#72416=CARTESIAN_POINT('Ctrl Pts',(0.23325369924883,-0.0429805784204745,
-0.428618814649973));
#72417=CARTESIAN_POINT('Ctrl Pts',(0.23272466247339,-0.0457452729318386,
-0.428805528409901));
#72418=CARTESIAN_POINT('Ctrl Pts',(0.232492066046093,-0.0469130861917967,
-0.428884789944866));
#72419=CARTESIAN_POINT('Ctrl Pts',(0.231996920755761,-0.0493049338275856,
-0.429047959753064));
#72420=CARTESIAN_POINT('Ctrl Pts',(0.231733455230604,-0.0505287379874477,
-0.429131895060779));
#72421=CARTESIAN_POINT('Ctrl Pts',(0.231038654738067,-0.0536363237877092,
-0.429346201667886));
#72422=CARTESIAN_POINT('Ctrl Pts',(0.230593968257228,-0.0555169940670322,
-0.429476996867895));
#72423=CARTESIAN_POINT('Ctrl Pts',(0.228768197821384,-0.062837842015074,
-0.429990571060034));
#72424=CARTESIAN_POINT('Ctrl Pts',(0.227217260567347,-0.0682333499428704,
-0.430378738217138));
#72425=CARTESIAN_POINT('Ctrl Pts',(0.220121007886839,-0.089982339936886,
-0.431984167073725));
#72426=CARTESIAN_POINT('Ctrl Pts',(0.212989736483191,-0.105760534315724,
-0.43324960033746));
#72427=CARTESIAN_POINT('Ctrl Pts',(0.200469044737067,-0.126957803020404,
-0.435043658018043));
#72428=CARTESIAN_POINT('Ctrl Pts',(0.19643382964896,-0.133116064449294,
-0.435576726327406));
#72429=CARTESIAN_POINT('Ctrl Pts',(0.189800908020513,-0.142278661390064,
-0.43637880373576));
#72430=CARTESIAN_POINT('Ctrl Pts',(0.187403414383106,-0.145422030492873,
-0.436655673345544));
#72431=CARTESIAN_POINT('Ctrl Pts',(0.184211833622378,-0.14939642008148,
-0.437006485523086));
#72432=CARTESIAN_POINT('Ctrl Pts',(0.183488897013931,-0.150283448142588,
-0.437084830715379));
#72433=CARTESIAN_POINT('Ctrl Pts',(0.182306219892668,-0.151713310929788,
-0.437211152784681));
#72434=CARTESIAN_POINT('Ctrl Pts',(0.181850418228026,-0.15225935750927,
-0.43725940123931));
#72435=CARTESIAN_POINT('Ctrl Pts',(0.180961816069301,-0.153314213045529,
-0.437352608865237));
#72436=CARTESIAN_POINT('Ctrl Pts',(0.180529314264568,-0.153823254099554,
-0.437397587223204));
#72437=CARTESIAN_POINT('Ctrl Pts',(0.179462826932491,-0.155067782685971,
-0.437507568946035));
#72438=CARTESIAN_POINT('Ctrl Pts',(0.178826454723412,-0.155801228015175,
-0.437572399658116));
#72439=CARTESIAN_POINT('Ctrl Pts',(0.176977415524469,-0.157906067508014,
-0.437758563791342));
#72440=CARTESIAN_POINT('Ctrl Pts',(0.175753321840142,-0.159267391888125,
-0.437879107303134));
#72441=CARTESIAN_POINT('Ctrl Pts',(0.164350572631791,-0.171656900411977,
-0.438978997848292));
#72442=CARTESIAN_POINT('Ctrl Pts',(0.153160949645616,-0.181711459257032,
-0.439893777391911));
#72443=CARTESIAN_POINT('Ctrl Pts',(0.138148528935538,-0.192822191159927,
-0.441038425045506));
#72444=CARTESIAN_POINT('Ctrl Pts',(0.135152405300156,-0.194933938540231,
-0.441263104408691));
#72445=CARTESIAN_POINT('Ctrl Pts',(0.122931893651822,-0.203130060792316,
-0.442168650629999));
#72446=CARTESIAN_POINT('Ctrl Pts',(0.113337284337999,-0.208635312100769,
-0.442856178370973));
#72447=CARTESIAN_POINT('Ctrl Pts',(0.100027671606413,-0.215082406365566,
-0.443807503838229));
#72448=CARTESIAN_POINT('Ctrl Pts',(0.0966228017272741,-0.216633349926769,
-0.444050583637591));
#72449=CARTESIAN_POINT('Ctrl Pts',(0.0917031371936131,-0.218735238080925,
-0.44440213740468));
#72450=CARTESIAN_POINT('Ctrl Pts',(0.0902170884414607,-0.219352334131449,
-0.444508369164063));
#72451=CARTESIAN_POINT('Ctrl Pts',(0.0876229608785047,-0.220398750486248,
-0.444693939303387));
#72452=CARTESIAN_POINT('Ctrl Pts',(0.0865177087370344,-0.220834957549538,
-0.44477304250186));
#72453=CARTESIAN_POINT('Ctrl Pts',(0.0842365786921663,-0.221715492184689,
-0.444936407309595));
#72454=CARTESIAN_POINT('Ctrl Pts',(0.0830603548880778,-0.222158812575235,
-0.445020699697912));
#72455=CARTESIAN_POINT('Ctrl Pts',(0.0800443984693883,-0.22326823129227,
-0.445237006210582));
#72456=CARTESIAN_POINT('Ctrl Pts',(0.0781998764283866,-0.223920940862848,
-0.445369460052377));
#72457=CARTESIAN_POINT('Ctrl Pts',(0.0708501825523862,-0.226419846148451,
-0.445898013209767));
#72458=CARTESIAN_POINT('Ctrl Pts',(0.0652864985862891,-0.228086295206418,
-0.446299910210928));
#72459=CARTESIAN_POINT('Ctrl Pts',(0.0411774939264183,-0.234353113480744,
-0.448050093494924));
#72460=CARTESIAN_POINT('Ctrl Pts',(0.0221759879560849,-0.236907139943528,
-0.449458710709847));
#72461=CARTESIAN_POINT('Ctrl Pts',(-0.00284066065774192,-0.237231848917687,
-0.451273932748468));
#72462=CARTESIAN_POINT('Ctrl Pts',(-0.0087607412272072,-0.237087068993664,
-0.451699909201556));
#72463=CARTESIAN_POINT('Ctrl Pts',(-0.0169756273633561,-0.236577993606905,
-0.452281181733561));
#72464=CARTESIAN_POINT('Ctrl Pts',(-0.0192795789151716,-0.236401391090274,
-0.45244312021214));
#72465=CARTESIAN_POINT('Ctrl Pts',(-0.0232979563725679,-0.236034233808542,
-0.452723260259365));
#72466=CARTESIAN_POINT('Ctrl Pts',(-0.0250135389880172,-0.235858596625228,
-0.452842126646201));
#72467=CARTESIAN_POINT('Ctrl Pts',(-0.027555335470836,-0.235570326833739,
-0.453016999107878));
#72468=CARTESIAN_POINT('Ctrl Pts',(-0.028383071328361,-0.235472029576621,
-0.453073750877317));
#72469=CARTESIAN_POINT('Ctrl Pts',(-0.0297986546241951,-0.235296349982555,
-0.453170452742688));
#72470=CARTESIAN_POINT('Ctrl Pts',(-0.0303867487670684,-0.235221125029791,
-0.453210521232329));
#72471=CARTESIAN_POINT('Ctrl Pts',(-0.0317263637550768,-0.235044662693193,
-0.453301549264324));
#72472=CARTESIAN_POINT('Ctrl Pts',(-0.0324776860982156,-0.234942025963743,
-0.453352429666835));
#72473=CARTESIAN_POINT('Ctrl Pts',(-0.0345381891891899,-0.234650471332525,
-0.453491527343151));
#72474=CARTESIAN_POINT('Ctrl Pts',(-0.035846326073275,-0.234454198758655,
-0.453579345008174));
#72475=CARTESIAN_POINT('Ctrl Pts',(-0.0427931742419882,-0.233352392536122,
-0.45404341983562));
#72476=CARTESIAN_POINT('Ctrl Pts',(-0.048399939233285,-0.232254284692115,
-0.454409982761481));
#72477=CARTESIAN_POINT('Ctrl Pts',(-0.070242644332587,-0.227150783254028,
-0.455825804021682));
#72478=CARTESIAN_POINT('Ctrl Pts',(-0.0860762115126081,-0.221635890598079,
-0.456828239404915));
#72479=CARTESIAN_POINT('Ctrl Pts',(-0.110897179275683,-0.209925670259526,
-0.45852886764447));
#72480=CARTESIAN_POINT('Ctrl Pts',(-0.120272781510286,-0.204698279790981,
-0.459204484337004));
#72481=CARTESIAN_POINT('Ctrl Pts',(-0.131170057264296,-0.197614716801845,
-0.460051577446284));
#72482=CARTESIAN_POINT('Ctrl Pts',(-0.133060212188065,-0.196346987655507,
-0.460200869375425));
#72483=CARTESIAN_POINT('Ctrl Pts',(-0.136022430203147,-0.194297807170501,
-0.46043877119538));
#72484=CARTESIAN_POINT('Ctrl Pts',(-0.137106715151686,-0.19353420351136,
-0.460526704445047));
#72485=CARTESIAN_POINT('Ctrl Pts',(-0.139134782726734,-0.192080347532853,
-0.460692820743926));
#72486=CARTESIAN_POINT('Ctrl Pts',(-0.140079979471034,-0.191392128729863,
-0.460770923843428));
#72487=CARTESIAN_POINT('Ctrl Pts',(-0.142198817739738,-0.189825251910599,
-0.460947577442449));
#72488=CARTESIAN_POINT('Ctrl Pts',(-0.143369469312758,-0.188942650374211,
-0.461046279823175));
#72489=CARTESIAN_POINT('Ctrl Pts',(-0.146796749557804,-0.186308494317819,
-0.461338566674719));
#72490=CARTESIAN_POINT('Ctrl Pts',(-0.149029933676435,-0.18452701255234,
-0.46153332556047));
#72491=CARTESIAN_POINT('Ctrl Pts',(-0.166631517953804,-0.169957717901932,
-0.463103962006038));
#72492=CARTESIAN_POINT('Ctrl Pts',(-0.180356218749445,-0.155315811630681,
-0.464560004873317));
#72493=CARTESIAN_POINT('Ctrl Pts',(-0.196891452236667,-0.132487819079628,
-0.466617053257804));
#72494=CARTESIAN_POINT('Ctrl Pts',(-0.201355788173507,-0.125599084031395,
-0.467213298114807));
#72495=CARTESIAN_POINT('Ctrl Pts',(-0.2075677115856,-0.114828213116781,
-0.468096700864029));
#72496=CARTESIAN_POINT('Ctrl Pts',(-0.209582769928244,-0.111107791776598,
-0.468393488839807));
#72497=CARTESIAN_POINT('Ctrl Pts',(-0.212027228168022,-0.106291137612642,
-0.468765412395763));
#72498=CARTESIAN_POINT('Ctrl Pts',(-0.212549361757136,-0.105243148844418,
-0.468845604880173));
#72499=CARTESIAN_POINT('Ctrl Pts',(-0.213378761086747,-0.103547086929671,
-0.468974165816297));
#72500=CARTESIAN_POINT('Ctrl Pts',(-0.213690877402603,-0.102901427804725,
-0.469022823232137));
#72501=CARTESIAN_POINT('Ctrl Pts',(-0.214286702653162,-0.101654472148345,
-0.469116235895805));
#72502=CARTESIAN_POINT('Ctrl Pts',(-0.214570816903586,-0.101053387804816,
-0.469161014465183));
#72503=CARTESIAN_POINT('Ctrl Pts',(-0.215193257597783,-0.099722064756122,
-0.469259656831312));
#72504=CARTESIAN_POINT('Ctrl Pts',(-0.215530405607414,-0.0989912754775003,
-0.469313449126351));
#72505=CARTESIAN_POINT('Ctrl Pts',(-0.216712615039491,-0.0963940899296627,
-0.469503419858634));
#72506=CARTESIAN_POINT('Ctrl Pts',(-0.217537235187122,-0.0945184114141076,
-0.469638420469324));
#72507=CARTESIAN_POINT('Ctrl Pts',(-0.224065539945921,-0.0791309594976372,
-0.470729992054561));
#72508=CARTESIAN_POINT('Ctrl Pts',(-0.228529786552498,-0.0651255177717425,
-0.471625291624658));
#72509=CARTESIAN_POINT('Ctrl Pts',(-0.23532626214526,-0.0341277841372568,
-0.473570121112919));
#72510=CARTESIAN_POINT('Ctrl Pts',(-0.237170985036829,-0.01711657282713,
-0.474617686914739));
#72511=CARTESIAN_POINT('Ctrl Pts',(-0.237175510836601,0.00214638939489631,
-0.475870955694842));
#72512=CARTESIAN_POINT('Ctrl Pts',(-0.237145359082231,0.00434834028815707,
-0.47601512181016));
#72513=CARTESIAN_POINT('Ctrl Pts',(-0.237044903180087,0.00798473490960728,
-0.476254855331902));
#72514=CARTESIAN_POINT('Ctrl Pts',(-0.236992223209531,0.00941955946395762,
-0.476349872605398));
#72515=CARTESIAN_POINT('Ctrl Pts',(-0.236873117601517,0.0120195060600362,
-0.476522857117236));
#72516=CARTESIAN_POINT('Ctrl Pts',(-0.236811113601335,0.0131847927332773,
-0.476600683486768));
#72517=CARTESIAN_POINT('Ctrl Pts',(-0.236658971904528,0.0156948426340991,
-0.476768981640673));
#72518=CARTESIAN_POINT('Ctrl Pts',(-0.236565966107027,0.0170393843122896,
-0.476859540754235));
#72519=CARTESIAN_POINT('Ctrl Pts',(-0.236277335842771,0.0207520433863723,
-0.477110764543423));
#72520=CARTESIAN_POINT('Ctrl Pts',(-0.236057579516744,0.0231180702826091,
-0.477272178452543));
#72521=CARTESIAN_POINT('Ctrl Pts',(-0.234371341527379,0.0387230070048102,
-0.478345799241754));
#72522=CARTESIAN_POINT('Ctrl Pts',(-0.231827622907716,0.051819307098901,
-0.479291876888957));
#72523=CARTESIAN_POINT('Ctrl Pts',(-0.224751972433897,0.0768019941004218,
-0.481174563573363));
#72524=CARTESIAN_POINT('Ctrl Pts',(-0.220336789296876,0.0886774573073427,
-0.482105981532162));
#72525=CARTESIAN_POINT('Ctrl Pts',(-0.21209038525342,0.106381357016382,
-0.483514374959463));
#72526=CARTESIAN_POINT('Ctrl Pts',(-0.208914736192351,0.112489897628098,
-0.484003931083776));
#72527=CARTESIAN_POINT('Ctrl Pts',(-0.204783659210171,0.119656024480095,
-0.484575659483176));
#72528=CARTESIAN_POINT('Ctrl Pts',(-0.204079126485024,0.120853720008388,
-0.484671121043142));
#72529=CARTESIAN_POINT('Ctrl Pts',(-0.202966120490294,0.122708323604762,
-0.484818713877912));
#72530=CARTESIAN_POINT('Ctrl Pts',(-0.202564904912202,0.123369518479409,
-0.484871287542501));
#72531=CARTESIAN_POINT('Ctrl Pts',(-0.201816990583711,0.124588580189074,
-0.484968117648391));
#72532=CARTESIAN_POINT('Ctrl Pts',(-0.201471208877567,0.125146969650448,
-0.485012428985358));
#72533=CARTESIAN_POINT('Ctrl Pts',(-0.200673488157288,0.126423302483734,
-0.485113625113941));
#72534=CARTESIAN_POINT('Ctrl Pts',(-0.200220013014459,0.127140263899515,
-0.485170408317801));
#72535=CARTESIAN_POINT('Ctrl Pts',(-0.198791562366065,0.129372101639205,
-0.485347025530662));
#72536=CARTESIAN_POINT('Ctrl Pts',(-0.197803140658203,0.130878355659917,
-0.485466015018669));
#72537=CARTESIAN_POINT('Ctrl Pts',(-0.18864869768923,0.144488148110305,
-0.486540663785389));
#72538=CARTESIAN_POINT('Ctrl Pts',(-0.179397232324798,0.155826553017773,
-0.487433626443334));
#72539=CARTESIAN_POINT('Ctrl Pts',(-0.15774239696061,0.177861371996881,
-0.489327073172076));
#72540=CARTESIAN_POINT('Ctrl Pts',(-0.145159473051866,0.188271021835937,
-0.490324847174287));
#72541=CARTESIAN_POINT('Ctrl Pts',(-0.129223059709154,0.198901015833218,
-0.491562713949262));
#72542=CARTESIAN_POINT('Ctrl Pts',(-0.12680748098783,0.200449681668915,
-0.491749589634421));
#72543=CARTESIAN_POINT('Ctrl Pts',(-0.12311560389951,0.202723160656437,
-0.492034416923675));
#72544=CARTESIAN_POINT('Ctrl Pts',(-0.12185964127556,0.203480611992349,
-0.492131178801979));
#72545=CARTESIAN_POINT('Ctrl Pts',(-0.119656643881099,0.204781493783321,
-0.492300710836373));
#72546=CARTESIAN_POINT('Ctrl Pts',(-0.118712722098046,0.205330129705883,
-0.492373289982694));
#72547=CARTESIAN_POINT('Ctrl Pts',(-0.116723903225186,0.206467793501117,
-0.492526104654826));
#72548=CARTESIAN_POINT('Ctrl Pts',(-0.115678261094875,0.207055449471853,
-0.492606386866096));
#72549=CARTESIAN_POINT('Ctrl Pts',(-0.113163273995616,0.208443887393663,
-0.492799359829047));
#72550=CARTESIAN_POINT('Ctrl Pts',(-0.111689840898464,0.209237090313794,
-0.492912316323004));
#72551=CARTESIAN_POINT('Ctrl Pts',(-0.106542987048353,0.211937975373904,
-0.493306621938611));
#72552=CARTESIAN_POINT('Ctrl Pts',(-0.102828297687207,0.213764943205885,
-0.493590763661581));
#72553=CARTESIAN_POINT('Ctrl Pts',(-0.0936053500143426,0.218004965719879,
-0.494295595237789));
#72554=CARTESIAN_POINT('Ctrl Pts',(-0.088049706851249,0.220307434051798,
-0.494719664064118));
#72555=CARTESIAN_POINT('Ctrl Pts',(-0.0722385820114713,0.226166534839886,
-0.495924181426436));
#72556=CARTESIAN_POINT('Ctrl Pts',(-0.0618181169873884,0.229233947684174,
-0.496715919119564));
#72557=CARTESIAN_POINT('Ctrl Pts',(-0.0481417438444124,0.232259177699159,
-0.497738874503745));
#72558=CARTESIAN_POINT('Ctrl Pts',(-0.0450458290258016,0.232879402586337,
-0.497969329421446));
#72559=CARTESIAN_POINT('Ctrl Pts',(-0.0419392658597717,0.233437526126678,
-0.498199055407226));
#72560=CARTESIAN_POINT('Ctrl Pts',(-0.0419392867764624,0.233437522368795,
-0.517737946518584));
#72561=CARTESIAN_POINT('Ctrl Pts',(-0.0514623511486289,0.231726612641677,
-0.51703411206606));
#72562=CARTESIAN_POINT('Ctrl Pts',(-0.0608759382465519,0.229433824766293,
-0.516337312495976));
#72563=CARTESIAN_POINT('Ctrl Pts',(-0.0715629283511039,0.226126043590324,
-0.515562958538504));
#72564=CARTESIAN_POINT('Ctrl Pts',(-0.0729947285602193,0.225667920181476,
-0.515459576608732));
#72565=CARTESIAN_POINT('Ctrl Pts',(-0.0751711249529407,0.224948671643561,
-0.515303087799546));
#72566=CARTESIAN_POINT('Ctrl Pts',(-0.0759189023175492,0.224697403673176,
-0.515249439445631));
#72567=CARTESIAN_POINT('Ctrl Pts',(-0.0772855192608476,0.224230592288743,
-0.515151629011857));
#72568=CARTESIAN_POINT('Ctrl Pts',(-0.0779047229749196,0.224016214068525,
-0.515107402689105));
#72569=CARTESIAN_POINT('Ctrl Pts',(-0.0793041858884918,0.223525193222377,
-0.515007647748705));
#72570=CARTESIAN_POINT('Ctrl Pts',(-0.0800838910345873,0.223247029887003,
-0.514952209355774));
#72571=CARTESIAN_POINT('Ctrl Pts',(-0.0821041079633582,0.222514362342653,
-0.514808892137006));
#72572=CARTESIAN_POINT('Ctrl Pts',(-0.0833423270342379,0.222053558208546,
-0.514721369203872));
#72573=CARTESIAN_POINT('Ctrl Pts',(-0.0922251708022917,0.218663030614834,
-0.514095341158277));
#72574=CARTESIAN_POINT('Ctrl Pts',(-0.0997183114492473,0.215349233822919,
-0.51357708992896));
#72575=CARTESIAN_POINT('Ctrl Pts',(-0.117882231037556,0.206164397940351,
-0.512310166070876));
#72576=CARTESIAN_POINT('Ctrl Pts',(-0.128300448376669,0.199847423043494,
-0.511573089755153));
#72577=CARTESIAN_POINT('Ctrl Pts',(-0.147672766592826,0.185959463134733,
-0.510103593364523));
#72578=CARTESIAN_POINT('Ctrl Pts',(-0.156641371690452,0.17847016250468,
-0.509374149377564));
#72579=CARTESIAN_POINT('Ctrl Pts',(-0.167033702916567,0.168402995036752,
-0.508435998315449));
#72580=CARTESIAN_POINT('Ctrl Pts',(-0.169010830082696,0.166418643426867,
-0.508252955764386));
#72581=CARTESIAN_POINT('Ctrl Pts',(-0.171947491464907,0.163364935657382,
-0.507973758136767));
#72582=CARTESIAN_POINT('Ctrl Pts',(-0.172933261847976,0.162321067077269,
-0.507878743396792));
#72583=CARTESIAN_POINT('Ctrl Pts',(-0.174702685431904,0.16041294584397,
-0.507705786759474));
#72584=CARTESIAN_POINT('Ctrl Pts',(-0.175489560840209,0.159551732814112,
-0.507627985883393));
#72585=CARTESIAN_POINT('Ctrl Pts',(-0.177171215091402,0.157683719433989,
-0.507459769557748));
#72586=CARTESIAN_POINT('Ctrl Pts',(-0.178063830872781,0.156675035778925,
-0.50736926704471));
#72587=CARTESIAN_POINT('Ctrl Pts',(-0.180464769243914,0.153914879862574,
-0.507122470887297));
#72588=CARTESIAN_POINT('Ctrl Pts',(-0.181956124299485,0.152148911765601,
-0.506965487148934));
#72589=CARTESIAN_POINT('Ctrl Pts',(-0.190134593628091,0.142172246476447,
-0.506083409527655));
#72590=CARTESIAN_POINT('Ctrl Pts',(-0.196290863209069,0.133543816870864,
-0.505337518261049));
#72591=CARTESIAN_POINT('Ctrl Pts',(-0.210478725735969,0.110547602358844,
-0.50339438022508));
#72592=CARTESIAN_POINT('Ctrl Pts',(-0.217630301738286,0.0957030689456048,
-0.502178219779088));
#72593=CARTESIAN_POINT('Ctrl Pts',(-0.225244129204583,0.0745247350646868,
-0.500561877307296));
#72594=CARTESIAN_POINT('Ctrl Pts',(-0.2270784659515,0.0687330955978113,
-0.500131726981203));
#72595=CARTESIAN_POINT('Ctrl Pts',(-0.229035072486159,0.0616167527717919,
-0.499622377079648));
#72596=CARTESIAN_POINT('Ctrl Pts',(-0.229371133830322,0.0603537224358601,
-0.49953270127418));
#72597=CARTESIAN_POINT('Ctrl Pts',(-0.229882831118833,0.0583645653148398,
-0.499392675940227));
#72598=CARTESIAN_POINT('Ctrl Pts',(-0.230065500234272,0.0576402998658913,
-0.499341941857678));
#72599=CARTESIAN_POINT('Ctrl Pts',(-0.230403405875435,0.0562733357002763,
-0.49924667385942));
#72600=CARTESIAN_POINT('Ctrl Pts',(-0.230559375793822,0.0556308547037943,
-0.499202101263233));
#72601=CARTESIAN_POINT('Ctrl Pts',(-0.230915453123314,0.0541368562435719,
-0.49909891527044));
#72602=CARTESIAN_POINT('Ctrl Pts',(-0.231113539158999,0.0532848737760093,
-0.499040417231651));
#72603=CARTESIAN_POINT('Ctrl Pts',(-0.231748558272797,0.0504834380976598,
-0.498849142919466));
#72604=CARTESIAN_POINT('Ctrl Pts',(-0.232165588398956,0.0485294961560803,
-0.498717438937636));
#72605=CARTESIAN_POINT('Ctrl Pts',(-0.235613769565828,0.0313103810206143,
-0.497569871360487));
#72606=CARTESIAN_POINT('Ctrl Pts',(-0.237160675224263,0.0157842829669599,
-0.496623519766758));
#72607=CARTESIAN_POINT('Ctrl Pts',(-0.237188604127509,-0.0147789281299883,
-0.494750069891481));
#72608=CARTESIAN_POINT('Ctrl Pts',(-0.23578018455968,-0.0297402292983789,
-0.493827016014195));
#72609=CARTESIAN_POINT('Ctrl Pts',(-0.23236734549757,-0.0476203715957152,
-0.492651002314969));
#72610=CARTESIAN_POINT('Ctrl Pts',(-0.231701642444954,-0.0507605193646444,
-0.492441802332666));
#72611=CARTESIAN_POINT('Ctrl Pts',(-0.230631972160886,-0.0553454584455917,
-0.492131964310255));
#72612=CARTESIAN_POINT('Ctrl Pts',(-0.230277679226126,-0.0568015548231795,
-0.492032911674053));
#72613=CARTESIAN_POINT('Ctrl Pts',(-0.229620965763451,-0.0593933820801181,
-0.491855385340801));
#72614=CARTESIAN_POINT('Ctrl Pts',(-0.229323854684311,-0.0605304166555545,
-0.491777085035815));
#72615=CARTESIAN_POINT('Ctrl Pts',(-0.228682341034493,-0.062912934223662,
-0.491612111504454));
#72616=CARTESIAN_POINT('Ctrl Pts',(-0.228336186359553,-0.064157901132294,
-0.491525383708313));
#72617=CARTESIAN_POINT('Ctrl Pts',(-0.227395156112566,-0.0674382697546252,
-0.491295450577449));
#72618=CARTESIAN_POINT('Ctrl Pts',(-0.226783138195888,-0.0694685898179573,
-0.491151692167827));
#72619=CARTESIAN_POINT('Ctrl Pts',(-0.22366841892273,-0.0793213156881715,
-0.490446793698876));
#72620=CARTESIAN_POINT('Ctrl Pts',(-0.220788051571348,-0.0870174763010837,
-0.48987342836396));
#72621=CARTESIAN_POINT('Ctrl Pts',(-0.213652113992268,-0.103434223423304,
-0.488599857345659));
#72622=CARTESIAN_POINT('Ctrl Pts',(-0.209248903577,-0.112074677576266,-0.487896429064942));
#72623=CARTESIAN_POINT('Ctrl Pts',(-0.197020347226297,-0.132824059607327,
-0.486138401879095));
#72624=CARTESIAN_POINT('Ctrl Pts',(-0.18859589810098,-0.144536876232833,
-0.485081792203671));
#72625=CARTESIAN_POINT('Ctrl Pts',(-0.177810426369258,-0.156970307311911,
-0.483934427361521));
#72626=CARTESIAN_POINT('Ctrl Pts',(-0.176440148551139,-0.158508989664251,
-0.483791980227073));
#72627=CARTESIAN_POINT('Ctrl Pts',(-0.174505815557176,-0.16062487754063,
-0.483595689220372));
#72628=CARTESIAN_POINT('Ctrl Pts',(-0.173958651448422,-0.161217302366558,
-0.483540684589748));
#72629=CARTESIAN_POINT('Ctrl Pts',(-0.172954742711665,-0.162293191194496,
-0.483440727706311));
#72630=CARTESIAN_POINT('Ctrl Pts',(-0.172498966030143,-0.162777546661928,
-0.483395704187179));
#72631=CARTESIAN_POINT('Ctrl Pts',(-0.171548327053136,-0.163779317003408,
-0.483302545048399));
#72632=CARTESIAN_POINT('Ctrl Pts',(-0.171053151864804,-0.164296416468658,
-0.483254434112858));
#72633=CARTESIAN_POINT('Ctrl Pts',(-0.169745288109525,-0.165649864728131,
-0.483128421265536));
#72634=CARTESIAN_POINT('Ctrl Pts',(-0.16892874727279,-0.166482488580105,
-0.483050810577667));
#72635=CARTESIAN_POINT('Ctrl Pts',(-0.165155689556132,-0.170273519791817,
-0.482696832755316));
#72636=CARTESIAN_POINT('Ctrl Pts',(-0.162127181963509,-0.173159624008968,
-0.482425631234877));
#72637=CARTESIAN_POINT('Ctrl Pts',(-0.153048168132241,-0.181364573800002,
-0.481643757450121));
#72638=CARTESIAN_POINT('Ctrl Pts',(-0.146800956810188,-0.186457365572262,
-0.481144171665557));
#72639=CARTESIAN_POINT('Ctrl Pts',(-0.123978034154506,-0.203203279985697,
-0.479402201908506));
#72640=CARTESIAN_POINT('Ctrl Pts',(-0.106184579874836,-0.213041973453268,
-0.478179868526611));
#72641=CARTESIAN_POINT('Ctrl Pts',(-0.0849653580669599,-0.221448622922334,
-0.476700754035614));
#72642=CARTESIAN_POINT('Ctrl Pts',(-0.0825573869965616,-0.222357553689453,
-0.476532763417803));
#72643=CARTESIAN_POINT('Ctrl Pts',(-0.078696082338833,-0.223743704105128,
-0.476262908351054));
#72644=CARTESIAN_POINT('Ctrl Pts',(-0.0772520564513907,-0.224246378103167,
-0.476161886098676));
#72645=CARTESIAN_POINT('Ctrl Pts',(-0.0746856261138126,-0.225112036978749,
-0.475982110346465));
#72646=CARTESIAN_POINT('Ctrl Pts',(-0.0735651740691968,-0.225480679923413,
-0.47590354642424));
#72647=CARTESIAN_POINT('Ctrl Pts',(-0.0712256807259108,-0.226231109220051,
-0.475739322221883));
#72648=CARTESIAN_POINT('Ctrl Pts',(-0.0700062144122565,-0.226611434412937,
-0.475653616889312));
#72649=CARTESIAN_POINT('Ctrl Pts',(-0.0668195534499327,-0.227577108437216,
-0.475429356496869));
#72650=CARTESIAN_POINT('Ctrl Pts',(-0.0648477636399524,-0.228146795061074,
-0.475290296577235));
#72651=CARTESIAN_POINT('Ctrl Pts',(-0.0557572574911122,-0.230645845931149,
-0.474647667199291));
#72652=CARTESIAN_POINT('Ctrl Pts',(-0.0485590568855369,-0.232267896181336,
-0.474134356723536));
#72653=CARTESIAN_POINT('Ctrl Pts',(-0.0284951742657086,-0.235815676410801,
-0.472690872100666));
#72654=CARTESIAN_POINT('Ctrl Pts',(-0.0155294289507012,-0.237022743404765,
-0.471742669150701));
#72655=CARTESIAN_POINT('Ctrl Pts',(0.0094366785587664,-0.237289243673352,
-0.469919356345127));
#72656=CARTESIAN_POINT('Ctrl Pts',(0.0213986745210681,-0.236510867068765,
-0.469047370412982));
#72657=CARTESIAN_POINT('Ctrl Pts',(0.035304013149444,-0.234541901188131,
-0.468067716503805));
#72658=CARTESIAN_POINT('Ctrl Pts',(0.0373524440351625,-0.234224406099606,
-0.46792430451187));
#72659=CARTESIAN_POINT('Ctrl Pts',(0.0402181788888056,-0.233741679995695,
-0.467725182387074));
#72660=CARTESIAN_POINT('Ctrl Pts',(0.0410391039769695,-0.233598944513275,
-0.467668315845569));
#72661=CARTESIAN_POINT('Ctrl Pts',(0.0425206148403899,-0.233333301031761,
-0.467566025705486));
#72662=CARTESIAN_POINT('Ctrl Pts',(0.0431814617101092,-0.233211906775567,
-0.467520519028002));
#72663=CARTESIAN_POINT('Ctrl Pts',(0.044533968352047,-0.232957511867592,
-0.467427644080444));
#72664=CARTESIAN_POINT('Ctrl Pts',(0.0452255655488018,-0.232824236123435,
-0.467380291629511));
#72665=CARTESIAN_POINT('Ctrl Pts',(0.0470088738068744,-0.232472333827784,
-0.467258525621523));
#72666=CARTESIAN_POINT('Ctrl Pts',(0.0480996729121381,-0.232249094292064,
-0.4671843684625));
#72667=CARTESIAN_POINT('Ctrl Pts',(0.0527646357164179,-0.23126010141126,
-0.466868453991817));
#72668=CARTESIAN_POINT('Ctrl Pts',(0.0563226241436127,-0.230419415123055,
-0.466630601618582));
#72669=CARTESIAN_POINT('Ctrl Pts',(0.0661697280620907,-0.227850980099421,
-0.465977358646288));
#72670=CARTESIAN_POINT('Ctrl Pts',(0.0724093857151596,-0.225945558088657,
-0.465569183306518));
#72671=CARTESIAN_POINT('Ctrl Pts',(0.0823864202456606,-0.222442978584746,
-0.464914471010075));
#72672=CARTESIAN_POINT('Ctrl Pts',(0.0861748967030278,-0.221002916982992,
-0.464665377033247));
#72673=CARTESIAN_POINT('Ctrl Pts',(0.106553528967471,-0.212652931231677,
-0.463314298453605));
#72674=CARTESIAN_POINT('Ctrl Pts',(0.122352154159339,-0.203972519875487,
-0.462220545870337));
#72675=CARTESIAN_POINT('Ctrl Pts',(0.139551044774914,-0.191799667874045,
-0.460857998384811));
#72676=CARTESIAN_POINT('Ctrl Pts',(0.142047991959621,-0.189957819576722,
-0.46065564795281));
#72677=CARTESIAN_POINT('Ctrl Pts',(0.145693190100282,-0.187156910089194,
-0.460353015817484));
#72678=CARTESIAN_POINT('Ctrl Pts',(0.146869720775871,-0.186235065395491,
-0.460254189487388));
#72679=CARTESIAN_POINT('Ctrl Pts',(0.148952883987814,-0.184570831629846,
-0.460077099347008));
#72680=CARTESIAN_POINT('Ctrl Pts',(0.149862883847405,-0.183832721508379,
-0.459999008289518));
#72681=CARTESIAN_POINT('Ctrl Pts',(0.151776956454218,-0.182256540535712,
-0.459833173423538));
#72682=CARTESIAN_POINT('Ctrl Pts',(0.152779637791821,-0.181416849371181,
-0.459745365394014));
#72683=CARTESIAN_POINT('Ctrl Pts',(0.155444549125654,-0.179147369388942,
-0.459509435362496));
#72684=CARTESIAN_POINT('Ctrl Pts',(0.157093949148122,-0.177702781040604,
-0.459360707463244));
#72685=CARTESIAN_POINT('Ctrl Pts',(0.165595322110128,-0.170046189899455,
-0.458579629646133));
#72686=CARTESIAN_POINT('Ctrl Pts',(0.172098807595499,-0.16346093926156,
-0.457931581224259));
#72687=CARTESIAN_POINT('Ctrl Pts',(0.185283715097079,-0.148449089382346,
-0.456503245439868));
#72688=CARTESIAN_POINT('Ctrl Pts',(0.191810725852447,-0.139913553763965,
-0.455719874969718));
#72689=CARTESIAN_POINT('Ctrl Pts',(0.204411021810946,-0.120889215053568,
-0.454053417957853));
#72690=CARTESIAN_POINT('Ctrl Pts',(0.210305811315452,-0.11031587462482,
-0.453172508836579));
#72691=CARTESIAN_POINT('Ctrl Pts',(0.21623846239433,-0.0974536575230821,
-0.452184422248417));
#72692=CARTESIAN_POINT('Ctrl Pts',(0.217082992328944,-0.0955576431178358,
-0.452040819644487));
#72693=CARTESIAN_POINT('Ctrl Pts',(0.218231746381074,-0.0928847701260245,
-0.451841478060546));
#72694=CARTESIAN_POINT('Ctrl Pts',(0.218556898643629,-0.0921170872198375,
-0.451784579434576));
#72695=CARTESIAN_POINT('Ctrl Pts',(0.219136826062409,-0.0907275244071472,
-0.451682248749058));
#72696=CARTESIAN_POINT('Ctrl Pts',(0.219393018375959,-0.0901062470092216,
-0.451636733407867));
#72697=CARTESIAN_POINT('Ctrl Pts',(0.21991223233453,-0.0888317875940768,
-0.451543861744528));
#72698=CARTESIAN_POINT('Ctrl Pts',(0.220174991358857,-0.0881785100269253,
-0.451496521097271));
#72699=CARTESIAN_POINT('Ctrl Pts',(0.220845399946186,-0.0864900439209981,
-0.451374821448213));
#72700=CARTESIAN_POINT('Ctrl Pts',(0.221248687831748,-0.0854531253327159,
-0.451300718312726));
#72701=CARTESIAN_POINT('Ctrl Pts',(0.222942878341639,-0.0810046801372399,
-0.450985362135807));
#72702=CARTESIAN_POINT('Ctrl Pts',(0.224162362922549,-0.0775662542901242,
-0.450747996940529));
#72703=CARTESIAN_POINT('Ctrl Pts',(0.227332931836171,-0.0679262032263988,
-0.45009653729647));
#72704=CARTESIAN_POINT('Ctrl Pts',(0.229109202077763,-0.0616702256393484,
-0.449689610618353));
#72705=CARTESIAN_POINT('Ctrl Pts',(0.231612389548724,-0.0512399843677539,
-0.449025390541219));
#72706=CARTESIAN_POINT('Ctrl Pts',(0.232488508698639,-0.0471055159063544,
-0.4487657115224));
#72707=CARTESIAN_POINT('Ctrl Pts',(0.23647883700083,-0.0254346505775926,
-0.447414084391004));
#72708=CARTESIAN_POINT('Ctrl Pts',(0.237720636882419,-0.00761416327510002,
-0.446329478342523));
#72709=CARTESIAN_POINT('Ctrl Pts',(0.236822961484322,0.0132876600504383,
-0.444976746520249));
#72710=CARTESIAN_POINT('Ctrl Pts',(0.236628102131184,0.0163956337452305,
-0.444773672864555));
#72711=CARTESIAN_POINT('Ctrl Pts',(0.236249063767338,0.0209904960157593,
-0.444470166132395));
#72712=CARTESIAN_POINT('Ctrl Pts',(0.236111891245874,0.0224810073932401,
-0.444371200947694));
#72713=CARTESIAN_POINT('Ctrl Pts',(0.23584217899795,0.0251360438902577,
-0.444193956681814));
#72714=CARTESIAN_POINT('Ctrl Pts',(0.235715097169576,0.0263010832222142,
-0.44411585151076));
#72715=CARTESIAN_POINT('Ctrl Pts',(0.235428080119742,0.0287629444071511,
-0.44395008621603));
#72716=CARTESIAN_POINT('Ctrl Pts',(0.235266052674576,0.0300594780412402,
-0.443862362613071));
#72717=CARTESIAN_POINT('Ctrl Pts',(0.234804215254474,0.0335222856539613,
-0.44362690176707));
#72718=CARTESIAN_POINT('Ctrl Pts',(0.234485148629836,0.0356858186086232,
-0.44347856282941));
#72719=CARTESIAN_POINT('Ctrl Pts',(0.23267450102878,0.0468879065362686,
-0.442703917987147));
#72720=CARTESIAN_POINT('Ctrl Pts',(0.230690270873367,0.0558378010345413,
-0.442062225799171));
#72721=CARTESIAN_POINT('Ctrl Pts',(0.225251352603745,0.0750355546668417,
-0.440636343388626));
#72722=CARTESIAN_POINT('Ctrl Pts',(0.221603480165496,0.0852078216531518,
-0.439848589708582));
#72723=CARTESIAN_POINT('Ctrl Pts',(0.212413278523452,0.106205752846442,
-0.438174641943308));
#72724=CARTESIAN_POINT('Ctrl Pts',(0.206705141033089,0.116927781852566,
-0.43729063317855));
#72725=CARTESIAN_POINT('Ctrl Pts',(0.19908986164733,0.128916656490078,-0.436299888886334));
#72726=CARTESIAN_POINT('Ctrl Pts',(0.197955516287549,0.130651795370431,
-0.436156467143259));
#72727=CARTESIAN_POINT('Ctrl Pts',(0.196333471553988,0.133063303984531,
-0.435957333790632));
#72728=CARTESIAN_POINT('Ctrl Pts',(0.195864773267705,0.133752254430053,
-0.435900465606926));
#72729=CARTESIAN_POINT('Ctrl Pts',(0.195011593591186,0.134992260630924,
-0.43579817339183));
#72730=CARTESIAN_POINT('Ctrl Pts',(0.194628383583158,0.135544178811035,
-0.435752666271157));
#72731=CARTESIAN_POINT('Ctrl Pts',(0.193838688223285,0.136671283038966,
-0.435659791492658));
#72732=CARTESIAN_POINT('Ctrl Pts',(0.193431978203111,0.137246298678765,
-0.435612439646585));
#72733=CARTESIAN_POINT('Ctrl Pts',(0.192375766403062,0.138725573051882,
-0.435490677039562));
#72734=CARTESIAN_POINT('Ctrl Pts',(0.191722439098596,0.139627098321284,
-0.435416522649381));
#72735=CARTESIAN_POINT('Ctrl Pts',(0.188897318589356,0.143468259334777,
-0.435100636820759));
#72736=CARTESIAN_POINT('Ctrl Pts',(0.186663952874782,0.146362258358951,
-0.434862809442849));
#72737=CARTESIAN_POINT('Ctrl Pts',(0.180262935483613,0.154271715467041,
-0.434209658028853));
#72738=CARTESIAN_POINT('Ctrl Pts',(0.175953889872365,0.159168869607122,
-0.43380154680976));
#72739=CARTESIAN_POINT('Ctrl Pts',(0.168641375131357,0.166818968297945,
-0.43314628192893));
#72740=CARTESIAN_POINT('Ctrl Pts',(0.165759502591866,0.169682851439624,
-0.432896580774437));
#72741=CARTESIAN_POINT('Ctrl Pts',(0.149744292150789,0.184800513316992,
-0.431545486892093));
#72742=CARTESIAN_POINT('Ctrl Pts',(0.135326600557098,0.195604725745614,
-0.430452273013452));
#72743=CARTESIAN_POINT('Ctrl Pts',(0.117150411071567,0.206245950702394,
-0.429090302541077));
#72744=CARTESIAN_POINT('Ctrl Pts',(0.114441922270815,0.207761054976932,
-0.428887907784918));
#72745=CARTESIAN_POINT('Ctrl Pts',(0.110385963612875,0.209926544454168,
-0.42858522204126));
#72746=CARTESIAN_POINT('Ctrl Pts',(0.109060741340316,0.210618065595952,
-0.428486387192704));
#72747=CARTESIAN_POINT('Ctrl Pts',(0.106685214654437,0.21182922023441,-0.428309287602884));
#72748=CARTESIAN_POINT('Ctrl Pts',(0.105637420018949,0.212353688402477,
-0.428231195685402));
#72749=CARTESIAN_POINT('Ctrl Pts',(0.1034120445917,0.213447042412632,-0.428065365116619));
#72750=CARTESIAN_POINT('Ctrl Pts',(0.102233562431806,0.214013993642643,
-0.42797756228994));
#72751=CARTESIAN_POINT('Ctrl Pts',(0.0990672143205684,0.215505158490184,
-0.427741661176857));
#72752=CARTESIAN_POINT('Ctrl Pts',(0.0970711631449704,0.216411587055149,
-0.427592957252577));
#72753=CARTESIAN_POINT('Ctrl Pts',(0.0865946862030465,0.220994970148713,
-0.42681227857495));
#72754=CARTESIAN_POINT('Ctrl Pts',(0.0779182515088997,0.224201078261169,
-0.426164624792756));
#72755=CARTESIAN_POINT('Ctrl Pts',(0.0588060693320402,0.230019816604003,
-0.424736438060719));
#72756=CARTESIAN_POINT('Ctrl Pts',(0.0483344366950005,0.232445739595188,
-0.423952792161658));
#72757=CARTESIAN_POINT('Ctrl Pts',(0.0258001242724952,0.236077280990494,
-0.422285869348412));
#72758=CARTESIAN_POINT('Ctrl Pts',(0.0137341111087947,0.237085557425128,
-0.421404770354038));
#72759=CARTESIAN_POINT('Ctrl Pts',(-0.000432393023030546,0.237183684747741,
-0.420416521983644));
#72760=CARTESIAN_POINT('Ctrl Pts',(-0.0025077789487524,0.237170822514593,
-0.420272931411953));
#72761=CARTESIAN_POINT('Ctrl Pts',(-0.00541631169140616,0.237114611884206,
-0.420073603679899));
#72762=CARTESIAN_POINT('Ctrl Pts',(-0.00624973361394499,0.237094108918329,
-0.420016707078061));
#72763=CARTESIAN_POINT('Ctrl Pts',(-0.0077547477749643,0.237049142791723,
-0.419914378950628));
#72764=CARTESIAN_POINT('Ctrl Pts',(-0.0084263757899602,0.237026218893271,
-0.419868864156181));
#72765=CARTESIAN_POINT('Ctrl Pts',(-0.00980153154737315,0.236973429761481,
-0.419775992286766));
#72766=CARTESIAN_POINT('Ctrl Pts',(-0.01050503797967,0.236943285711089,
-0.41972865089578));
#72767=CARTESIAN_POINT('Ctrl Pts',(-0.0123197623723455,0.236857429576628,
-0.419606947065551));
#72768=CARTESIAN_POINT('Ctrl Pts',(-0.0134307569198347,0.236797029923703,
-0.419532840526114));
#72769=CARTESIAN_POINT('Ctrl Pts',(-0.0181824776367429,0.236505150558754,
-0.419217449203993));
#72770=CARTESIAN_POINT('Ctrl Pts',(-0.0218182432858041,0.236197494786223,
-0.418980053342243));
#72771=CARTESIAN_POINT('Ctrl Pts',(-0.030969545985803,0.235209982859015,
-0.418389173064982));
#72772=CARTESIAN_POINT('Ctrl Pts',(-0.0364708068239119,0.23441998686729,
-0.418040077434656));
#72773=CARTESIAN_POINT('Ctrl Pts',(-0.041939274266712,0.233437524616291,
-0.417694787181515));
#72774=CARTESIAN_POINT('Origin',(0.,0.,-2.1456589891905));
#72775=CARTESIAN_POINT('',(-0.0419325474085422,0.233395695413117,-0.298126337027085));
#72776=CARTESIAN_POINT('',(-0.0418736008932845,0.233079825957759,-0.317824451239062));
#72777=CARTESIAN_POINT('',(-0.0419392741328076,0.233437524640348,-2.1456589891905));
#72778=CARTESIAN_POINT('',(-0.237369928097243,-0.000181986744939411,-0.375941010809497));
#72779=CARTESIAN_POINT('Ctrl Pts',(-0.237369928097243,-0.000181986744939411,
-0.375941010809497));
#72780=CARTESIAN_POINT('Ctrl Pts',(-0.237469999104454,-0.0119683065141777,
-0.375148184390915));
#72781=CARTESIAN_POINT('Ctrl Pts',(-0.231312589235971,-0.102360953237923,
-0.369060714614336));
#72782=CARTESIAN_POINT('Ctrl Pts',(-0.115177429001217,-0.255620947329064,
-0.357678601479762));
#72783=CARTESIAN_POINT('Ctrl Pts',(0.152400560897723,-0.235333760199054,
-0.341794671405773));
#72784=CARTESIAN_POINT('Ctrl Pts',(0.280370506222409,0.000533234281509477,
-0.325910741331786));
#72785=CARTESIAN_POINT('Ctrl Pts',(0.162276893924525,0.216235263332081,
-0.311354629872224));
#72786=CARTESIAN_POINT('Ctrl Pts',(0.0163630136312862,0.243270981762062,
-0.302093161770659));
#72787=CARTESIAN_POINT('Ctrl Pts',(-0.0419325474085123,0.233395695413122,
-0.298126337027087));
#72788=CARTESIAN_POINT('Ctrl Pts',(-0.237174924912043,-0.000188727228977812,
-0.376053073332811));
#72789=CARTESIAN_POINT('Ctrl Pts',(-0.237190585303674,0.0194918044542662,
-0.377272926375048));
#72790=CARTESIAN_POINT('Ctrl Pts',(-0.234756782705812,0.0390977061925586,
-0.378451184420277));
#72791=CARTESIAN_POINT('Ctrl Pts',(-0.229105195484696,0.0614333847607206,
-0.379919998904733));
#72792=CARTESIAN_POINT('Ctrl Pts',(-0.228212702756558,0.0646700237461788,
-0.380135849644863));
#72793=CARTESIAN_POINT('Ctrl Pts',(-0.226491614925483,0.0704314095087167,
-0.380526254875689));
#72794=CARTESIAN_POINT('Ctrl Pts',(-0.225688713936378,0.0729632685109562,
-0.380699991109408));
#72795=CARTESIAN_POINT('Ctrl Pts',(-0.224395850630544,0.0768144599800887,
-0.380967855542854));
#72796=CARTESIAN_POINT('Ctrl Pts',(-0.223936367095655,0.078143857021848,
-0.381060982329268));
#72797=CARTESIAN_POINT('Ctrl Pts',(-0.223078216687786,0.080556955284831,
-0.381231271595175));
#72798=CARTESIAN_POINT('Ctrl Pts',(-0.22268340597101,0.0816419893768781,
-0.381308304032937));
#72799=CARTESIAN_POINT('Ctrl Pts',(-0.221803655756444,0.0840058897771032,
-0.38147716554136));
#72800=CARTESIAN_POINT('Ctrl Pts',(-0.221315547558358,0.0852835241817804,
-0.381569098305943));
#72801=CARTESIAN_POINT('Ctrl Pts',(-0.219939615107987,0.0887936855495577,
-0.381823555960584));
#72802=CARTESIAN_POINT('Ctrl Pts',(-0.219028896687038,0.0910170015028857,
-0.381986843881685));
#72803=CARTESIAN_POINT('Ctrl Pts',(-0.212370799921784,0.106592354277255,
-0.383146136638752));
#72804=CARTESIAN_POINT('Ctrl Pts',(-0.205441365751811,0.119402648033143,
-0.384182916473199));
#72805=CARTESIAN_POINT('Ctrl Pts',(-0.190568615642849,0.141727634527022,
-0.386133581692759));
#72806=CARTESIAN_POINT('Ctrl Pts',(-0.182967356395915,0.151413587888032,
-0.387038167992818));
#72807=CARTESIAN_POINT('Ctrl Pts',(-0.171882058048072,0.163478649016614,
-0.388215039346255));
#72808=CARTESIAN_POINT('Ctrl Pts',(-0.169037093203672,0.166418675765035,
-0.388506147198009));
#72809=CARTESIAN_POINT('Ctrl Pts',(-0.164245486320776,0.171120655449421,
-0.388976999564615));
#72810=CARTESIAN_POINT('Ctrl Pts',(-0.162343188455039,0.172926426810922,
-0.389159183029999));
#72811=CARTESIAN_POINT('Ctrl Pts',(-0.159703418668383,0.17535028397106,
-0.389405137297903));
#72812=CARTESIAN_POINT('Ctrl Pts',(-0.158991645560508,0.175995911160324,
-0.389470791627737));
#72813=CARTESIAN_POINT('Ctrl Pts',(-0.157820416812469,0.177045391888606,
-0.389577717980516));
#72814=CARTESIAN_POINT('Ctrl Pts',(-0.157363296841877,0.177451817631253,
-0.389619177469419));
#72815=CARTESIAN_POINT('Ctrl Pts',(-0.156400609881027,0.178301098009743,
-0.389705910087934));
#72816=CARTESIAN_POINT('Ctrl Pts',(-0.155894724843367,0.178743579201823,
-0.389751153800993));
#72817=CARTESIAN_POINT('Ctrl Pts',(-0.154757371946464,0.179729883221839,
-0.389852145791806));
#72818=CARTESIAN_POINT('Ctrl Pts',(-0.154124898513095,0.180272545899769,
-0.389907809728756));
#72819=CARTESIAN_POINT('Ctrl Pts',(-0.151909575130615,0.182153113904561,
-0.390101109266142));
#72820=CARTESIAN_POINT('Ctrl Pts',(-0.150312005502342,0.183473642906006,
-0.390237556081786));
#72821=CARTESIAN_POINT('Ctrl Pts',(-0.139350334965236,0.192295112575101,
-0.391155589866821));
#72822=CARTESIAN_POINT('Ctrl Pts',(-0.129444850091223,0.199098043317687,
-0.391896836478088));
#72823=CARTESIAN_POINT('Ctrl Pts',(-0.109939702884554,0.210420035364313,
-0.393281432332941));
#72824=CARTESIAN_POINT('Ctrl Pts',(-0.100470304905444,0.21510239281493,
-0.393924314566495));
#72825=CARTESIAN_POINT('Ctrl Pts',(-0.0819504608263965,0.222769402657644,
-0.395172090841339));
#72826=CARTESIAN_POINT('Ctrl Pts',(-0.0729709057571046,0.2258700938572,
-0.395773115494786));
#72827=CARTESIAN_POINT('Ctrl Pts',(-0.0617037172939343,0.229018575852127,
-0.39653613915634));
#72828=CARTESIAN_POINT('Ctrl Pts',(-0.0595688466963732,0.229583119536072,
-0.396681071878779));
#72829=CARTESIAN_POINT('Ctrl Pts',(-0.056153956429874,0.230435313952003,
-0.396913617204924));
#72830=CARTESIAN_POINT('Ctrl Pts',(-0.0548788605507008,0.230742304933986,
-0.397000605165877));
#72831=CARTESIAN_POINT('Ctrl Pts',(-0.0524601018400909,0.231303460380716,
-0.397165942201058));
#72832=CARTESIAN_POINT('Ctrl Pts',(-0.05131697020594,0.231559758060649,
-0.397244220040114));
#72833=CARTESIAN_POINT('Ctrl Pts',(-0.048716098995227,0.232122685836553,
-0.397422653988228));
#72834=CARTESIAN_POINT('Ctrl Pts',(-0.0472572871926885,0.232424069777982,
-0.397522974605593));
#72835=CARTESIAN_POINT('Ctrl Pts',(-0.0445122365249925,0.232964273359007,
-0.397712226431447));
#72836=CARTESIAN_POINT('Ctrl Pts',(-0.04322669682703,0.233206226894684,
-0.39780105124681));
#72837=CARTESIAN_POINT('Ctrl Pts',(-0.0419392740612461,0.233437524653205,
-0.397890210729054));
#72838=CARTESIAN_POINT('',(-0.236816548519718,-4.82205570482326E-5,-0.395672065486472));
#72839=CARTESIAN_POINT('Ctrl Pts',(-0.041939274266712,0.233437524616291,
-0.417694787181515));
#72840=CARTESIAN_POINT('Ctrl Pts',(-0.0428698155356764,0.233270344016001,
-0.417636030896746));
#72841=CARTESIAN_POINT('Ctrl Pts',(-0.0437994072801449,0.233097590351859,
-0.417577385479228));
#72842=CARTESIAN_POINT('Ctrl Pts',(-0.0481263531409487,0.23226667743249,
-0.417304550759911));
#72843=CARTESIAN_POINT('Ctrl Pts',(-0.0515100750404628,0.231539776861124,
-0.417091590177645));
#72844=CARTESIAN_POINT('Ctrl Pts',(-0.0730643407221923,0.226413520843067,
-0.415731321572093));
#72845=CARTESIAN_POINT('Ctrl Pts',(-0.0906745869905617,0.219953437514709,
-0.414596511065129));
#72846=CARTESIAN_POINT('Ctrl Pts',(-0.109995505769665,0.210147130652429,
-0.413194607920678));
#72847=CARTESIAN_POINT('Ctrl Pts',(-0.112622192228822,0.208751211597952,
-0.413000569756606));
#72848=CARTESIAN_POINT('Ctrl Pts',(-0.11653627827804,0.206575743854621,
-0.412705816499035));
#72849=CARTESIAN_POINT('Ctrl Pts',(-0.117843711415678,0.205832702961808,
-0.412606397290873));
#72850=CARTESIAN_POINT('Ctrl Pts',(-0.120112899086648,0.204514370675183,
-0.412432112128609));
#72851=CARTESIAN_POINT('Ctrl Pts',(-0.121077816773909,0.203944596768285,
-0.412357447253752));
#72852=CARTESIAN_POINT('Ctrl Pts',(-0.123117521890662,0.202720594792607,
-0.412198414774323));
#72853=CARTESIAN_POINT('Ctrl Pts',(-0.124191209850555,0.202064611051853,
-0.412113984670837));
#72854=CARTESIAN_POINT('Ctrl Pts',(-0.126376271600266,0.200705624901073,
-0.411940666037161));
#72855=CARTESIAN_POINT('Ctrl Pts',(-0.127487118026636,0.20000186125685,
-0.411851751454164));
#72856=CARTESIAN_POINT('Ctrl Pts',(-0.130214875953954,0.1982417635852,-0.411631398698134));
#72857=CARTESIAN_POINT('Ctrl Pts',(-0.131824822177707,0.197174863060566,
-0.411499572145909));
#72858=CARTESIAN_POINT('Ctrl Pts',(-0.144869112648568,0.188299332280254,
-0.410416684793781));
#72859=CARTESIAN_POINT('Ctrl Pts',(-0.155610667273648,0.179524090849719,
-0.409428755865637));
#72860=CARTESIAN_POINT('Ctrl Pts',(-0.175998990922182,0.159656644566247,
-0.4073594508553));
#72861=CARTESIAN_POINT('Ctrl Pts',(-0.18550737581262,0.148502279798145,
-0.406280363932357));
#72862=CARTESIAN_POINT('Ctrl Pts',(-0.196312641385644,0.133155871578909,
-0.404947002586524));
#72863=CARTESIAN_POINT('Ctrl Pts',(-0.198608427800127,0.129706733800864,
-0.404656325229395));
#72864=CARTESIAN_POINT('Ctrl Pts',(-0.201455416163695,0.1251764926425,-0.404287669095979));
#72865=CARTESIAN_POINT('Ctrl Pts',(-0.202090188945879,0.124149082556119,
-0.404204912092669));
#72866=CARTESIAN_POINT('Ctrl Pts',(-0.203093503802128,0.122497082078524,
-0.404073254579364));
#72867=CARTESIAN_POINT('Ctrl Pts',(-0.203467066745241,0.121875588984757,
-0.404024040241966));
#72868=CARTESIAN_POINT('Ctrl Pts',(-0.20417947741013,0.120677953061953,
-0.403929823028724));
#72869=CARTESIAN_POINT('Ctrl Pts',(-0.204518745392452,0.120102082182325,
-0.403884794844485));
#72870=CARTESIAN_POINT('Ctrl Pts',(-0.205327868345856,0.118715312399557,
-0.403777004447757));
#72871=CARTESIAN_POINT('Ctrl Pts',(-0.205795366284811,0.117903037312684,
-0.403714392515051));
#72872=CARTESIAN_POINT('Ctrl Pts',(-0.207399599021535,0.115077077996875,
-0.403498296667782));
#72873=CARTESIAN_POINT('Ctrl Pts',(-0.208511734536915,0.113049480760451,
-0.403346286137321));
#72874=CARTESIAN_POINT('Ctrl Pts',(-0.211186592785501,0.107998985907927,
-0.40297427101964));
#72875=CARTESIAN_POINT('Ctrl Pts',(-0.212714293180425,0.104958038560421,
-0.402756033157679));
#72876=CARTESIAN_POINT('Ctrl Pts',(-0.219017458803409,0.0917079433893473,
-0.401825180362117));
#72877=CARTESIAN_POINT('Ctrl Pts',(-0.223127630984375,0.0811978604855395,
-0.401136796826917));
#72878=CARTESIAN_POINT('Ctrl Pts',(-0.230148509132521,0.0586229852930964,
-0.399687854717072));
#72879=CARTESIAN_POINT('Ctrl Pts',(-0.232892040678517,0.046543019007061,
-0.398928593311946));
#72880=CARTESIAN_POINT('Ctrl Pts',(-0.235454519399103,0.0290129582105658,
-0.397802477268319));
#72881=CARTESIAN_POINT('Ctrl Pts',(-0.236048799425014,0.0236968321811222,
-0.397458039662757));
#72882=CARTESIAN_POINT('Ctrl Pts',(-0.23660689132188,0.0165111704860901,
-0.396986274539072));
#72883=CARTESIAN_POINT('Ctrl Pts',(-0.236729089594629,0.0146552920532204,
-0.396863880091339));
#72884=CARTESIAN_POINT('Ctrl Pts',(-0.236896966262464,0.0115487533799083,
-0.396657999017235));
#72885=CARTESIAN_POINT('Ctrl Pts',(-0.236954596731431,0.0102988016100876,
-0.396574888504609));
#72886=CARTESIAN_POINT('Ctrl Pts',(-0.237044835434167,0.00793522221117625,
-0.39641719225462));
#72887=CARTESIAN_POINT('Ctrl Pts',(-0.237079493106086,0.00682170308155223,
-0.396342672917639));
#72888=CARTESIAN_POINT('Ctrl Pts',(-0.237130791666075,0.00469079598739136,
-0.396199618979042));
#72889=CARTESIAN_POINT('Ctrl Pts',(-0.237148732963697,0.00367346167808046,
-0.396131126857865));
#72890=CARTESIAN_POINT('Ctrl Pts',(-0.237170272980592,0.00175014714279538,
-0.396001259635131));
#72891=CARTESIAN_POINT('Ctrl Pts',(-0.237175227796383,0.000844199745607207,
-0.395939928391633));
#72892=CARTESIAN_POINT('Ctrl Pts',(-0.237174991963874,-6.17408820430942E-5,
-0.395878435029662));
#72893=CARTESIAN_POINT('Ctrl Pts',(-0.236793760552407,-4.73610052024943E-5,
-0.395658945585743));
#72894=CARTESIAN_POINT('Ctrl Pts',(-0.236858273123243,-0.036785166275623,
-0.393202937948888));
#72895=CARTESIAN_POINT('Ctrl Pts',(-0.211519713818698,-0.152637591068471,
-0.385452286954036));
#72896=CARTESIAN_POINT('Ctrl Pts',(-0.0307313623949624,-0.278681719209718,
-0.372406992601189));
#72897=CARTESIAN_POINT('Ctrl Pts',(0.217548020283183,-0.176863722360531,
-0.3565230625272));
#72898=CARTESIAN_POINT('Ctrl Pts',(0.266540396953676,0.086972027342936,
-0.340639132453212));
#72899=CARTESIAN_POINT('Ctrl Pts',(0.108036699394564,0.236534038370805,
-0.327739595357166));
#72900=CARTESIAN_POINT('Ctrl Pts',(-0.00788774517042406,0.239305024134992,
-0.320134701619114));
#72901=CARTESIAN_POINT('Ctrl Pts',(-0.0418736008932845,0.233079825957759,
-0.317824451239062));
#72902=CARTESIAN_POINT('Origin',(0.,0.,-2.1456589891905));
#72903=CARTESIAN_POINT('',(-0.0419392735105505,0.233437524752143,-0.198319131484844));
#72904=CARTESIAN_POINT('',(-0.0419392741328085,0.233437524640348,-0.217838756538471));
#72905=CARTESIAN_POINT('',(-0.0419392741328076,0.233437524640348,-2.1456589891905));
#72906=CARTESIAN_POINT('',(-0.237378208863769,0.000179012329966397,-0.275941010809497));
#72907=CARTESIAN_POINT('Ctrl Pts',(-0.0419392735105505,0.233437524752143,
-0.198319131484844));
#72908=CARTESIAN_POINT('Ctrl Pts',(-0.0408906519443126,0.233625919598782,
-0.198393501506002));
#72909=CARTESIAN_POINT('Ctrl Pts',(-0.0398406677809363,0.233807265436557,
-0.198467570847434));
#72910=CARTESIAN_POINT('Ctrl Pts',(-0.0374695049912287,0.234200356104447,
-0.198633892873104));
#72911=CARTESIAN_POINT('Ctrl Pts',(-0.0361477522691964,0.234408000749219,
-0.198725944022587));
#72912=CARTESIAN_POINT('Ctrl Pts',(-0.0340003552892332,0.234726756608232,
-0.198874348178815));
#72913=CARTESIAN_POINT('Ctrl Pts',(-0.0331757802923443,0.234844719086903,
-0.198931059852335));
#72914=CARTESIAN_POINT('Ctrl Pts',(-0.0317010447894705,0.235047770219734,
-0.199031978163518));
#72915=CARTESIAN_POINT('Ctrl Pts',(-0.0310511370933753,0.235134509259918,
-0.19907627447507));
#72916=CARTESIAN_POINT('Ctrl Pts',(-0.0296223739676866,0.235319169930043,
-0.199173264260355));
#72917=CARTESIAN_POINT('Ctrl Pts',(-0.0288433872861542,0.2354159209371,
-0.199225892132143));
#72918=CARTESIAN_POINT('Ctrl Pts',(-0.0265902388878308,0.235684412714702,
-0.199377421091112));
#72919=CARTESIAN_POINT('Ctrl Pts',(-0.0251148948729674,0.235846190417251,
-0.199475785416768));
#72920=CARTESIAN_POINT('Ctrl Pts',(-0.0123063785541186,0.237129140955931,
-0.200323103571914));
#72921=CARTESIAN_POINT('Ctrl Pts',(-0.000905972739818323,0.237446684457663,
-0.201032502145055));
#72922=CARTESIAN_POINT('Ctrl Pts',(0.0295443988519499,0.236100574073751,
-0.202909331837398));
#72923=CARTESIAN_POINT('Ctrl Pts',(0.048440995153022,0.232958724438614,
-0.204060836371404));
#72924=CARTESIAN_POINT('Ctrl Pts',(0.0703384475933215,0.226535688858469,
-0.20552794567744));
#72925=CARTESIAN_POINT('Ctrl Pts',(0.0738950040511176,0.225400624303204,
-0.205770343728593));
#72926=CARTESIAN_POINT('Ctrl Pts',(0.0788299145653848,0.22369631253669,
-0.206113198361948));
#72927=CARTESIAN_POINT('Ctrl Pts',(0.0802320547282062,0.223197251099559,
-0.206211357300669));
#72928=CARTESIAN_POINT('Ctrl Pts',(0.0826593353134839,0.222307485849543,
-0.20638262590514));
#72929=CARTESIAN_POINT('Ctrl Pts',(0.0836866449615448,0.221922800462884,
-0.206455534206672));
#72930=CARTESIAN_POINT('Ctrl Pts',(0.0858270451439506,0.22110433291032,
-0.206608340352562));
#72931=CARTESIAN_POINT('Ctrl Pts',(0.0869395982322922,0.220669240898619,
-0.2066882803394));
#72932=CARTESIAN_POINT('Ctrl Pts',(0.089578173805124,0.219614307988721,
-0.206879117937247));
#72933=CARTESIAN_POINT('Ctrl Pts',(0.0911011023744059,0.218986945736783,
-0.206990266462376));
#72934=CARTESIAN_POINT('Ctrl Pts',(0.0962753840534234,0.216792112460512,
-0.207371407883418));
#72935=CARTESIAN_POINT('Ctrl Pts',(0.0998936502034588,0.215148843663351,
-0.207643949904716));
#72936=CARTESIAN_POINT('Ctrl Pts',(0.108586211261025,0.210934490776281,
-0.208313891516673));
#72937=CARTESIAN_POINT('Ctrl Pts',(0.113612396482174,0.208270351323096,
-0.208714248660186));
#72938=CARTESIAN_POINT('Ctrl Pts',(0.137763556271179,0.194334484591581,
-0.210701628754575));
#72939=CARTESIAN_POINT('Ctrl Pts',(0.155334491883245,0.18059829748691,-0.21236254026382));
#72940=CARTESIAN_POINT('Ctrl Pts',(0.172900510626221,0.16237946676154,-0.21414609014474));
#72941=CARTESIAN_POINT('Ctrl Pts',(0.175017704239143,0.16009523201039,-0.214363227042695));
#72942=CARTESIAN_POINT('Ctrl Pts',(0.177811975682375,0.156958790154907,
-0.214652019838792));
#72943=CARTESIAN_POINT('Ctrl Pts',(0.178528972667212,0.156142776125272,
-0.214726326617835));
#72944=CARTESIAN_POINT('Ctrl Pts',(0.179652342302017,0.154846415190829,
-0.214843033014999));
#72945=CARTESIAN_POINT('Ctrl Pts',(0.180062442168332,0.154369340660612,
-0.214885699062894));
#72946=CARTESIAN_POINT('Ctrl Pts',(0.180906737906747,0.153379218042015,
-0.214973654470858));
#72947=CARTESIAN_POINT('Ctrl Pts',(0.181340656304526,0.152865950199629,
-0.215018921401336));
#72948=CARTESIAN_POINT('Ctrl Pts',(0.182387336131514,0.151617138601297,
-0.215128283732326));
#72949=CARTESIAN_POINT('Ctrl Pts',(0.182997846070875,0.150879705431736,
-0.215192217481971));
#72950=CARTESIAN_POINT('Ctrl Pts',(0.185148164527114,0.148250089331276,
-0.215418003435874));
#72951=CARTESIAN_POINT('Ctrl Pts',(0.186663288011938,0.146337793715882,
-0.215578200461039));
#72952=CARTESIAN_POINT('Ctrl Pts',(0.190375847449172,0.14150052366493,-0.215974530621141));
#72953=CARTESIAN_POINT('Ctrl Pts',(0.192535681095711,0.138547378018361,
-0.216208584079583));
#72954=CARTESIAN_POINT('Ctrl Pts',(0.208412292795654,0.115750507007908,
-0.217966155721346));
#72955=CARTESIAN_POINT('Ctrl Pts',(0.219098122065027,0.093968359373036,
-0.219383456521826));
#72956=CARTESIAN_POINT('Ctrl Pts',(0.227712964072919,0.0664877947031829,
-0.221222284110396));
#72957=CARTESIAN_POINT('Ctrl Pts',(0.228978734388096,0.0619883484522639,
-0.22152425417164));
#72958=CARTESIAN_POINT('Ctrl Pts',(0.230547735911851,0.0557043685174594,
-0.22194871340123));
#72959=CARTESIAN_POINT('Ctrl Pts',(0.230964763746884,0.0539491688019627,
-0.222067557427068));
#72960=CARTESIAN_POINT('Ctrl Pts',(0.231604332458714,0.0511138870388545,
-0.222260070633318));
#72961=CARTESIAN_POINT('Ctrl Pts',(0.231839439966796,0.0500366892163563,
-0.222333335500144));
#72962=CARTESIAN_POINT('Ctrl Pts',(0.232312822599627,0.0477927922263265,
-0.222486229520478));
#72963=CARTESIAN_POINT('Ctrl Pts',(0.232549838588974,0.0466258620923692,
-0.222565896559128));
#72964=CARTESIAN_POINT('Ctrl Pts',(0.233089278674585,0.0438634884240857,
-0.222754875469015));
#72965=CARTESIAN_POINT('Ctrl Pts',(0.233384121295515,0.0422666434468315,
-0.222864425064524));
#72966=CARTESIAN_POINT('Ctrl Pts',(0.23431914321321,0.0368942293103895,
-0.223234090724907));
#72967=CARTESIAN_POINT('Ctrl Pts',(0.234884246888271,0.033106383409515,
-0.223496551858554));
#72968=CARTESIAN_POINT('Ctrl Pts',(0.237086903605599,0.0154172038502997,
-0.224731413607685));
#72969=CARTESIAN_POINT('Ctrl Pts',(0.237583260247537,0.00140402554505526,
-0.225738242708841));
#72970=CARTESIAN_POINT('Ctrl Pts',(0.236011994139174,-0.0282037735747135,
-0.227899908143103));
#72971=CARTESIAN_POINT('Ctrl Pts',(0.233636114644562,-0.0437190768782639,
-0.229053052127985));
#72972=CARTESIAN_POINT('Ctrl Pts',(0.22925320235401,-0.0608187706105084,
-0.230282619571909));
#72973=CARTESIAN_POINT('Ctrl Pts',(0.228733960281828,-0.062743363942219,
-0.230420356199139));
#72974=CARTESIAN_POINT('Ctrl Pts',(0.227952183963314,-0.0655022635516871,
-0.230616638709787));
#72975=CARTESIAN_POINT('Ctrl Pts',(0.22770922049643,-0.0663419600718826,
-0.230676223086176));
#72976=CARTESIAN_POINT('Ctrl Pts',(0.227274304100026,-0.0678145163145308,
-0.230780417146112));
#72977=CARTESIAN_POINT('Ctrl Pts',(0.22708433872812,-0.0684479442741014,
-0.230825138860422));
#72978=CARTESIAN_POINT('Ctrl Pts',(0.22667392167327,-0.0697959383767032,
-0.230920095263616));
#72979=CARTESIAN_POINT('Ctrl Pts',(0.22645273827191,-0.0705102627194792,
-0.230970287213825));
#72980=CARTESIAN_POINT('Ctrl Pts',(0.225834787739539,-0.0724730662974802,
-0.231107884305723));
#72981=CARTESIAN_POINT('Ctrl Pts',(0.225431042509389,-0.0737193458962792,
-0.23119489495115));
#72982=CARTESIAN_POINT('Ctrl Pts',(0.223082868363784,-0.0807679476473073,
-0.231685317642865));
#72983=CARTESIAN_POINT('Ctrl Pts',(0.220924596420078,-0.0864971953561818,
-0.232077461834929));
#72984=CARTESIAN_POINT('Ctrl Pts',(0.212040151735574,-0.107570886020958,
-0.233517943615066));
#72985=CARTESIAN_POINT('Ctrl Pts',(0.203916569277001,-0.122272738137984,
-0.234522017734836));
#72986=CARTESIAN_POINT('Ctrl Pts',(0.188434147729298,-0.144393928146496,
-0.23619724329017));
#72987=CARTESIAN_POINT('Ctrl Pts',(0.18201955647348,-0.152400382984631,
-0.236843800015503));
#72988=CARTESIAN_POINT('Ctrl Pts',(0.173559932183318,-0.161660748833739,
-0.237660872086531));
#72989=CARTESIAN_POINT('Ctrl Pts',(0.171987549801099,-0.163332574466902,
-0.237811353683865));
#72990=CARTESIAN_POINT('Ctrl Pts',(0.169456642744818,-0.165946472877133,
-0.238051571146007));
#72991=CARTESIAN_POINT('Ctrl Pts',(0.168513919737545,-0.166903697860553,
-0.238140622580898));
#72992=CARTESIAN_POINT('Ctrl Pts',(0.166737020919909,-0.168677529749143,
-0.238307715990569));
#72993=CARTESIAN_POINT('Ctrl Pts',(0.165904846725866,-0.169496091212868,
-0.238385667980301));
#72994=CARTESIAN_POINT('Ctrl Pts',(0.164031656499945,-0.171311628022471,
-0.238560485292351));
#72995=CARTESIAN_POINT('Ctrl Pts',(0.162987533467228,-0.172305316239645,
-0.238657489243466));
#72996=CARTESIAN_POINT('Ctrl Pts',(0.159868385752157,-0.175220078545677,
-0.238946027794434));
#72997=CARTESIAN_POINT('Ctrl Pts',(0.157768053294167,-0.177113570464016,
-0.239138719367062));
#72998=CARTESIAN_POINT('Ctrl Pts',(0.147992014620262,-0.185614978290297,
-0.240028755909638));
#72999=CARTESIAN_POINT('Ctrl Pts',(0.1399327717453,-0.191763726430454,-0.240744257494194));
#73000=CARTESIAN_POINT('Ctrl Pts',(0.120110858059246,-0.204970391008402,
-0.242459265759643));
#73001=CARTESIAN_POINT('Ctrl Pts',(0.108079532206323,-0.211561490916474,
-0.243467770606852));
#73002=CARTESIAN_POINT('Ctrl Pts',(0.0880773396988655,-0.220365566623388,
-0.24505117752501));
#73003=CARTESIAN_POINT('Ctrl Pts',(0.0804412308386572,-0.223266295351193,
-0.245635194754938));
#73004=CARTESIAN_POINT('Ctrl Pts',(0.0714131627912768,-0.226172244112975,
-0.246291307043648));
#73005=CARTESIAN_POINT('Ctrl Pts',(0.0701529690250268,-0.2265662926427,
-0.246382126756864));
#73006=CARTESIAN_POINT('Ctrl Pts',(0.0680974913850215,-0.227190222925519,
-0.246528947435672));
#73007=CARTESIAN_POINT('Ctrl Pts',(0.0673041993674203,-0.227426494775398,
-0.246585294980196));
#73008=CARTESIAN_POINT('Ctrl Pts',(0.0658805072608992,-0.227842421469994,
-0.246685833461541));
#73009=CARTESIAN_POINT('Ctrl Pts',(0.0652505854859661,-0.228023620233389,
-0.246730111046778));
#73010=CARTESIAN_POINT('Ctrl Pts',(0.0638603168994318,-0.228417301824784,
-0.246827379129658));
#73011=CARTESIAN_POINT('Ctrl Pts',(0.063099655717341,-0.228628601319358,
-0.246880301429568));
#73012=CARTESIAN_POINT('Ctrl Pts',(0.0608854961345036,-0.229231767276363,
-0.247033527987953));
#73013=CARTESIAN_POINT('Ctrl Pts',(0.0594292719137986,-0.229613607387583,
-0.247133276936913));
#73014=CARTESIAN_POINT('Ctrl Pts',(0.0446346667033431,-0.233342755548294,
-0.24813723621359));
#73015=CARTESIAN_POINT('Ctrl Pts',(0.0310306665192168,-0.235538335204974,
-0.248983660376269));
#73016=CARTESIAN_POINT('Ctrl Pts',(-0.000352386463949084,-0.237835097405011,
-0.250913660966725));
#73017=CARTESIAN_POINT('Ctrl Pts',(-0.0181031180450091,-0.237145208320164,
-0.251992654571631));
#73018=CARTESIAN_POINT('Ctrl Pts',(-0.0386961959379133,-0.234017784850299,
-0.253339363571248));
#73019=CARTESIAN_POINT('Ctrl Pts',(-0.0417718169183226,-0.233488400218571,
-0.253542869799111));
#73020=CARTESIAN_POINT('Ctrl Pts',(-0.0463073460652319,-0.232615251997926,
-0.253846918526893));
#73021=CARTESIAN_POINT('Ctrl Pts',(-0.0477759604003386,-0.23231806472192,
-0.253945985761868));
#73022=CARTESIAN_POINT('Ctrl Pts',(-0.0503885426558618,-0.231763564979018,
-0.254123365508268));
#73023=CARTESIAN_POINT('Ctrl Pts',(-0.0515336141072254,-0.231511645096038,
-0.254201503408333));
#73024=CARTESIAN_POINT('Ctrl Pts',(-0.0539505652592379,-0.230961087467525,
-0.254367288842436));
#73025=CARTESIAN_POINT('Ctrl Pts',(-0.0552219354157915,-0.230660410877781,
-0.254454999528943));
#73026=CARTESIAN_POINT('Ctrl Pts',(-0.0586126931778994,-0.229828863144447,
-0.254690306866756));
#73027=CARTESIAN_POINT('Ctrl Pts',(-0.0607272951177369,-0.229279194882732,
-0.254838503549516));
#73028=CARTESIAN_POINT('Ctrl Pts',(-0.071629987061836,-0.226283751568062,
-0.25561034665026));
#73029=CARTESIAN_POINT('Ctrl Pts',(-0.0802781627260963,-0.223361971272003,
-0.256249242590259));
#73030=CARTESIAN_POINT('Ctrl Pts',(-0.09877060054596,-0.215901452667303,
-0.257673979071009));
#73031=CARTESIAN_POINT('Ctrl Pts',(-0.108515986908028,-0.211171300074533,
-0.258463592668211));
#73032=CARTESIAN_POINT('Ctrl Pts',(-0.128441729312765,-0.199755361036593,
-0.260140711265932));
#73033=CARTESIAN_POINT('Ctrl Pts',(-0.138501535037477,-0.192916732527656,
-0.261026027896984));
#73034=CARTESIAN_POINT('Ctrl Pts',(-0.149613458168704,-0.184043714414448,
-0.262017946315261));
#73035=CARTESIAN_POINT('Ctrl Pts',(-0.15121599525498,-0.182729305778164,
-0.262161340208199));
#73036=CARTESIAN_POINT('Ctrl Pts',(-0.153438505119097,-0.180857126524833,
-0.262360452283735));
#73037=CARTESIAN_POINT('Ctrl Pts',(-0.154073024968241,-0.18031688245355,
-0.262417326486901));
#73038=CARTESIAN_POINT('Ctrl Pts',(-0.155214106493161,-0.179334919751906,
-0.262519636310813));
#73039=CARTESIAN_POINT('Ctrl Pts',(-0.155721662199803,-0.178894371793139,
-0.262565154993845));
#73040=CARTESIAN_POINT('Ctrl Pts',(-0.156746873733782,-0.177996839768093,
-0.262657108873602));
#73041=CARTESIAN_POINT('Ctrl Pts',(-0.157264416946585,-0.177539743680831,
-0.262703535262519));
#73042=CARTESIAN_POINT('Ctrl Pts',(-0.158542445501955,-0.176401010562457,
-0.262818219573316));
#73043=CARTESIAN_POINT('Ctrl Pts',(-0.159300547407176,-0.17571670166335,
-0.262886282046332));
#73044=CARTESIAN_POINT('Ctrl Pts',(-0.162356336224479,-0.172922329931214,
-0.26316088556557));
#73045=CARTESIAN_POINT('Ctrl Pts',(-0.164616828546704,-0.170771818953241,
-0.263364610678865));
#73046=CARTESIAN_POINT('Ctrl Pts',(-0.1705318051301,-0.164917994784074,
-0.263901461125042));
#73047=CARTESIAN_POINT('Ctrl Pts',(-0.174108111644666,-0.16113787333786,
-0.264230066746408));
#73048=CARTESIAN_POINT('Ctrl Pts',(-0.185178561386462,-0.148637214531152,
-0.26527232113807));
#73049=CARTESIAN_POINT('Ctrl Pts',(-0.192164247961001,-0.139488506833902,
-0.265970144835793));
#73050=CARTESIAN_POINT('Ctrl Pts',(-0.205900771978131,-0.118497051428662,
-0.26751258562063));
#73051=CARTESIAN_POINT('Ctrl Pts',(-0.212350238620743,-0.10650813398858,
-0.268358706109745));
#73052=CARTESIAN_POINT('Ctrl Pts',(-0.218688355073152,-0.0918321107238223,
-0.26939897385841));
#73053=CARTESIAN_POINT('Ctrl Pts',(-0.219605797813507,-0.0896159923442804,
-0.269556109723826));
#73054=CARTESIAN_POINT('Ctrl Pts',(-0.220993037739358,-0.0861157709838005,
-0.269804568529628));
#73055=CARTESIAN_POINT('Ctrl Pts',(-0.221485625389237,-0.0848408295278547,
-0.269895124200468));
#73056=CARTESIAN_POINT('Ctrl Pts',(-0.222373976181857,-0.0824810804611815,
-0.270062867421355));
#73057=CARTESIAN_POINT('Ctrl Pts',(-0.222772891684219,-0.0813974972983083,
-0.270139946763227));
#73058=CARTESIAN_POINT('Ctrl Pts',(-0.223640514567448,-0.0789865954731762,
-0.270311581284186));
#73059=CARTESIAN_POINT('Ctrl Pts',(-0.224105346713349,-0.0776579387204261,
-0.270406261968071));
#73060=CARTESIAN_POINT('Ctrl Pts',(-0.225414692289538,-0.0738056821353131,
-0.270681084056492));
#73061=CARTESIAN_POINT('Ctrl Pts',(-0.226228571654414,-0.0712719760977893,
-0.270862222809807));
#73062=CARTESIAN_POINT('Ctrl Pts',(-0.227974805574555,-0.065504158222808,
-0.271275591665741));
#73063=CARTESIAN_POINT('Ctrl Pts',(-0.228881277717332,-0.062262873832811,
-0.271508607248377));
#73064=CARTESIAN_POINT('Ctrl Pts',(-0.234684897256532,-0.039667644587641,
-0.273138252610976));
#73065=CARTESIAN_POINT('Ctrl Pts',(-0.237189270172021,-0.0197850128759254,
-0.274608699299126));
#73066=CARTESIAN_POINT('Ctrl Pts',(-0.23717493883632,0.000170331993290248,
-0.27605765282612));
#73067=CARTESIAN_POINT('Ctrl Pts',(-0.0419325474085123,0.233395695413122,
-0.298126337027087));
#73068=CARTESIAN_POINT('Ctrl Pts',(-0.061445870050903,0.230090132428982,
-0.296798518412659));
#73069=CARTESIAN_POINT('Ctrl Pts',(-0.156420177455278,0.201614181129484,
-0.290176056440238));
#73070=CARTESIAN_POINT('Ctrl Pts',(-0.23149538472674,0.101752851827335,
-0.282780947701042));
#73071=CARTESIAN_POINT('Ctrl Pts',(-0.23747464009092,0.0116642938095829,
-0.276713657576272));
#73072=CARTESIAN_POINT('Ctrl Pts',(-0.237378208863769,0.000179012329966397,
-0.275941010809497));
#73073=CARTESIAN_POINT('',(-0.237174920140862,-0.000194630870780877,-0.2956589891905));
#73074=CARTESIAN_POINT('Ctrl Pts',(-0.0418736008932845,0.233079825957759,
-0.317824451239062));
#73075=CARTESIAN_POINT('Ctrl Pts',(-0.0857766990355478,0.22503808386485,
-0.314840058261121));
#73076=CARTESIAN_POINT('Ctrl Pts',(-0.189385050560669,0.175933016957098,
-0.307451603093063));
#73077=CARTESIAN_POINT('Ctrl Pts',(-0.236747464188876,0.0653079928409343,
-0.300063147925004));
#73078=CARTESIAN_POINT('Ctrl Pts',(-0.237328574752462,-0.000193321075562004,
-0.295659085734888));
#73079=CARTESIAN_POINT('Ctrl Pts',(-0.237174920140862,-0.000194630870780877,
-0.2956589891905));
#73080=CARTESIAN_POINT('Ctrl Pts',(-0.237164058071819,-0.013431022135193,
-0.294768440204083));
#73081=CARTESIAN_POINT('Ctrl Pts',(-0.236044766251475,-0.0266231619079329,
-0.293877891217663));
#73082=CARTESIAN_POINT('Ctrl Pts',(-0.233841221537961,-0.0396265534034244,
-0.292987342231242));
#73083=CARTESIAN_POINT('Ctrl Pts',(-0.231495933747312,-0.0534663884312158,
-0.292039508655633));
#73084=CARTESIAN_POINT('Ctrl Pts',(-0.227909804592804,-0.0671440084078081,
-0.291091675080023));
#73085=CARTESIAN_POINT('Ctrl Pts',(-0.223123839459559,-0.0804222163946304,
-0.290143841504413));
#73086=CARTESIAN_POINT('Ctrl Pts',(-0.218347568795678,-0.0936735279923352,
-0.289197927864136));
#73087=CARTESIAN_POINT('Ctrl Pts',(-0.212376499564324,-0.106526232553001,
-0.288252014223859));
#73088=CARTESIAN_POINT('Ctrl Pts',(-0.20530180552342,-0.118756680965005,
-0.287306100583582));
#73089=CARTESIAN_POINT('Ctrl Pts',(-0.198228244350353,-0.130985170920353,
-0.286360338412066));
#73090=CARTESIAN_POINT('Ctrl Pts',(-0.19005178309994,-0.142590856550964,
-0.28541457624055));
#73091=CARTESIAN_POINT('Ctrl Pts',(-0.180909866664417,-0.153374055069503,
-0.284468814069034));
#73092=CARTESIAN_POINT('Ctrl Pts',(-0.171769479814827,-0.164155449389886,
-0.283523210138355));
#73093=CARTESIAN_POINT('Ctrl Pts',(-0.161664512499544,-0.174114004722382,
-0.282577606207676));
#73094=CARTESIAN_POINT('Ctrl Pts',(-0.15077169015199,-0.183084346883376,
-0.281632002276998));
#73095=CARTESIAN_POINT('Ctrl Pts',(-0.139853365450954,-0.192075690473508,
-0.280684184491643));
#73096=CARTESIAN_POINT('Ctrl Pts',(-0.128144177315514,-0.200073704553567,
-0.279736366706287));
#73097=CARTESIAN_POINT('Ctrl Pts',(-0.115852324306153,-0.206954631689803,
-0.278788548920932));
#73098=CARTESIAN_POINT('Ctrl Pts',(-0.108567712671679,-0.211032526359908,
-0.278226836666376));
#73099=CARTESIAN_POINT('Ctrl Pts',(-0.101078986156344,-0.214718936239686,
-0.27766512441182));
#73100=CARTESIAN_POINT('Ctrl Pts',(-0.0934328807077565,-0.217996049110185,
-0.277103412157264));
#73101=CARTESIAN_POINT('Ctrl Pts',(-0.0805308487538358,-0.223525846633392,
-0.276155579367627));
#73102=CARTESIAN_POINT('Ctrl Pts',(-0.0670926434824372,-0.227924930145413,
-0.275207746577991));
#73103=CARTESIAN_POINT('Ctrl Pts',(-0.0533398279857906,-0.231099206782382,
-0.274259913788354));
#73104=CARTESIAN_POINT('Ctrl Pts',(-0.0396148702701166,-0.234267053586615,
-0.273314000934184));
#73105=CARTESIAN_POINT('Ctrl Pts',(-0.0255773559771039,-0.236214763200705,
-0.272368088080015));
#73106=CARTESIAN_POINT('Ctrl Pts',(-0.0114646524321514,-0.23689774665372,
-0.271422175225845));
#73107=CARTESIAN_POINT('Ctrl Pts',(0.00264579141979539,-0.237580620749025,
-0.270476413829025));
#73108=CARTESIAN_POINT('Ctrl Pts',(0.0168305710547536,-0.236999080620268,
-0.269530652432204));
#73109=CARTESIAN_POINT('Ctrl Pts',(0.0308473827951734,-0.235160412484091,
-0.268584891035384));
#73110=CARTESIAN_POINT('Ctrl Pts',(0.0448618493803064,-0.233322051975811,
-0.267639287874072));
#73111=CARTESIAN_POINT('Ctrl Pts',(0.0587075782799197,-0.230227107852141,
-0.26669368471276));
#73112=CARTESIAN_POINT('Ctrl Pts',(0.0721498098128534,-0.225934471847412,
-0.265748081551449));
#73113=CARTESIAN_POINT('Ctrl Pts',(0.0856235127516525,-0.221631785778481,
-0.264800264512121));
#73114=CARTESIAN_POINT('Ctrl Pts',(0.0986910490096823,-0.21612610661674,
-0.263852447472793));
#73115=CARTESIAN_POINT('Ctrl Pts',(0.111135576046833,-0.209525331074166,
-0.262904630433465));
#73116=CARTESIAN_POINT('Ctrl Pts',(0.118510724532073,-0.205613434736209,
-0.262342914316732));
#73117=CARTESIAN_POINT('Ctrl Pts',(0.125667491310397,-0.201317822332404,
-0.2617811982));
#73118=CARTESIAN_POINT('Ctrl Pts',(0.132565576710731,-0.196668117640738,
-0.261219482083267));
#73119=CARTESIAN_POINT('Ctrl Pts',(0.144205329226883,-0.188822257703783,
-0.260271648560825));
#73120=CARTESIAN_POINT('Ctrl Pts',(0.155185420939559,-0.179912984470352,
-0.259323815038384));
#73121=CARTESIAN_POINT('Ctrl Pts',(0.16530669567106,-0.170075503795566,
-0.258375981515942));
#73122=CARTESIAN_POINT('Ctrl Pts',(0.17540746861187,-0.160257950054399,
-0.257430067937875));
#73123=CARTESIAN_POINT('Ctrl Pts',(0.184652235968526,-0.149516445600452,
-0.256484154359809));
#73124=CARTESIAN_POINT('Ctrl Pts',(0.192874879116141,-0.138026307749407,
-0.255538240781742));
#73125=CARTESIAN_POINT('Ctrl Pts',(0.201096205468579,-0.126538009958528,
-0.254592478684703));
#73126=CARTESIAN_POINT('Ctrl Pts',(0.208295207260659,-0.114301965120842,
-0.253646716587665));
#73127=CARTESIAN_POINT('Ctrl Pts',(0.214346686308301,-0.101525753844288,
-0.252700954490626));
#73128=CARTESIAN_POINT('Ctrl Pts',(0.220397152803617,-0.0887516803232042,
-0.251755350641448));
#73129=CARTESIAN_POINT('Ctrl Pts',(0.225300136886879,-0.0754383823506948,
-0.25080974679227));
#73130=CARTESIAN_POINT('Ctrl Pts',(0.228977898146495,-0.0618150692421615,
-0.249864142943091));
#73131=CARTESIAN_POINT('Ctrl Pts',(0.232664269772247,-0.0481598612645623,
-0.248916325248373));
#73132=CARTESIAN_POINT('Ctrl Pts',(0.235119516839297,-0.0341940083580267,
-0.247968507553655));
#73133=CARTESIAN_POINT('Ctrl Pts',(0.236316793157245,-0.0201582215702607,
-0.247020689858938));
#73134=CARTESIAN_POINT('Ctrl Pts',(0.237026344389551,-0.0118400834242511,
-0.246458977242387));
#73135=CARTESIAN_POINT('Ctrl Pts',(0.237295070610515,-0.00349751050045388,
-0.245897264625838));
#73136=CARTESIAN_POINT('Ctrl Pts',(0.237126026238738,0.0048195752121259,
-0.245335552009287));
#73137=CARTESIAN_POINT('Ctrl Pts',(0.236840780463713,0.0188538405064866,
-0.244387717136319));
#73138=CARTESIAN_POINT('Ctrl Pts',(0.235304324253603,0.0329100654086107,
-0.24343988226335));
#73139=CARTESIAN_POINT('Ctrl Pts',(0.232522348153217,0.046747601374982,
-0.242492047390382));
#73140=CARTESIAN_POINT('Ctrl Pts',(0.22974600719756,0.0605571081581194,
-0.241546132442853));
#73141=CARTESIAN_POINT('Ctrl Pts',(0.225729247348527,0.0741479816775976,
-0.240600217495324));
#73142=CARTESIAN_POINT('Ctrl Pts',(0.220529374087023,0.0872855989827991,
-0.239654302547795));
#73143=CARTESIAN_POINT('Ctrl Pts',(0.215330333504744,0.100421112501918,
-0.238708539073906));
#73144=CARTESIAN_POINT('Ctrl Pts',(0.208948815794916,0.113102721053147,
-0.237762775600016));
#73145=CARTESIAN_POINT('Ctrl Pts',(0.201491418064631,0.12511270547512,-0.236817012126127));
#73146=CARTESIAN_POINT('Ctrl Pts',(0.194035268079209,0.137120680429863,
-0.235871406893967));
#73147=CARTESIAN_POINT('Ctrl Pts',(0.185504051561946,0.148456554616219,
-0.234925801661806));
#73148=CARTESIAN_POINT('Ctrl Pts',(0.176048263005386,0.158930770204472,
-0.233980196429646));
#73149=CARTESIAN_POINT('Ctrl Pts',(0.166570336790122,0.169429507767649,
-0.233032377369864));
#73150=CARTESIAN_POINT('Ctrl Pts',(0.15616411072589,0.179061968283412,-0.232084558310081));
#73151=CARTESIAN_POINT('Ctrl Pts',(0.145017328464764,0.187675131730186,
-0.231136739250299));
#73152=CARTESIAN_POINT('Ctrl Pts',(0.138411413689159,0.192779548623317,
-0.23057503347863));
#73153=CARTESIAN_POINT('Ctrl Pts',(0.131546056594898,0.197526748657646,
-0.23001332770696));
#73154=CARTESIAN_POINT('Ctrl Pts',(0.124464865211157,0.201892243419524,
-0.229451621935291));
#73155=CARTESIAN_POINT('Ctrl Pts',(0.112264984280593,0.209413367113511,
-0.228483883152223));
#73156=CARTESIAN_POINT('Ctrl Pts',(0.0993388589516617,0.215850597682492,
-0.227516144369154));
#73157=CARTESIAN_POINT('Ctrl Pts',(0.0859053425306205,0.221070696270891,
-0.226548405586086));
#73158=CARTESIAN_POINT('Ctrl Pts',(0.0727733693233782,0.226173618890218,
-0.225602389712613));
#73159=CARTESIAN_POINT('Ctrl Pts',(0.0591573674941752,0.230113191175845,
-0.22465637383914));
#73160=CARTESIAN_POINT('Ctrl Pts',(0.0452860359781853,0.232811416323132,
-0.223710357965667));
#73161=CARTESIAN_POINT('Ctrl Pts',(0.0309369233451853,0.235602578548833,
-0.222731757727801));
#73162=CARTESIAN_POINT('Ctrl Pts',(0.016315423833323,0.237064855767117,
-0.221753157489935));
#73163=CARTESIAN_POINT('Ctrl Pts',(0.00168848205185222,0.237168989653708,
-0.220774557252068));
#73164=CARTESIAN_POINT('Ctrl Pts',(-0.0129384597296185,0.237273123540299,
-0.219795957014202));
#73165=CARTESIAN_POINT('Ctrl Pts',(-0.0275698529512033,0.236019127983656,
-0.218817356776337));
#73166=CARTESIAN_POINT('Ctrl Pts',(-0.0419392741328085,0.233437524640348,
-0.217838756538471));
#73167=CARTESIAN_POINT('Origin',(0.,0.,-2.1456589891905));
#73168=CARTESIAN_POINT('',(-0.0419392282806928,0.233437532878113,-0.0979609479953583));
#73169=CARTESIAN_POINT('',(-0.0419392741328228,0.233437524640346,-0.117607182502807));
#73170=CARTESIAN_POINT('',(-0.0419392741328076,0.233437524640348,-2.1456589891905));
#73171=CARTESIAN_POINT('Ctrl Pts',(-0.0419392282806931,0.233437532878113,
-0.0979609479953583));
#73172=CARTESIAN_POINT('Ctrl Pts',(-0.0317635392632918,0.235265690241466,
-0.0986991702520308));
#73173=CARTESIAN_POINT('Ctrl Pts',(-0.0214726811650525,0.23642772405573,
-0.0994531880114252));
#73174=CARTESIAN_POINT('Ctrl Pts',(-0.00136646084210373,0.237372473734899,
-0.100924066052501));
#73175=CARTESIAN_POINT('Ctrl Pts',(0.00841873030292184,0.237227116043163,
-0.101638678885694));
#73176=CARTESIAN_POINT('Ctrl Pts',(0.0213076755559574,0.236236920560851,
-0.102560202574135));
#73177=CARTESIAN_POINT('Ctrl Pts',(0.0244429230897771,0.235933137185549,
-0.102782765074389));
#73178=CARTESIAN_POINT('Ctrl Pts',(0.0297406827468052,0.235313074254126,
-0.103155166051736));
#73179=CARTESIAN_POINT('Ctrl Pts',(0.0319065096461671,0.235029203762183,
-0.103306364786636));
#73180=CARTESIAN_POINT('Ctrl Pts',(0.0349757976741866,0.23458370635857,
-0.10351886394209));
#73181=CARTESIAN_POINT('Ctrl Pts',(0.0358826423319724,0.234446705589172,
-0.103581428036273));
#73182=CARTESIAN_POINT('Ctrl Pts',(0.0374456242908962,0.234201298140421,
-0.10368885301994));
#73183=CARTESIAN_POINT('Ctrl Pts',(0.0381021378283496,0.234095386469795,
-0.103733851438361));
#73184=CARTESIAN_POINT('Ctrl Pts',(0.0394782195698376,0.23386744842694,
-0.103827898609573));
#73185=CARTESIAN_POINT('Ctrl Pts',(0.0401976813562165,0.23374486027367,
-0.103876915329461));
#73186=CARTESIAN_POINT('Ctrl Pts',(0.0421387178844203,0.233404902524112,
-0.104008768952267));
#73187=CARTESIAN_POINT('Ctrl Pts',(0.0433591924056388,0.233181261401142,
-0.104091258861908));
#73188=CARTESIAN_POINT('Ctrl Pts',(0.0490415825753238,0.232093856033384,
-0.104473619026303));
#73189=CARTESIAN_POINT('Ctrl Pts',(0.05348016031268,0.231111474826344,-0.104767380930168));
#73190=CARTESIAN_POINT('Ctrl Pts',(0.0621535256294052,0.228928517752236,
-0.105336649232027));
#73191=CARTESIAN_POINT('Ctrl Pts',(0.0663884748542621,0.227736472978143,
-0.105612325596284));
#73192=CARTESIAN_POINT('Ctrl Pts',(0.0912801443464492,0.21997657121836,
-0.107232006774772));
#73193=CARTESIAN_POINT('Ctrl Pts',(0.110989247272626,0.210720560787885,
-0.108522448033418));
#73194=CARTESIAN_POINT('Ctrl Pts',(0.132540244981078,0.196726297267704,
-0.110171268580961));
#73195=CARTESIAN_POINT('Ctrl Pts',(0.135856563976942,0.194450876843222,
-0.110432086465231));
#73196=CARTESIAN_POINT('Ctrl Pts',(0.140447843833548,0.191125871940096,
-0.110804269739766));
#73197=CARTESIAN_POINT('Ctrl Pts',(0.141772263293761,0.190145525565056,
-0.110912974506636));
#73198=CARTESIAN_POINT('Ctrl Pts',(0.1440340085122,0.188434596153315,-0.111101002614679));
#73199=CARTESIAN_POINT('Ctrl Pts',(0.144976268251543,0.187710612888308,
-0.111180064330605));
#73200=CARTESIAN_POINT('Ctrl Pts',(0.14676948991735,0.186311238702517,-0.111331950162483));
#73201=CARTESIAN_POINT('Ctrl Pts',(0.147621331739057,0.18563701997331,-0.111404726089653));
#73202=CARTESIAN_POINT('Ctrl Pts',(0.149830301012876,0.18386383818349,-0.111595104158352));
#73203=CARTESIAN_POINT('Ctrl Pts',(0.151179955263766,0.182755713817817,
-0.111713075262875));
#73204=CARTESIAN_POINT('Ctrl Pts',(0.155838073374351,0.178844288287787,
-0.112126128294458));
#73205=CARTESIAN_POINT('Ctrl Pts',(0.159081622531094,0.175965387535873,
-0.112424298257366));
#73206=CARTESIAN_POINT('Ctrl Pts',(0.175792944629793,0.160292981960417,
-0.114018569877111));
#73207=CARTESIAN_POINT('Ctrl Pts',(0.187800063385754,0.146040767498145,
-0.115378112400515));
#73208=CARTESIAN_POINT('Ctrl Pts',(0.204197668210822,0.121166335832178,
-0.117552510211982));
#73209=CARTESIAN_POINT('Ctrl Pts',(0.209703168483444,0.111367009378906,
-0.11836556833137));
#73210=CARTESIAN_POINT('Ctrl Pts',(0.215123329420001,0.0998804605168641,
-0.119244528014781));
#73211=CARTESIAN_POINT('Ctrl Pts',(0.215739926291081,0.09854155335073,-0.119345881672176));
#73212=CARTESIAN_POINT('Ctrl Pts',(0.216663241156643,0.0964864100011733,
-0.119499682372998));
#73213=CARTESIAN_POINT('Ctrl Pts',(0.216978965820279,0.0957742962353528,
-0.119552652571218));
#73214=CARTESIAN_POINT('Ctrl Pts',(0.217553184764051,0.0944617369030223,
-0.119649677852005));
#73215=CARTESIAN_POINT('Ctrl Pts',(0.217812704576054,0.0938617796454056,
-0.119693792594117));
#73216=CARTESIAN_POINT('Ctrl Pts',(0.21839693045004,0.0924956957159582,
-0.119793718175686));
#73217=CARTESIAN_POINT('Ctrl Pts',(0.21872008856859,0.0917289260012577,
-0.119849435273378));
#73218=CARTESIAN_POINT('Ctrl Pts',(0.219550943832558,0.0897281677865304,
-0.11999389835299));
#73219=CARTESIAN_POINT('Ctrl Pts',(0.22005228305086,0.0884915473765325,
-0.120082279464231));
#73220=CARTESIAN_POINT('Ctrl Pts',(0.223871299255121,0.0788382415558933,
-0.120765655145308));
#73221=CARTESIAN_POINT('Ctrl Pts',(0.226715789494457,0.070241141679544,
-0.121335839871748));
#73222=CARTESIAN_POINT('Ctrl Pts',(0.232587774936777,0.0483709533665607,
-0.12274029999639));
#73223=CARTESIAN_POINT('Ctrl Pts',(0.234977717149941,0.0349615070469867,
-0.123561780396935));
#73224=CARTESIAN_POINT('Ctrl Pts',(0.237139121633588,0.0111280437616441,
-0.125046799678374));
#73225=CARTESIAN_POINT('Ctrl Pts',(0.237398690208547,0.000786308062397829,
-0.1256990214052));
#73226=CARTESIAN_POINT('Ctrl Pts',(0.236892216344357,-0.0117968966932127,
-0.126519987660863));
#73227=CARTESIAN_POINT('Ctrl Pts',(0.236769044922754,-0.0140537441573658,
-0.126668275838954));
#73228=CARTESIAN_POINT('Ctrl Pts',(0.236522534332127,-0.0176302863716958,
-0.126905090297152));
#73229=CARTESIAN_POINT('Ctrl Pts',(0.236420352132248,-0.0189513382505818,
-0.126992954605069));
#73230=CARTESIAN_POINT('Ctrl Pts',(0.236206847835148,-0.0214401884444225,
-0.127159263198825));
#73231=CARTESIAN_POINT('Ctrl Pts',(0.236097920001129,-0.0226081562903602,
-0.12723763008589));
#73232=CARTESIAN_POINT('Ctrl Pts',(0.235832225310229,-0.02524529875237,
-0.127415323371018));
#73233=CARTESIAN_POINT('Ctrl Pts',(0.235670386127033,-0.0267139015321142,
-0.127514806058743));
#73234=CARTESIAN_POINT('Ctrl Pts',(0.235150194295314,-0.0310609107078595,
-0.127810882168602));
#73235=CARTESIAN_POINT('Ctrl Pts',(0.234752759183562,-0.0339342719189924,
-0.128008689105845));
#73236=CARTESIAN_POINT('Ctrl Pts',(0.231275530909281,-0.0560738064319622,
-0.12954971415502));
#73237=CARTESIAN_POINT('Ctrl Pts',(0.225882086601258,-0.0748974520192039,
-0.130968446756744));
#73238=CARTESIAN_POINT('Ctrl Pts',(0.214960827071432,-0.100569957832654,
-0.1330036856912));
#73239=CARTESIAN_POINT('Ctrl Pts',(0.211266000785236,-0.108116455798295,
-0.133614122015012));
#73240=CARTESIAN_POINT('Ctrl Pts',(0.205089425930616,-0.119200361663949,
-0.134515751058621));
#73241=CARTESIAN_POINT('Ctrl Pts',(0.202898816247151,-0.122892126758162,
-0.134816909096948));
#73242=CARTESIAN_POINT('Ctrl Pts',(0.199979768200804,-0.127520447391947,
-0.135193689043195));
#73243=CARTESIAN_POINT('Ctrl Pts',(0.199343025299983,-0.128513542483922,
-0.135274486758466));
#73244=CARTESIAN_POINT('Ctrl Pts',(0.198305132959889,-0.130106014060527,
-0.135403920471898));
#73245=CARTESIAN_POINT('Ctrl Pts',(0.197908623051454,-0.130708368553989,
-0.135452848881824));
#73246=CARTESIAN_POINT('Ctrl Pts',(0.197140680941502,-0.131863474879834,
-0.135546604232513));
#73247=CARTESIAN_POINT('Ctrl Pts',(0.196769662478786,-0.132416479442879,
-0.135591455544656));
#73248=CARTESIAN_POINT('Ctrl Pts',(0.195945035774624,-0.133634469811613,
-0.135690180169615));
#73249=CARTESIAN_POINT('Ctrl Pts',(0.195490357401895,-0.134298729616357,
-0.13574398258863));
#73250=CARTESIAN_POINT('Ctrl Pts',(0.193868397689006,-0.136642631146042,
-0.13593373893578));
#73251=CARTESIAN_POINT('Ctrl Pts',(0.192682740122091,-0.138309531927601,
-0.136068521644786));
#73252=CARTESIAN_POINT('Ctrl Pts',(0.1827836108456,-0.15185217967709,-0.137164068017958));
#73253=CARTESIAN_POINT('Ctrl Pts',(0.17300149511792,-0.162909600824409,
-0.138063104962052));
#73254=CARTESIAN_POINT('Ctrl Pts',(0.153872711728283,-0.180851474159983,
-0.139670676231541));
#73255=CARTESIAN_POINT('Ctrl Pts',(0.144930104029103,-0.188093876450735,
-0.140375369078716));
#73256=CARTESIAN_POINT('Ctrl Pts',(0.132003548327169,-0.197091793980823,
-0.141370829727221));
#73257=CARTESIAN_POINT('Ctrl Pts',(0.128444046254087,-0.199429776545429,
-0.141642628895989));
#73258=CARTESIAN_POINT('Ctrl Pts',(0.122107333326926,-0.203351875156971,
-0.142124177396081));
#73259=CARTESIAN_POINT('Ctrl Pts',(0.119357391255386,-0.20497804163141,
-0.142332417952089));
#73260=CARTESIAN_POINT('Ctrl Pts',(0.115258162000108,-0.207291642524837,
-0.142642215903759));
#73261=CARTESIAN_POINT('Ctrl Pts',(0.11393371946252,-0.20802253810478,-0.142742216090707));
#73262=CARTESIAN_POINT('Ctrl Pts',(0.111568572310416,-0.20929838535573,
-0.142920673804633));
#73263=CARTESIAN_POINT('Ctrl Pts',(0.110530630974945,-0.209848373763131,
-0.142998949300023));
#73264=CARTESIAN_POINT('Ctrl Pts',(0.108335743067134,-0.210990607864978,
-0.143164412619173));
#73265=CARTESIAN_POINT('Ctrl Pts',(0.107177931467915,-0.211581097271691,
-0.143251659075141));
#73266=CARTESIAN_POINT('Ctrl Pts',(0.104090466951129,-0.213123873866501,
-0.143484250993119));
#73267=CARTESIAN_POINT('Ctrl Pts',(0.102152646038065,-0.214059448044098,
-0.143630171686381));
#73268=CARTESIAN_POINT('Ctrl Pts',(0.0933807409431472,-0.218148261529492,
-0.144290612805715));
#73269=CARTESIAN_POINT('Ctrl Pts',(0.0864123022932157,-0.221001174729244,
-0.144815208604353));
#73270=CARTESIAN_POINT('Ctrl Pts',(0.064578534578444,-0.228749412997202,
-0.146459115906403));
#73271=CARTESIAN_POINT('Ctrl Pts',(0.0493560779889504,-0.232509276452619,
-0.147608394117222));
#73272=CARTESIAN_POINT('Ctrl Pts',(0.0239346547052643,-0.236177926863205,
-0.149478070160238));
#73273=CARTESIAN_POINT('Ctrl Pts',(0.0139103833567047,-0.236979809411012,
-0.150202021012649));
#73274=CARTESIAN_POINT('Ctrl Pts',(0.0024051977859521,-0.237167294413206,
-0.150998016541098));
#73275=CARTESIAN_POINT('Ctrl Pts',(0.000945742120645826,-0.237177605090394,
-0.151098340038964));
#73276=CARTESIAN_POINT('Ctrl Pts',(-0.00129349645152199,-0.237172754510377,
-0.151251175640611));
#73277=CARTESIAN_POINT('Ctrl Pts',(-0.00207323299373263,-0.237167220256647,
-0.15130419241869));
#73278=CARTESIAN_POINT('Ctrl Pts',(-0.0035086113051823,-0.237149953059226,
-0.151401397571196));
#73279=CARTESIAN_POINT('Ctrl Pts',(-0.00416423374441061,-0.237139346727902,
-0.15144564493904));
#73280=CARTESIAN_POINT('Ctrl Pts',(-0.00565833808986251,-0.237108977521131,
-0.151546140231133));
#73281=CARTESIAN_POINT('Ctrl Pts',(-0.00649676585406703,-0.237087486170394,
-0.151602291692027));
#73282=CARTESIAN_POINT('Ctrl Pts',(-0.00869278053640779,-0.2370195378284,
-0.151748770809671));
#73283=CARTESIAN_POINT('Ctrl Pts',(-0.0100501360724432,-0.236965864044813,
-0.151838715524392));
#73284=CARTESIAN_POINT('Ctrl Pts',(-0.0230833179739347,-0.236338303478938,
-0.152697294297803));
#73285=CARTESIAN_POINT('Ctrl Pts',(-0.0347038318256782,-0.234913503793368,
-0.153424178222884));
#73286=CARTESIAN_POINT('Ctrl Pts',(-0.0602796956831921,-0.229837268003803,
-0.15502840576495));
#73287=CARTESIAN_POINT('Ctrl Pts',(-0.074101590421285,-0.225760377299027,
-0.155899790937294));
#73288=CARTESIAN_POINT('Ctrl Pts',(-0.0919352750746342,-0.218684646942566,
-0.157106642431737));
#73289=CARTESIAN_POINT('Ctrl Pts',(-0.0963465458354181,-0.216777324111726,
-0.157412086840691));
#73290=CARTESIAN_POINT('Ctrl Pts',(-0.103867642789056,-0.213250462402792,
-0.157947437397418));
#73291=CARTESIAN_POINT('Ctrl Pts',(-0.107005170831192,-0.211693500796118,
-0.158175300989801));
#73292=CARTESIAN_POINT('Ctrl Pts',(-0.111494957946378,-0.209340179707107,
-0.158508607580227));
#73293=CARTESIAN_POINT('Ctrl Pts',(-0.112875693782438,-0.208598931067458,
-0.158612119598968));
#73294=CARTESIAN_POINT('Ctrl Pts',(-0.11528358032905,-0.207275349768651,
-0.158794469453041));
#73295=CARTESIAN_POINT('Ctrl Pts',(-0.116313928072974,-0.206698922505567,
-0.15887309467931));
#73296=CARTESIAN_POINT('Ctrl Pts',(-0.118444549876502,-0.205485972561805,
-0.159036948065097));
#73297=CARTESIAN_POINT('Ctrl Pts',(-0.1195440939656,-0.204848250673099,
-0.159122217643613));
#73298=CARTESIAN_POINT('Ctrl Pts',(-0.122382674859691,-0.203171271887754,
-0.159344230093433));
#73299=CARTESIAN_POINT('Ctrl Pts',(-0.12411358575642,-0.202118535053269,
-0.159481460259121));
#73300=CARTESIAN_POINT('Ctrl Pts',(-0.131269589973405,-0.19763968279577,
-0.160056726445009));
#73301=CARTESIAN_POINT('Ctrl Pts',(-0.136567555451433,-0.194016593814558,
-0.160501955461516));
#73302=CARTESIAN_POINT('Ctrl Pts',(-0.154994307295865,-0.180286238218627,
-0.16212242874649));
#73303=CARTESIAN_POINT('Ctrl Pts',(-0.167202170236288,-0.169025639410055,
-0.163337922385332));
#73304=CARTESIAN_POINT('Ctrl Pts',(-0.185031388432316,-0.148742907379374,
-0.165305156860093));
#73305=CARTESIAN_POINT('Ctrl Pts',(-0.191402175016785,-0.140450442205517,
-0.166059085705771));
#73306=CARTESIAN_POINT('Ctrl Pts',(-0.198020970858295,-0.130544350485439,
-0.166883324480858));
#73307=CARTESIAN_POINT('Ctrl Pts',(-0.198824594959166,-0.129317102719204,
-0.166984167750053));
#73308=CARTESIAN_POINT('Ctrl Pts',(-0.200038509967097,-0.127425213109616,
-0.167137595701303));
#73309=CARTESIAN_POINT('Ctrl Pts',(-0.200456973158922,-0.126765895895795,
-0.167190691833981));
#73310=CARTESIAN_POINT('Ctrl Pts',(-0.201220830419954,-0.125549145830893,
-0.167287977667876));
#73311=CARTESIAN_POINT('Ctrl Pts',(-0.201567169900439,-0.124992346368357,
-0.167332226924011));
#73312=CARTESIAN_POINT('Ctrl Pts',(-0.202350456624617,-0.123721357341604,
-0.167432627053454));
#73313=CARTESIAN_POINT('Ctrl Pts',(-0.202785935199133,-0.123006284789944,
-0.167488682374463));
#73314=CARTESIAN_POINT('Ctrl Pts',(-0.203914684663908,-0.121130548129553,
-0.167634641480022));
#73315=CARTESIAN_POINT('Ctrl Pts',(-0.204601845898348,-0.119966216808555,
-0.16772416768257));
#73316=CARTESIAN_POINT('Ctrl Pts',(-0.210346950344549,-0.11003870169986,
-0.168478985290338));
#73317=CARTESIAN_POINT('Ctrl Pts',(-0.214849973970703,-0.100964833240656,
-0.169113162522728));
#73318=CARTESIAN_POINT('Ctrl Pts',(-0.219517946093408,-0.0898203819165326,
-0.169859698398523));
#73319=CARTESIAN_POINT('Ctrl Pts',(-0.220253428481769,-0.0880014605055449,
-0.169980543942454));
#73320=CARTESIAN_POINT('Ctrl Pts',(-0.221250697507531,-0.0854442644068944,
-0.170149299073959));
#73321=CARTESIAN_POINT('Ctrl Pts',(-0.221531518372763,-0.0847135162836387,
-0.170197393619803));
#73322=CARTESIAN_POINT('Ctrl Pts',(-0.225436883741637,-0.0743988014777939,
-0.170874601171089));
#73323=CARTESIAN_POINT('Ctrl Pts',(-0.228440214760001,-0.0645912679262485,
-0.171498899042203));
#73324=CARTESIAN_POINT('Ctrl Pts',(-0.233067808386633,-0.0450373123278173,
-0.172748038565983));
#73325=CARTESIAN_POINT('Ctrl Pts',(-0.234736445492843,-0.0353231998860428,
-0.173370695311321));
#73326=CARTESIAN_POINT('Ctrl Pts',(-0.236036555603795,-0.0233173233311289,
-0.174158148960352));
#73327=CARTESIAN_POINT('Ctrl Pts',(-0.236245343936131,-0.0210971576527419,
-0.174304481991065));
#73328=CARTESIAN_POINT('Ctrl Pts',(-0.236527566576646,-0.0175620133324477,
-0.174538772081519));
#73329=CARTESIAN_POINT('Ctrl Pts',(-0.236621410058296,-0.0162487613803373,
-0.174626088405674));
#73330=CARTESIAN_POINT('Ctrl Pts',(-0.236778066356169,-0.0137658907706906,
-0.174791732887196));
#73331=CARTESIAN_POINT('Ctrl Pts',(-0.236843158614524,-0.0125964514341567,
-0.174869987076174));
#73332=CARTESIAN_POINT('Ctrl Pts',(-0.236971023209236,-0.00994552459101086,
-0.175047931581799));
#73333=CARTESIAN_POINT('Ctrl Pts',(-0.237028568816733,-0.0084638461175782,
-0.175147782463482));
#73334=CARTESIAN_POINT('Ctrl Pts',(-0.237141608843325,-0.00462546271417778,
-0.17540751224517));
#73335=CARTESIAN_POINT('Ctrl Pts',(-0.237175866105723,-0.00226834485232048,
-0.175568045190495));
#73336=CARTESIAN_POINT('Ctrl Pts',(-0.23717374932495,0.00338407696309937,
-0.175955600589388));
#73337=CARTESIAN_POINT('Ctrl Pts',(-0.237103840333012,0.00667880153782812,
-0.176183619433192));
#73338=CARTESIAN_POINT('Ctrl Pts',(-0.236645877390351,0.0175626458177593,
-0.176944017009669));
#73339=CARTESIAN_POINT('Ctrl Pts',(-0.235961820736989,0.0251339961851816,
-0.177484688742312));
#73340=CARTESIAN_POINT('Ctrl Pts',(-0.233645105216224,0.0417981664330959,
-0.178697684000097));
#73341=CARTESIAN_POINT('Ctrl Pts',(-0.231842309578179,0.0508552074570876,
-0.179372493758461));
#73342=CARTESIAN_POINT('Ctrl Pts',(-0.228880033345431,0.0622277197680743,
-0.18023024885811));
#73343=CARTESIAN_POINT('Ctrl Pts',(-0.228204439465065,0.0646613703820853,
-0.180414394828264));
#73344=CARTESIAN_POINT('Ctrl Pts',(-0.224772007709468,0.0763012057397664,
-0.181296935440569));
#73345=CARTESIAN_POINT('Ctrl Pts',(-0.221495882486234,0.0853460401025865,
-0.181988494429987));
#73346=CARTESIAN_POINT('Ctrl Pts',(-0.217145550247915,0.0954023019437799,
-0.182746764247662));
#73347=CARTESIAN_POINT('Ctrl Pts',(-0.216601092375262,0.0966320661011829,
-0.182839298312313));
#73348=CARTESIAN_POINT('Ctrl Pts',(-0.215701529202356,0.098618095325905,
-0.18298834609361));
#73349=CARTESIAN_POINT('Ctrl Pts',(-0.215352845971618,0.0993772117321909,
-0.183045222763101));
#73350=CARTESIAN_POINT('Ctrl Pts',(-0.214723124938131,0.100729294572572,
-0.183146339223));
#73351=CARTESIAN_POINT('Ctrl Pts',(-0.214443630171735,0.101322952392927,
-0.183190669843936));
#73352=CARTESIAN_POINT('Ctrl Pts',(-0.213824830519985,0.102623276746964,
-0.183287622092679));
#73353=CARTESIAN_POINT('Ctrl Pts',(-0.213484484020065,0.103329425646501,
-0.183340178991159));
#73354=CARTESIAN_POINT('Ctrl Pts',(-0.212492233791753,0.105362309849602,
-0.18349124804005));
#73355=CARTESIAN_POINT('Ctrl Pts',(-0.211831405379961,0.106684683662526,
-0.18358922882327));
#73356=CARTESIAN_POINT('Ctrl Pts',(-0.206151449967395,0.117789869820153,
-0.184410350524637));
#73357=CARTESIAN_POINT('Ctrl Pts',(-0.200469284858491,0.127220304297074,
-0.185096652792071));
#73358=CARTESIAN_POINT('Ctrl Pts',(-0.183813048715642,0.150959598894989,
-0.186884163567184));
#73359=CARTESIAN_POINT('Ctrl Pts',(-0.171830478782721,0.164469721334244,
-0.187969515819806));
#73360=CARTESIAN_POINT('Ctrl Pts',(-0.154851828792529,0.179711103260258,
-0.189424900495335));
#73361=CARTESIAN_POINT('Ctrl Pts',(-0.15117145590068,0.18281782001336,-0.189735834443007));
#73362=CARTESIAN_POINT('Ctrl Pts',(-0.145969417315702,0.18694448614643,
-0.19017086984896));
#73363=CARTESIAN_POINT('Ctrl Pts',(-0.14452655033769,0.188062190857791,
-0.190291076608971));
#73364=CARTESIAN_POINT('Ctrl Pts',(-0.142188513756844,0.189830533241875,
-0.190485212410213));
#73365=CARTESIAN_POINT('Ctrl Pts',(-0.141301420632521,0.190491766887114,
-0.190558723771199));
#73366=CARTESIAN_POINT('Ctrl Pts',(-0.139452258873633,0.191850096648846,
-0.190711675294912));
#73367=CARTESIAN_POINT('Ctrl Pts',(-0.138489515924331,0.192546217774897,
-0.190791150379207));
#73368=CARTESIAN_POINT('Ctrl Pts',(-0.136211587036532,0.194167374996316,
-0.190978850828351));
#73369=CARTESIAN_POINT('Ctrl Pts',(-0.134892157681595,0.195086318151782,
-0.191087305076769));
#73370=CARTESIAN_POINT('Ctrl Pts',(-0.130477949500889,0.198094491417262,
-0.191449333368615));
#73371=CARTESIAN_POINT('Ctrl Pts',(-0.127343321667718,0.200123957843785,
-0.191705122435571));
#73372=CARTESIAN_POINT('Ctrl Pts',(-0.115042864309425,0.207681676565704,
-0.192704482667673));
#73373=CARTESIAN_POINT('Ctrl Pts',(-0.105555866580389,0.212660396015786,
-0.193466874231611));
#73374=CARTESIAN_POINT('Ctrl Pts',(-0.086051537853299,0.221268782257148,
-0.195010864836056));
#73375=CARTESIAN_POINT('Ctrl Pts',(-0.0760598859657186,0.224899145862902,
-0.195790513614848));
#73376=CARTESIAN_POINT('Ctrl Pts',(-0.0579878194108664,0.230122849107711,
-0.197157622533095));
#73377=CARTESIAN_POINT('Ctrl Pts',(-0.0500038365085975,0.231988649239616,
-0.19774717899015));
#73378=CARTESIAN_POINT('Ctrl Pts',(-0.0419392735105505,0.233437524752143,
-0.198319131484844));
#73379=CARTESIAN_POINT('',(-0.237174944070688,0.000162880526358662,-0.1956589891905));
#73380=CARTESIAN_POINT('Ctrl Pts',(-0.0419392741328085,0.233437524640348,
-0.217838756538471));
#73381=CARTESIAN_POINT('Ctrl Pts',(-0.0558566731803301,0.230937131377658,
-0.216890940349756));
#73382=CARTESIAN_POINT('Ctrl Pts',(-0.0695275470206164,0.227191865779455,
-0.215943124161042));
#73383=CARTESIAN_POINT('Ctrl Pts',(-0.082723246704858,0.222281004765606,
-0.214995307972327));
#73384=CARTESIAN_POINT('Ctrl Pts',(-0.0893484389765401,0.219815398604902,
-0.214519435935322));
#73385=CARTESIAN_POINT('Ctrl Pts',(-0.0958541374193577,0.21705674966462,
-0.214043563898317));
#73386=CARTESIAN_POINT('Ctrl Pts',(-0.102213610392895,0.214019528257235,
-0.213567691861312));
#73387=CARTESIAN_POINT('Ctrl Pts',(-0.114880326844257,0.207970029733153,
-0.212619856060302));
#73388=CARTESIAN_POINT('Ctrl Pts',(-0.12705087675837,0.200771692096791,
-0.211672020259292));
#73389=CARTESIAN_POINT('Ctrl Pts',(-0.138508390745754,0.192528975268715,
-0.210724184458281));
#73390=CARTESIAN_POINT('Ctrl Pts',(-0.149942695774464,0.184302955332691,
-0.209778268644623));
#73391=CARTESIAN_POINT('Ctrl Pts',(-0.160666120031039,0.175037180079499,
-0.208832352830964));
#73392=CARTESIAN_POINT('Ctrl Pts',(-0.170488576055934,0.16488064185774,
-0.207886437017305));
#73393=CARTESIAN_POINT('Ctrl Pts',(-0.180309458097597,0.154725731153661,
-0.206940672780363));
#73394=CARTESIAN_POINT('Ctrl Pts',(-0.189229043617759,0.143680904924962,
-0.20599490854342));
#73395=CARTESIAN_POINT('Ctrl Pts',(-0.197092978050972,0.131933083902405,
-0.205049144306477));
#73396=CARTESIAN_POINT('Ctrl Pts',(-0.204955596245962,0.120187229189613,
-0.204103538368291));
#73397=CARTESIAN_POINT('Ctrl Pts',(-0.211762464883004,0.10773931743606,
-0.203157932430105));
#73398=CARTESIAN_POINT('Ctrl Pts',(-0.217402991910532,0.0948046398302793,
-0.202212326491919));
#73399=CARTESIAN_POINT('Ctrl Pts',(-0.223056723787191,0.081839681283462,
-0.201264506827304));
#73400=CARTESIAN_POINT('Ctrl Pts',(-0.227538369305371,0.0683864664481,-0.200316687162689));
#73401=CARTESIAN_POINT('Ctrl Pts',(-0.230785986797566,0.0546791452280835,
-0.199368867498074));
#73402=CARTESIAN_POINT('Ctrl Pts',(-0.232710607055604,0.0465558400152984,
-0.198807165594489));
#73403=CARTESIAN_POINT('Ctrl Pts',(-0.234202800191289,0.0383435642722978,
-0.198245463690903));
#73404=CARTESIAN_POINT('Ctrl Pts',(-0.235258248560059,0.0300921436500207,
-0.197683761787317));
#73405=CARTESIAN_POINT('Ctrl Pts',(-0.236526443736657,0.0201774835464205,
-0.197008837588379));
#73406=CARTESIAN_POINT('Ctrl Pts',(-0.237168064099412,0.0101810014103574,
-0.19633391338944));
#73407=CARTESIAN_POINT('Ctrl Pts',(-0.237174944070688,0.000162880526358662,
-0.1956589891905));
#73408=CARTESIAN_POINT('Ctrl Pts',(-0.0419392741328228,0.233437524640346,
-0.117607182502807));
#73409=CARTESIAN_POINT('Ctrl Pts',(-0.0419233069101264,0.233440393303946,
-0.117608254364183));
#73410=CARTESIAN_POINT('Ctrl Pts',(-0.0419073393854834,0.233443260337026,
-0.11760932631259));
#73411=CARTESIAN_POINT('Ctrl Pts',(-0.0406613141794025,0.233666856699471,
-0.11769298041077));
#73412=CARTESIAN_POINT('Ctrl Pts',(-0.0394295655190218,0.233877856112213,
-0.117776051018579));
#73413=CARTESIAN_POINT('Ctrl Pts',(-0.0374715243177032,0.23419736268533,
-0.117908781232462));
#73414=CARTESIAN_POINT('Ctrl Pts',(-0.0367462751363644,0.234312251173553,
-0.117958091049391));
#73415=CARTESIAN_POINT('Ctrl Pts',(-0.0353639204475622,0.234524657664918,
-0.118052377902706));
#73416=CARTESIAN_POINT('Ctrl Pts',(-0.0347069258778216,0.234622784854061,
-0.11809732065703));
#73417=CARTESIAN_POINT('Ctrl Pts',(-0.033144621262886,0.234849421577537,
-0.118204493981608));
#73418=CARTESIAN_POINT('Ctrl Pts',(-0.0322389705330159,0.234975457107885,
-0.118266860235112));
#73419=CARTESIAN_POINT('Ctrl Pts',(-0.0291755708059842,0.235383734052467,
-0.118478572780337));
#73420=CARTESIAN_POINT('Ctrl Pts',(-0.0270147491157533,0.235641504566257,
-0.11862917365776));
#73421=CARTESIAN_POINT('Ctrl Pts',(-0.0217308353624622,0.236198208205375,
-0.119000041144256));
#73422=CARTESIAN_POINT('Ctrl Pts',(-0.0186048258583135,0.2364649682449,
-0.119221657036352));
#73423=CARTESIAN_POINT('Ctrl Pts',(-0.00576030112902554,0.237304805753033,
-0.120138982690224));
#73424=CARTESIAN_POINT('Ctrl Pts',(0.00398336794439466,0.237341239431457,
-0.120850203430668));
#73425=CARTESIAN_POINT('Ctrl Pts',(0.0312231769978453,0.235765020726392,
-0.122843171008102));
#73426=CARTESIAN_POINT('Ctrl Pts',(0.0485818250559329,0.232809063584704,
-0.124114015434344));
#73427=CARTESIAN_POINT('Ctrl Pts',(0.0684646634710677,0.227099886388252,
-0.125538943349998));
#73428=CARTESIAN_POINT('Ctrl Pts',(0.0714544569375792,0.226176989894679,
-0.12575255085971));
#73429=CARTESIAN_POINT('Ctrl Pts',(0.0758482204165325,0.22472488538814,
-0.126065631322679));
#73430=CARTESIAN_POINT('Ctrl Pts',(0.0772667352360214,0.224241116789075,
-0.126166579372806));
#73431=CARTESIAN_POINT('Ctrl Pts',(0.0797853948396371,0.223355418355039,
-0.12634561859638));
#73432=CARTESIAN_POINT('Ctrl Pts',(0.0808873155438912,0.222958728035803,
-0.126423879998563));
#73433=CARTESIAN_POINT('Ctrl Pts',(0.0832092110477833,0.22210336866464,
-0.126588662580306));
#73434=CARTESIAN_POINT('Ctrl Pts',(0.0844284380617033,0.221642771452417,
-0.126675116542418));
#73435=CARTESIAN_POINT('Ctrl Pts',(0.0876725020877363,0.220386582223038,
-0.126904995179905));
#73436=CARTESIAN_POINT('Ctrl Pts',(0.0896903257542046,0.219573129572948,
-0.127047818471099));
#73437=CARTESIAN_POINT('Ctrl Pts',(0.100002505295372,0.215250062541782,
-0.127777335077885));
#73438=CARTESIAN_POINT('Ctrl Pts',(0.108103802279133,0.211297626187242,
-0.128348759130919));
#73439=CARTESIAN_POINT('Ctrl Pts',(0.125487704905034,0.201554150426609,
-0.129591715403383));
#73440=CARTESIAN_POINT('Ctrl Pts',(0.134634101961298,0.195563055040453,
-0.130257032561207));
#73441=CARTESIAN_POINT('Ctrl Pts',(0.153053908972181,0.181590975116401,
-0.131675820923081));
#73442=CARTESIAN_POINT('Ctrl Pts',(0.162188224000305,0.173481077428067,
-0.132428506538101));
#73443=CARTESIAN_POINT('Ctrl Pts',(0.172094245765931,0.163217135574412,
-0.133359207778695));
#73444=CARTESIAN_POINT('Ctrl Pts',(0.173511686439202,0.161709482481619,
-0.133495434229795));
#73445=CARTESIAN_POINT('Ctrl Pts',(0.175471221910759,0.159569807570801,
-0.133688433008307));
#73446=CARTESIAN_POINT('Ctrl Pts',(0.17603003968329,0.158953132350848,-0.133744018966581));
#73447=CARTESIAN_POINT('Ctrl Pts',(0.177033678867831,0.157833797705537,
-0.133844873059607));
#73448=CARTESIAN_POINT('Ctrl Pts',(0.177479639748936,0.157332160127695,
-0.133890057060902));
#73449=CARTESIAN_POINT('Ctrl Pts',(0.178389254654472,0.156300194070775,
-0.133982995760833));
#73450=CARTESIAN_POINT('Ctrl Pts',(0.178852682950757,0.155769684505577,
-0.134030764903502));
#73451=CARTESIAN_POINT('Ctrl Pts',(0.180042616421704,0.154395197507338,
-0.134154489362849));
#73452=CARTESIAN_POINT('Ctrl Pts',(0.180765542867942,0.153548165504204,
-0.134230696644829));
#73453=CARTESIAN_POINT('Ctrl Pts',(0.183836621162676,0.149898125592831,
-0.134558810662025));
#73454=CARTESIAN_POINT('Ctrl Pts',(0.186125606477016,0.147046272714128,
-0.134814469141503));
#73455=CARTESIAN_POINT('Ctrl Pts',(0.192312433121669,0.138962112472606,
-0.135534700329734));
#73456=CARTESIAN_POINT('Ctrl Pts',(0.196061568367257,0.133620322461467,
-0.136005510592295));
#73457=CARTESIAN_POINT('Ctrl Pts',(0.201770372409919,0.124727917694376,
-0.136773861340206));
#73458=CARTESIAN_POINT('Ctrl Pts',(0.203867807946244,0.121269339854454,
-0.13706916217845));
#73459=CARTESIAN_POINT('Ctrl Pts',(0.214800835754819,0.102155319502525,
-0.138677422479804));
#73460=CARTESIAN_POINT('Ctrl Pts',(0.221924778514198,0.0855846835914042,
-0.139980412817154));
#73461=CARTESIAN_POINT('Ctrl Pts',(0.228002525397906,0.0653946144547187,
-0.141432465470148));
#73462=CARTESIAN_POINT('Ctrl Pts',(0.228838519214608,0.0624062569083836,
-0.141644271690046));
#73463=CARTESIAN_POINT('Ctrl Pts',(0.229990116612161,0.0579548277846998,
-0.141955332757995));
#73464=CARTESIAN_POINT('Ctrl Pts',(0.230350876387253,0.0565038912700911,
-0.142056031237064));
#73465=CARTESIAN_POINT('Ctrl Pts',(0.230969966771371,0.0539094523898376,
-0.142234891463863));
#73466=CARTESIAN_POINT('Ctrl Pts',(0.231233581824808,0.0527672751700546,
-0.142313220550652));
#73467=CARTESIAN_POINT('Ctrl Pts',(0.231773529879102,0.0503460391445611,
-0.14247841560043));
#73468=CARTESIAN_POINT('Ctrl Pts',(0.232047768050413,0.0490665493941061,
-0.142565212226774));
#73469=CARTESIAN_POINT('Ctrl Pts',(0.232753444964353,0.0456358207419901,
-0.14279664962511));
#73470=CARTESIAN_POINT('Ctrl Pts',(0.233165652926233,0.0434807210531672,
-0.142940676721724));
#73471=CARTESIAN_POINT('Ctrl Pts',(0.235161830736234,0.0321980141257359,
-0.143688117149105));
#73472=CARTESIAN_POINT('Ctrl Pts',(0.236240042013914,0.0229885135371988,
-0.144275337543931));
#73473=CARTESIAN_POINT('Ctrl Pts',(0.237397162333193,0.00304624986000087,
-0.145520097420657));
#73474=CARTESIAN_POINT('Ctrl Pts',(0.237292600406242,-0.00767613580710551,
-0.14617274365936));
#73475=CARTESIAN_POINT('Ctrl Pts',(0.235529536730651,-0.0303895884491641,
-0.147571376429492));
#73476=CARTESIAN_POINT('Ctrl Pts',(0.233678080003207,-0.0423340270988234,
-0.148316746171546));
#73477=CARTESIAN_POINT('Ctrl Pts',(0.230452728613299,-0.056105537690637,
-0.14923956944462));
#73478=CARTESIAN_POINT('Ctrl Pts',(0.229952765032285,-0.0581207073085242,
-0.149376249136292));
#73479=CARTESIAN_POINT('Ctrl Pts',(0.229214966752837,-0.0609358300574998,
-0.149569833449145));
#73480=CARTESIAN_POINT('Ctrl Pts',(0.228999250339493,-0.0617415553740832,
-0.149625545766298));
#73481=CARTESIAN_POINT('Ctrl Pts',(0.228601967178426,-0.0631947258300784,
-0.149726607456939));
#73482=CARTESIAN_POINT('Ctrl Pts',(0.228421886341667,-0.0638425766452738,
-0.149771872254705));
#73483=CARTESIAN_POINT('Ctrl Pts',(0.228047528574421,-0.0651674879565829,
-0.149864888607596));
#73484=CARTESIAN_POINT('Ctrl Pts',(0.227852987027905,-0.0658444610035887,
-0.149912654281116));
#73485=CARTESIAN_POINT('Ctrl Pts',(0.227343197449048,-0.0675891305191501,
-0.150036351909273));
#73486=CARTESIAN_POINT('Ctrl Pts',(0.22702344669927,-0.0686554769580445,
-0.150112535588346));
#73487=CARTESIAN_POINT('Ctrl Pts',(0.225622343033365,-0.0732112305367457,
-0.15044038472327));
#73488=CARTESIAN_POINT('Ctrl Pts',(0.224468018572885,-0.0766774475920768,
-0.150695794277266));
#73489=CARTESIAN_POINT('Ctrl Pts',(0.221033683606676,-0.0862469084447028,
-0.151415094649121));
#73490=CARTESIAN_POINT('Ctrl Pts',(0.218581626439671,-0.0922847747616836,
-0.151885204845275));
#73491=CARTESIAN_POINT('Ctrl Pts',(0.21417117132057,-0.101979441210671,
-0.152659601789109));
#73492=CARTESIAN_POINT('Ctrl Pts',(0.212359743947641,-0.105699741909095,
-0.152961708599504));
#73493=CARTESIAN_POINT('Ctrl Pts',(0.202207528789262,-0.125234711837627,
-0.15456962969795));
#73494=CARTESIAN_POINT('Ctrl Pts',(0.192194200116681,-0.140118666259069,
-0.155865231049579));
#73495=CARTESIAN_POINT('Ctrl Pts',(0.178586406111427,-0.156104250519835,
-0.157311032985161));
#73496=CARTESIAN_POINT('Ctrl Pts',(0.17652525903678,-0.158431297410584,
-0.15752322418723));
#73497=CARTESIAN_POINT('Ctrl Pts',(0.173405317849516,-0.161817222802482,
-0.157834711247489));
#73498=CARTESIAN_POINT('Ctrl Pts',(0.172381357010381,-0.162907598925841,
-0.157935457524008));
#73499=CARTESIAN_POINT('Ctrl Pts',(0.170536897323632,-0.16483482783265,
-0.158114343254752));
#73500=CARTESIAN_POINT('Ctrl Pts',(0.169720390364434,-0.1656754145761,-0.158192650681002));
#73501=CARTESIAN_POINT('Ctrl Pts',(0.167979939349333,-0.167440823588724,
-0.158357738947634));
#73502=CARTESIAN_POINT('Ctrl Pts',(0.167054508930708,-0.168364130948288,
-0.158444450935687));
#73503=CARTESIAN_POINT('Ctrl Pts',(0.164558690474189,-0.170813384518051,
-0.158675514807385));
#73504=CARTESIAN_POINT('Ctrl Pts',(0.162974700843463,-0.172325338686806,
-0.158819255828806));
#73505=CARTESIAN_POINT('Ctrl Pts',(0.154626504230812,-0.180075801523522,
-0.159562374211088));
#73506=CARTESIAN_POINT('Ctrl Pts',(0.147523963190298,-0.185939130802494,
-0.160145780548163));
#73507=CARTESIAN_POINT('Ctrl Pts',(0.131409680509794,-0.197735720883886,
-0.161390469743401));
#73508=CARTESIAN_POINT('Ctrl Pts',(0.12229817477599,-0.20349713804708,-0.162046523425559));
#73509=CARTESIAN_POINT('Ctrl Pts',(0.102170866704393,-0.214382491576574,
-0.163451090007482));
#73510=CARTESIAN_POINT('Ctrl Pts',(0.0910904829798847,-0.219319828080074,
-0.164198943852727));
#73511=CARTESIAN_POINT('Ctrl Pts',(0.0777298910860151,-0.224085576513676,
-0.16512444955251));
#73512=CARTESIAN_POINT('Ctrl Pts',(0.0757675930409317,-0.224756652171625,
-0.165260973505059));
#73513=CARTESIAN_POINT('Ctrl Pts',(0.0730048228234889,-0.225661186261036,
-0.165454351537729));
#73514=CARTESIAN_POINT('Ctrl Pts',(0.0722114685927882,-0.225916309485954,
-0.165510015129837));
#73515=CARTESIAN_POINT('Ctrl Pts',(0.070776085624787,-0.226369560184181,
-0.165610993478031));
#73516=CARTESIAN_POINT('Ctrl Pts',(0.070134520061887,-0.226569153135777,
-0.165656223794456));
#73517=CARTESIAN_POINT('Ctrl Pts',(0.0688188774111642,-0.226972329940867,
-0.165749190140842));
#73518=CARTESIAN_POINT('Ctrl Pts',(0.0681447300253172,-0.227175641704029,
-0.165796940352851));
#73519=CARTESIAN_POINT('Ctrl Pts',(0.0664028052847694,-0.22769252636039,
-0.165920596091726));
#73520=CARTESIAN_POINT('Ctrl Pts',(0.0653337233026107,-0.228001586806835,
-0.165996753232333));
#73521=CARTESIAN_POINT('Ctrl Pts',(0.0607476486542171,-0.229292470577999,
-0.1663244637223));
#73522=CARTESIAN_POINT('Ctrl Pts',(0.0572106174746963,-0.230200468094717,
-0.166579758981892));
#73523=CARTESIAN_POINT('Ctrl Pts',(0.0473125528260156,-0.232499225371961,
-0.16729866916973));
#73524=CARTESIAN_POINT('Ctrl Pts',(0.0409132710682016,-0.233710205763855,
-0.167768498715436));
#73525=CARTESIAN_POINT('Ctrl Pts',(0.0303334731170175,-0.235264456523317,
-0.168546003443792));
#73526=CARTESIAN_POINT('Ctrl Pts',(0.0261788674989858,-0.235762911008172,
-0.16885152753961));
#73527=CARTESIAN_POINT('Ctrl Pts',(0.00425317270159916,-0.237806758298755,
-0.170459880130942));
#73528=CARTESIAN_POINT('Ctrl Pts',(-0.0136404184221096,-0.237453816122117,
-0.171752365742219));
#73529=CARTESIAN_POINT('Ctrl Pts',(-0.0344117743366196,-0.234685940736986,
-0.173195578486813));
#73530=CARTESIAN_POINT('Ctrl Pts',(-0.0374875775764345,-0.234214312381348,
-0.173407987406293));
#73531=CARTESIAN_POINT('Ctrl Pts',(-0.0420274952558084,-0.233426452746969,
-0.173719719009552));
#73532=CARTESIAN_POINT('Ctrl Pts',(-0.0434992233954118,-0.233156678956929,
-0.173820495945463));
#73533=CARTESIAN_POINT('Ctrl Pts',(-0.046118792410249,-0.232650833931493,
-0.173999404302277));
#73534=CARTESIAN_POINT('Ctrl Pts',(-0.0472676101201849,-0.232420151150761,
-0.174077704045024));
#73535=CARTESIAN_POINT('Ctrl Pts',(-0.0496937718187097,-0.231914244619261,
-0.17424274363375));
#73536=CARTESIAN_POINT('Ctrl Pts',(-0.0509706498374841,-0.231636959024393,
-0.174329414883327));
#73537=CARTESIAN_POINT('Ctrl Pts',(-0.0543788447542903,-0.230867291978971,
-0.174560292661675));
#73538=CARTESIAN_POINT('Ctrl Pts',(-0.0565057846285708,-0.230355946508815,
-0.174703889831387));
#73539=CARTESIAN_POINT('Ctrl Pts',(-0.0675119475841352,-0.227548296392982,
-0.175444886714059));
#73540=CARTESIAN_POINT('Ctrl Pts',(-0.0762601508909911,-0.224767678651007,
-0.176026426779777));
#73541=CARTESIAN_POINT('Ctrl Pts',(-0.0948988896575572,-0.217629324586893,
-0.177270529810449));
#73542=CARTESIAN_POINT('Ctrl Pts',(-0.104696979828549,-0.213088887619416,
-0.177927729059481));
#73543=CARTESIAN_POINT('Ctrl Pts',(-0.124784407854769,-0.202059301641824,
-0.179334359043513));
#73544=CARTESIAN_POINT('Ctrl Pts',(-0.134951920443454,-0.195414976646931,
-0.180083115762509));
#73545=CARTESIAN_POINT('Ctrl Pts',(-0.146206861234186,-0.186761402787457,
-0.181009436949204));
#73546=CARTESIAN_POINT('Ctrl Pts',(-0.147831657988762,-0.185477944843892,
-0.181145746290077));
#73547=CARTESIAN_POINT('Ctrl Pts',(-0.150086069528746,-0.183648702460812,
-0.181338867702054));
#73548=CARTESIAN_POINT('Ctrl Pts',(-0.150729983689493,-0.183120578163806,
-0.181394493315748));
#73549=CARTESIAN_POINT('Ctrl Pts',(-0.151888226556527,-0.182160364754587,
-0.181495422619538));
#73550=CARTESIAN_POINT('Ctrl Pts',(-0.152403532942728,-0.181729455465044,
-0.181540642127857));
#73551=CARTESIAN_POINT('Ctrl Pts',(-0.15344467486292,-0.18085128951155,
-0.181632663444296));
#73552=CARTESIAN_POINT('Ctrl Pts',(-0.153970397898302,-0.180403918199303,
-0.18167947256891));
#73553=CARTESIAN_POINT('Ctrl Pts',(-0.155271847595331,-0.179286598938222,
-0.181796189931273));
#73554=CARTESIAN_POINT('Ctrl Pts',(-0.156045189387923,-0.178613913195304,
-0.181866292779184));
#73555=CARTESIAN_POINT('Ctrl Pts',(-0.157750947807456,-0.177110638746918,
-0.182022538978979));
#73556=CARTESIAN_POINT('Ctrl Pts',(-0.158681208070373,-0.176277661476834,
-0.18210884060396));
#73557=CARTESIAN_POINT('Ctrl Pts',(-0.16138203919936,-0.173820570363269,
-0.182362501518714));
#73558=CARTESIAN_POINT('Ctrl Pts',(-0.163134509806404,-0.172176897345417,
-0.182531046370922));
#73559=CARTESIAN_POINT('Ctrl Pts',(-0.169382400913826,-0.166135868117174,
-0.183145505707788));
#73560=CARTESIAN_POINT('Ctrl Pts',(-0.173727248986793,-0.16158699430277,
-0.183598815142674));
#73561=CARTESIAN_POINT('Ctrl Pts',(-0.179598737349793,-0.154928952377287,
-0.184243778871834));
#73562=CARTESIAN_POINT('Ctrl Pts',(-0.181279606378228,-0.152958787757367,
-0.184432490648436));
#73563=CARTESIAN_POINT('Ctrl Pts',(-0.195745765150561,-0.135429397117074,
-0.186090913059738));
#73564=CARTESIAN_POINT('Ctrl Pts',(-0.206536204325546,-0.118324348639466,
-0.187558681570756));
#73565=CARTESIAN_POINT('Ctrl Pts',(-0.216232155612315,-0.09748682807027,
-0.18913822938638));
#73566=CARTESIAN_POINT('Ctrl Pts',(-0.217382649080613,-0.0948936871644106,
-0.18933161298771));
#73567=CARTESIAN_POINT('Ctrl Pts',(-0.219055091062853,-0.0909339547118214,
-0.189622243280102));
#73568=CARTESIAN_POINT('Ctrl Pts',(-0.219611343117681,-0.0895822258077033,
-0.18972064484483));
#73569=CARTESIAN_POINT('Ctrl Pts',(-0.220589739889991,-0.0871407636020019,
-0.189896951656467));
#73570=CARTESIAN_POINT('Ctrl Pts',(-0.221016390015588,-0.0860528991643905,
-0.18997500655894));
#73571=CARTESIAN_POINT('Ctrl Pts',(-0.221910859804268,-0.0837216555441437,
-0.19014122259533));
#73572=CARTESIAN_POINT('Ctrl Pts',(-0.222376309620995,-0.0824774050709694,
-0.190229302283899));
#73573=CARTESIAN_POINT('Ctrl Pts',(-0.223614668619061,-0.079080291306097,
-0.190468106229765));
#73574=CARTESIAN_POINT('Ctrl Pts',(-0.224366941078171,-0.076920015894052,
-0.190618144707412));
#73575=CARTESIAN_POINT('Ctrl Pts',(-0.228545521215175,-0.06433729207203,
-0.191482158114994));
#73576=CARTESIAN_POINT('Ctrl Pts',(-0.231276852359328,-0.0536973565629997,
-0.192172821148151));
#73577=CARTESIAN_POINT('Ctrl Pts',(-0.235875800516865,-0.0286944258220648,
-0.193746838634687));
#73578=CARTESIAN_POINT('Ctrl Pts',(-0.237185388115221,-0.0142756234224376,
-0.194617895383358));
#73579=CARTESIAN_POINT('Ctrl Pts',(-0.237174937953315,0.000171557107381939,
-0.195520038937142));
#73580=CARTESIAN_POINT('Origin',(0.,0.,-0.9775));
#73581=CARTESIAN_POINT('',(-0.29419993969113,0.000188376579435279,-1.92858238829104));
#73582=CARTESIAN_POINT('',(0.12894108841962,0.264438718264107,-1.96079706282707));
#73583=CARTESIAN_POINT('Ctrl Pts',(-0.29419993969113,0.000188376579435279,
-1.92858238829104));
#73584=CARTESIAN_POINT('Ctrl Pts',(-0.294193636363906,0.0100326921233836,
-1.92911748512889));
#73585=CARTESIAN_POINT('Ctrl Pts',(-0.293693265724678,0.019862149828654,
-1.92965258196674));
#73586=CARTESIAN_POINT('Ctrl Pts',(-0.292703045250943,0.0296406359720001,
-1.93018767880459));
#73587=CARTESIAN_POINT('Ctrl Pts',(-0.291037817615491,0.0460848580323184,
-1.93108753703381));
#73588=CARTESIAN_POINT('Ctrl Pts',(-0.287977283616911,0.0624400269542837,
-1.93198739526302));
#73589=CARTESIAN_POINT('Ctrl Pts',(-0.28354685905932,0.078452652712285,
-1.93288725349224));
#73590=CARTESIAN_POINT('Ctrl Pts',(-0.279125085348672,0.0944340122174017,
-1.93378535465829));
#73591=CARTESIAN_POINT('Ctrl Pts',(-0.273338875571435,0.110073387857488,
-1.93468345582433));
#73592=CARTESIAN_POINT('Ctrl Pts',(-0.266264720315519,0.125126890456442,
-1.93558155699038));
#73593=CARTESIAN_POINT('Ctrl Pts',(-0.259192119958031,0.140177084297433,
-1.9364794607539));
#73594=CARTESIAN_POINT('Ctrl Pts',(-0.250832423035421,0.15464092744763,
-1.93737736451743));
#73595=CARTESIAN_POINT('Ctrl Pts',(-0.241310388426852,0.168294196089116,
-1.93827526828095));
#73596=CARTESIAN_POINT('Ctrl Pts',(-0.2317911197368,0.181943498789488,-1.93917291122536));
#73597=CARTESIAN_POINT('Ctrl Pts',(-0.221110642536091,0.194782053275159,
-1.94007055416976));
#73598=CARTESIAN_POINT('Ctrl Pts',(-0.20943635480893,0.206615714030535,
-1.94096819711417));
#73599=CARTESIAN_POINT('Ctrl Pts',(-0.197734962313328,0.218476849578557,
-1.94186792416038));
#73600=CARTESIAN_POINT('Ctrl Pts',(-0.185035724332008,0.229327885384296,
-1.9427676512066));
#73601=CARTESIAN_POINT('Ctrl Pts',(-0.171542350944017,0.239012262933515,
-1.94366737825281));
#73602=CARTESIAN_POINT('Ctrl Pts',(-0.159523453405146,0.247638389117453,
-1.9444687884614));
#73603=CARTESIAN_POINT('Ctrl Pts',(-0.146875316353266,0.255339274278587,
-1.94527019866999));
#73604=CARTESIAN_POINT('Ctrl Pts',(-0.133759077941881,0.262034633337156,
-1.94607160887857));
#73605=CARTESIAN_POINT('Ctrl Pts',(-0.119199316029112,0.269466858244615,
-1.94696121925813));
#73606=CARTESIAN_POINT('Ctrl Pts',(-0.103967986147468,0.275707332434235,
-1.94785082963768));
#73607=CARTESIAN_POINT('Ctrl Pts',(-0.0882868080160081,0.280640480918816,
-1.94874044001724));
#73608=CARTESIAN_POINT('Ctrl Pts',(-0.0726355375993347,0.285564220722709,
-1.94962835369944));
#73609=CARTESIAN_POINT('Ctrl Pts',(-0.0565368624984817,0.28918527751626,
-1.95051626738163));
#73610=CARTESIAN_POINT('Ctrl Pts',(-0.040232402904419,0.291436088631001,
-1.95140418106383));
#73611=CARTESIAN_POINT('Ctrl Pts',(-0.0239311430304607,0.293686458028214,
-1.95229192049461));
#73612=CARTESIAN_POINT('Ctrl Pts',(-0.00742497013263192,0.294566957618438,
-1.95317965992538));
#73613=CARTESIAN_POINT('Ctrl Pts',(0.00903488855945793,0.294061236460568,
-1.95406739935616));
#73614=CARTESIAN_POINT('Ctrl Pts',(0.0254921775252421,0.29355559425629,
-1.95495500019235));
#73615=CARTESIAN_POINT('Ctrl Pts',(0.0419023600789404,0.291664204113601,
-1.95584260102853));
#73616=CARTESIAN_POINT('Ctrl Pts',(0.0580166101801649,0.288422802398151,
-1.95673020186472));
#73617=CARTESIAN_POINT('Ctrl Pts',(0.0741645751101561,0.285174618902406,
-1.95761965977213));
#73618=CARTESIAN_POINT('Ctrl Pts',(0.0900145886645593,0.280570990771778,
-1.95850911767955));
#73619=CARTESIAN_POINT('Ctrl Pts',(0.105330521385611,0.274698236733757,
-1.95939857558696));
#73620=CARTESIAN_POINT('Ctrl Pts',(0.113357559091118,0.271620342689892,
-1.95986473800033));
#73621=CARTESIAN_POINT('Ctrl Pts',(0.121238206880903,0.268194665714199,
-1.9603309004137));
#73622=CARTESIAN_POINT('Ctrl Pts',(0.12894108841962,0.264438718264107,-1.96079706282707));
#73623=CARTESIAN_POINT('',(-0.128892185405333,0.264462557919712,-1.9608));
#73624=CARTESIAN_POINT('Origin',(0.,0.,-1.9608));
#73625=CARTESIAN_POINT('',(-0.294199832726378,0.000313725630257716,-1.94301761170573));
#73626=CARTESIAN_POINT('Ctrl Pts',(-0.128892185405333,0.264462557919712,
-1.9608));
#73627=CARTESIAN_POINT('Ctrl Pts',(-0.144172453258884,0.257015352036523,
-1.95988042553177));
#73628=CARTESIAN_POINT('Ctrl Pts',(-0.158823731371776,0.248230991355156,
-1.95896085106354));
#73629=CARTESIAN_POINT('Ctrl Pts',(-0.17261306769371,0.238240149557892,
-1.95804127659531));
#73630=CARTESIAN_POINT('Ctrl Pts',(-0.186392524158092,0.228256466052477,
-1.95712236098871));
#73631=CARTESIAN_POINT('Ctrl Pts',(-0.199310661850408,0.217068438626958,
-1.95620344538212));
#73632=CARTESIAN_POINT('Ctrl Pts',(-0.211164165757333,0.204849542591654,
-1.95528452977553));
#73633=CARTESIAN_POINT('Ctrl Pts',(-0.223031084542253,0.192616818155832,
-1.9543645742114));
#73634=CARTESIAN_POINT('Ctrl Pts',(-0.233830441426606,0.179351418393509,
-1.95344461864728));
#73635=CARTESIAN_POINT('Ctrl Pts',(-0.243395958708843,0.165263569137917,
-1.95252466308315));
#73636=CARTESIAN_POINT('Ctrl Pts',(-0.252965853013338,0.151169273515868,
-1.95160428656259));
#73637=CARTESIAN_POINT('Ctrl Pts',(-0.261300398891812,0.136252410350624,
-1.95068391004203));
#73638=CARTESIAN_POINT('Ctrl Pts',(-0.268277579228135,0.120750902619781,
-1.94976353352148));
#73639=CARTESIAN_POINT('Ctrl Pts',(-0.275274713264632,0.105205062877639,
-1.94884052486068));
#73640=CARTESIAN_POINT('Ctrl Pts',(-0.280906460402522,0.0890719304062782,
-1.94791751619988));
#73641=CARTESIAN_POINT('Ctrl Pts',(-0.28509924002603,0.0726089755924176,
-1.94699450753908));
#73642=CARTESIAN_POINT('Ctrl Pts',(-0.28824635057256,0.0602518418114619,
-1.94630169500139));
#73643=CARTESIAN_POINT('Ctrl Pts',(-0.290583772810123,0.0477093161032033,
-1.9456088824637));
#73644=CARTESIAN_POINT('Ctrl Pts',(-0.292099501141714,0.0350930396626186,
-1.94491606992601));
#73645=CARTESIAN_POINT('Ctrl Pts',(-0.293483977099918,0.0235692520220445,
-1.94428325052032));
#73646=CARTESIAN_POINT('Ctrl Pts',(-0.294187418228296,0.0119555623629466,
-1.94365043111464));
#73647=CARTESIAN_POINT('Ctrl Pts',(-0.294199832726315,0.000313725689767731,
-1.94301761170896));
#73648=CARTESIAN_POINT('',(-0.294181798577116,0.000133869447550703,-1.84301761781353));
#73649=CARTESIAN_POINT('Ctrl Pts',(-0.294199832726378,0.000313725630257912,
-1.94301761170573));
#73650=CARTESIAN_POINT('Ctrl Pts',(-0.294217035041623,-0.0158179441453529,
-1.94214073686488));
#73651=CARTESIAN_POINT('Ctrl Pts',(-0.292903174616159,-0.0320111324691114,
-1.94126386202403));
#73652=CARTESIAN_POINT('Ctrl Pts',(-0.290254358978592,-0.0480213191606245,
-1.94038698718318));
#73653=CARTESIAN_POINT('Ctrl Pts',(-0.287610259166518,-0.0640030020765365,
-1.93951167348863));
#73654=CARTESIAN_POINT('Ctrl Pts',(-0.283635983382084,-0.0798015088650099,
-1.93863635979408));
#73655=CARTESIAN_POINT('Ctrl Pts',(-0.278379474364989,-0.0951761958279081,
-1.93776104609953));
#73656=CARTESIAN_POINT('Ctrl Pts',(-0.273122876603055,-0.110551142359301,
-1.93688571762719));
#73657=CARTESIAN_POINT('Ctrl Pts',(-0.266584228486466,-0.125501456989427,
-1.93601038915485));
#73658=CARTESIAN_POINT('Ctrl Pts',(-0.25886143281037,-0.139801282552637,
-1.93513506068251));
#73659=CARTESIAN_POINT('Ctrl Pts',(-0.251138408936953,-0.154101530654787,
-1.9342597063455));
#73660=CARTESIAN_POINT('Ctrl Pts',(-0.242231590358653,-0.167750537452882,
-1.93338435200848));
#73661=CARTESIAN_POINT('Ctrl Pts',(-0.232283958546599,-0.180548615618957,
-1.93250899767147));
#73662=CARTESIAN_POINT('Ctrl Pts',(-0.22231468153334,-0.193374541315195,
-1.93163173863783));
#73663=CARTESIAN_POINT('Ctrl Pts',(-0.211300636300945,-0.205345235053099,
-1.93075447960419));
#73664=CARTESIAN_POINT('Ctrl Pts',(-0.199423466513676,-0.216295910741902,
-1.92987722057055));
#73665=CARTESIAN_POINT('Ctrl Pts',(-0.195609630161698,-0.21981224382198,
-1.92959552699771));
#73666=CARTESIAN_POINT('Ctrl Pts',(-0.191707050176684,-0.223223717710466,
-1.92931383342487));
#73667=CARTESIAN_POINT('Ctrl Pts',(-0.187722398853854,-0.22652580640747,
-1.92903213985203));
#73668=CARTESIAN_POINT('Ctrl Pts',(-0.174999249451123,-0.237069506327294,
-1.92813268112336));
#73669=CARTESIAN_POINT('Ctrl Pts',(-0.161345053520292,-0.246571091634817,
-1.92723322239468));
#73670=CARTESIAN_POINT('Ctrl Pts',(-0.146955739436558,-0.254867908232195,
-1.92633376366601));
#73671=CARTESIAN_POINT('Ctrl Pts',(-0.132594367936121,-0.263148613256254,
-1.92543605159464));
#73672=CARTESIAN_POINT('Ctrl Pts',(-0.117501354938071,-0.270228747692943,
-1.92453833952326));
#73673=CARTESIAN_POINT('Ctrl Pts',(-0.101902268212067,-0.275988347096822,
-1.92364062745189));
#73674=CARTESIAN_POINT('Ctrl Pts',(-0.0863062601140787,-0.281746809789021,
-1.92274309255253));
#73675=CARTESIAN_POINT('Ctrl Pts',(-0.0702050961063534,-0.286184933517517,
-1.92184555765316));
#73676=CARTESIAN_POINT('Ctrl Pts',(-0.0538449204140348,-0.289230642473453,
-1.92094802275379));
#73677=CARTESIAN_POINT('Ctrl Pts',(-0.0374893075748574,-0.292275501981135,
-1.92005073817692));
#73678=CARTESIAN_POINT('Ctrl Pts',(-0.0208756039515256,-0.293928583288013,
-1.91915345360005));
#73679=CARTESIAN_POINT('Ctrl Pts',(-0.00425919539984884,-0.294169167749691,
-1.91825616902317));
#73680=CARTESIAN_POINT('Ctrl Pts',(0.0123962441238195,-0.294410317330201,
-1.9173567767773));
#73681=CARTESIAN_POINT('Ctrl Pts',(0.0290536088470616,-0.293232357194632,
-1.91645738453142));
#73682=CARTESIAN_POINT('Ctrl Pts',(0.0454580461426138,-0.290666829963269,
-1.91555799228555));
#73683=CARTESIAN_POINT('Ctrl Pts',(0.0601090975319945,-0.288375518738729,
-1.91475473144971));
#73684=CARTESIAN_POINT('Ctrl Pts',(0.0745580725981294,-0.284978244983199,
-1.91395147061387));
#73685=CARTESIAN_POINT('Ctrl Pts',(0.0886326038546962,-0.280531462645345,
-1.91314820977803));
#73686=CARTESIAN_POINT('Ctrl Pts',(0.104397103171186,-0.275550742801266,
-1.91224849918258));
#73687=CARTESIAN_POINT('Ctrl Pts',(0.119788857198775,-0.269221776581918,
-1.91134878858713));
#73688=CARTESIAN_POINT('Ctrl Pts',(0.134564982691761,-0.261621683797743,
-1.91044907799168));
#73689=CARTESIAN_POINT('Ctrl Pts',(0.149313219172654,-0.25403593571304,
-1.90955106554366));
#73690=CARTESIAN_POINT('Ctrl Pts',(0.163447411623416,-0.245184124227383,
-1.90865305309565));
#73691=CARTESIAN_POINT('Ctrl Pts',(0.176744624805868,-0.235191363791771,
-1.90775504064764));
#73692=CARTESIAN_POINT('Ctrl Pts',(0.19004026610177,-0.225199784617638,
-1.90685713435523));
#73693=CARTESIAN_POINT('Ctrl Pts',(0.202498465489455,-0.214067955634066,
-1.90595922806282));
#73694=CARTESIAN_POINT('Ctrl Pts',(0.213925481031022,-0.201964176441383,
-1.90506132177041));
#73695=CARTESIAN_POINT('Ctrl Pts',(0.225349814876871,-0.189863237767531,
-1.90416362619895));
#73696=CARTESIAN_POINT('Ctrl Pts',(0.235742912830622,-0.176791383399317,
-1.90326593062748));
#73697=CARTESIAN_POINT('Ctrl Pts',(0.244949280141027,-0.162952416853487,
-1.90236823505601));
#73698=CARTESIAN_POINT('Ctrl Pts',(0.254177861619886,-0.149080058077724,
-1.90146837342273));
#73699=CARTESIAN_POINT('Ctrl Pts',(0.262213577408823,-0.134437564321108,
-1.90056851178945));
#73700=CARTESIAN_POINT('Ctrl Pts',(0.268945203200768,-0.119256520472877,
-1.89966865015617));
#73701=CARTESIAN_POINT('Ctrl Pts',(0.274940688710376,-0.105735607215682,
-1.8988671933388));
#73702=CARTESIAN_POINT('Ctrl Pts',(0.2799022483917,-0.0917882161141617,
-1.89806573652142));
#73703=CARTESIAN_POINT('Ctrl Pts',(0.283784549488893,-0.0775884622310952,
-1.89726427970405));
#73704=CARTESIAN_POINT('Ctrl Pts',(0.288129241563922,-0.061697485045494,
-1.89636736753888));
#73705=CARTESIAN_POINT('Ctrl Pts',(0.291149258518538,-0.0453882981460449,
-1.8954704553737));
#73706=CARTESIAN_POINT('Ctrl Pts',(0.292776608790061,-0.0289049709460469,
-1.89457354320853));
#73707=CARTESIAN_POINT('Ctrl Pts',(0.294400747119029,-0.0124541773075123,
-1.89367840130168));
#73708=CARTESIAN_POINT('Ctrl Pts',(0.294637529594483,0.00416930050062396,
-1.89278325939482));
#73709=CARTESIAN_POINT('Ctrl Pts',(0.293470035720682,0.0207117873227185,
-1.89188811748797));
#73710=CARTESIAN_POINT('Ctrl Pts',(0.292302769717584,0.0372510453928779,
-1.89099315029434));
#73711=CARTESIAN_POINT('Ctrl Pts',(0.289731772884849,0.0537085506239803,
-1.8900981831007));
#73712=CARTESIAN_POINT('Ctrl Pts',(0.285792240943256,0.069831475830259,
-1.88920321590707));
#73713=CARTESIAN_POINT('Ctrl Pts',(0.281853825128017,0.0859498331787345,
-1.88830850227058));
#73714=CARTESIAN_POINT('Ctrl Pts',(0.276547842355274,0.101733029589139,
-1.88741378863409));
#73715=CARTESIAN_POINT('Ctrl Pts',(0.269960107105045,0.116940927702121,
-1.8865190749976));
#73716=CARTESIAN_POINT('Ctrl Pts',(0.263356487414368,0.132185495314217,
-1.88562220401493));
#73717=CARTESIAN_POINT('Ctrl Pts',(0.255465283571869,0.146851272710017,
-1.88472533303226));
#73718=CARTESIAN_POINT('Ctrl Pts',(0.246419722265722,0.160720130906133,
-1.8838284620496));
#73719=CARTESIAN_POINT('Ctrl Pts',(0.23818942255219,0.173339011678179,-1.88301242457642));
#73720=CARTESIAN_POINT('Ctrl Pts',(0.229004329318591,0.185298117620465,
-1.88219638710324));
#73721=CARTESIAN_POINT('Ctrl Pts',(0.218993716856664,0.19645709958488,-1.88138034963006));
#73722=CARTESIAN_POINT('Ctrl Pts',(0.207972888625727,0.208742184431554,
-1.88048196215816));
#73723=CARTESIAN_POINT('Ctrl Pts',(0.19587999043407,0.220136142643117,-1.87958357468625));
#73724=CARTESIAN_POINT('Ctrl Pts',(0.182884332901883,0.230449475545147,
-1.87868518721435));
#73725=CARTESIAN_POINT('Ctrl Pts',(0.169913911101314,0.24074278141118,-1.87778854428404));
#73726=CARTESIAN_POINT('Ctrl Pts',(0.156044781088644,0.249959089577038,
-1.87689190135373));
#73727=CARTESIAN_POINT('Ctrl Pts',(0.141481890185821,0.257946728510844,
-1.87599525842342));
#73728=CARTESIAN_POINT('Ctrl Pts',(0.126921552086915,0.265932967250411,
-1.87509877267025));
#73729=CARTESIAN_POINT('Ctrl Pts',(0.11166836044177,0.272690538754484,-1.87420228691709));
#73730=CARTESIAN_POINT('Ctrl Pts',(0.0959546917773066,0.278112094533701,
-1.87330580116392));
#73731=CARTESIAN_POINT('Ctrl Pts',(0.0802452495683534,0.283532192094294,
-1.87240955653568));
#73732=CARTESIAN_POINT('Ctrl Pts',(0.064076327662526,0.287616739394745,
-1.87151331190743));
#73733=CARTESIAN_POINT('Ctrl Pts',(0.0476969939611587,0.290307831046751,
-1.87061706727919));
#73734=CARTESIAN_POINT('Ctrl Pts',(0.0312784436967652,0.293005365901351,
-1.86971867679846));
#73735=CARTESIAN_POINT('Ctrl Pts',(0.0146492636034039,0.29430267865183,
-1.86882028631773));
#73736=CARTESIAN_POINT('Ctrl Pts',(-0.0019343336099744,0.294193640912725,
-1.867921895837));
#73737=CARTESIAN_POINT('Ctrl Pts',(-0.0168584757494519,0.294095514149513,
-1.86711340374336));
#73738=CARTESIAN_POINT('Ctrl Pts',(-0.0317452363588749,0.292859161753257,
-1.86630491164972));
#73739=CARTESIAN_POINT('Ctrl Pts',(-0.0464121480238433,0.290516010773611,
-1.86549641955607));
#73740=CARTESIAN_POINT('Ctrl Pts',(-0.0627085619740153,0.287912534378286,
-1.86459810352783));
#73741=CARTESIAN_POINT('Ctrl Pts',(-0.0788370821054864,0.283925291532679,
-1.86369978749959));
#73742=CARTESIAN_POINT('Ctrl Pts',(-0.0945467246718159,0.2785938923484,
-1.86280147147135));
#73743=CARTESIAN_POINT('Ctrl Pts',(-0.110225942020353,0.273272818604731,
-1.86190489523195));
#73744=CARTESIAN_POINT('Ctrl Pts',(-0.125487130426198,0.266612944882,-1.86100831899255));
#73745=CARTESIAN_POINT('Ctrl Pts',(-0.140091790292761,0.258704329868228,
-1.86011174275314));
#73746=CARTESIAN_POINT('Ctrl Pts',(-0.154694026867372,0.250797027098856,
-1.859215315279));
#73747=CARTESIAN_POINT('Ctrl Pts',(-0.168639232467807,0.241641723459449,
-1.85831888780486));
#73748=CARTESIAN_POINT('Ctrl Pts',(-0.181711297679933,0.231375548179739,
-1.85742246033071));
#73749=CARTESIAN_POINT('Ctrl Pts',(-0.194779912490204,0.221112082680745,
-1.85652626947067));
#73750=CARTESIAN_POINT('Ctrl Pts',(-0.206975228840357,0.209738825049817,
-1.85563007861063));
#73751=CARTESIAN_POINT('Ctrl Pts',(-0.218113653404721,0.197433721026691,
-1.8547338877506));
#73752=CARTESIAN_POINT('Ctrl Pts',(-0.229278857310927,0.185099032695198,
-1.85383554224101));
#73753=CARTESIAN_POINT('Ctrl Pts',(-0.239381580730588,0.171828630164055,
-1.85293719673143));
#73754=CARTESIAN_POINT('Ctrl Pts',(-0.248277879238832,0.157834516759384,
-1.85203885122185));
#73755=CARTESIAN_POINT('Ctrl Pts',(-0.256287283970732,0.145235510777484,
-1.85123006397526));
#73756=CARTESIAN_POINT('Ctrl Pts',(-0.263319194239916,0.132050695847513,
-1.85042127672867));
#73757=CARTESIAN_POINT('Ctrl Pts',(-0.269301100085867,0.118450654251219,
-1.84961248948208));
#73758=CARTESIAN_POINT('Ctrl Pts',(-0.276605475269511,0.101843939118829,
-1.84862489695806));
#73759=CARTESIAN_POINT('Ctrl Pts',(-0.282384365359411,0.0845267189773186,
-1.84763730443405));
#73760=CARTESIAN_POINT('Ctrl Pts',(-0.286520638407411,0.0667799653085389,
-1.84664971191003));
#73761=CARTESIAN_POINT('Ctrl Pts',(-0.290628292530723,0.0491560016492214,
-1.84566895255097));
#73762=CARTESIAN_POINT('Ctrl Pts',(-0.29311574621684,0.0311089028882957,
-1.84468819319192));
#73763=CARTESIAN_POINT('Ctrl Pts',(-0.29391554915533,0.0129340621894621,
-1.84370743383287));
#73764=CARTESIAN_POINT('Ctrl Pts',(-0.294103062588117,0.00867297910787347,
-1.84347749525012));
#73765=CARTESIAN_POINT('Ctrl Pts',(-0.294198025887685,0.0044049446360574,
-1.84324755666737));
#73766=CARTESIAN_POINT('Ctrl Pts',(-0.294199969536726,0.000133882744709338,
-1.84301761808462));
#73767=CARTESIAN_POINT('',(-0.294199886788754,-0.00025809588161594,-1.74301760920454));
#73768=CARTESIAN_POINT('Ctrl Pts',(-0.293772605452732,0.000133570007895117,
-1.84301761170896));
#73769=CARTESIAN_POINT('Ctrl Pts',(-0.293541789016053,-0.0572970795812668,
-1.83992126094201));
#73770=CARTESIAN_POINT('Ctrl Pts',(-0.249523258593931,-0.213261476144942,
-1.83153026681705));
#73771=CARTESIAN_POINT('Ctrl Pts',(0.0037807816485258,-0.347758850054799,
-1.81784462933411));
#73772=CARTESIAN_POINT('Ctrl Pts',(0.294305938288256,-0.185300865244264,
-1.80196069926011));
#73773=CARTESIAN_POINT('Ctrl Pts',(0.315230872436925,0.146908278444259,
-1.78607676918614));
#73774=CARTESIAN_POINT('Ctrl Pts',(0.0473846120171572,0.344538303459251,
-1.77019283911214));
#73775=CARTESIAN_POINT('Ctrl Pts',(-0.233870088077291,0.23792327169595,
-1.75583978661975));
#73776=CARTESIAN_POINT('Ctrl Pts',(-0.29345314308191,0.0693924262310005,
-1.74678137748536));
#73777=CARTESIAN_POINT('Ctrl Pts',(-0.294038510274165,-0.000257907963998623,
-1.74301761170896));
#73778=CARTESIAN_POINT('',(-0.294199999759564,1.18942342969988E-5,-1.64301761170595));
#73779=CARTESIAN_POINT('Ctrl Pts',(-0.294199886788754,-0.00025809588161594,
-1.74301760920454));
#73780=CARTESIAN_POINT('Ctrl Pts',(-0.294182004219665,-0.0206421863546536,
-1.74191668866673));
#73781=CARTESIAN_POINT('Ctrl Pts',(-0.292041631426675,-0.0409317727345108,
-1.74081576812892));
#73782=CARTESIAN_POINT('Ctrl Pts',(-0.287860331974439,-0.060745940403997,
-1.73971484759111));
#73783=CARTESIAN_POINT('Ctrl Pts',(-0.286227357023594,-0.0684842140784187,
-1.73928489138213));
#73784=CARTESIAN_POINT('Ctrl Pts',(-0.284283610133334,-0.0761502155981999,
-1.73885493517315));
#73785=CARTESIAN_POINT('Ctrl Pts',(-0.282035889300632,-0.0837221425096234,
-1.73842497896416));
#73786=CARTESIAN_POINT('Ctrl Pts',(-0.277340653829632,-0.0995390443690926,
-1.73752684890547));
#73787=CARTESIAN_POINT('Ctrl Pts',(-0.271295716406367,-0.115010317437608,
-1.73662871884677));
#73788=CARTESIAN_POINT('Ctrl Pts',(-0.263972782043712,-0.129892302851643,
-1.73573058878808));
#73789=CARTESIAN_POINT('Ctrl Pts',(-0.256664082356794,-0.144745359939108,
-1.73483420455825));
#73790=CARTESIAN_POINT('Ctrl Pts',(-0.248082602783536,-0.159010671921717,
-1.73393782032842));
#73791=CARTESIAN_POINT('Ctrl Pts',(-0.238348459422095,-0.172463479876506,
-1.73304143609858));
#73792=CARTESIAN_POINT('Ctrl Pts',(-0.228616002021185,-0.18591395779542,
-1.73214520712314));
#73793=CARTESIAN_POINT('Ctrl Pts',(-0.217731696690339,-0.198551540690138,
-1.73124897814769));
#73794=CARTESIAN_POINT('Ctrl Pts',(-0.205859437392401,-0.21017976124376,
-1.73035274917224));
#73795=CARTESIAN_POINT('Ctrl Pts',(-0.193990364349679,-0.221804861036838,
-1.72945676072508));
#73796=CARTESIAN_POINT('Ctrl Pts',(-0.181134436886301,-0.232420589967314,
-1.72856077227793));
#73797=CARTESIAN_POINT('Ctrl Pts',(-0.16749181297899,-0.241868006534579,
-1.72766478383077));
#73798=CARTESIAN_POINT('Ctrl Pts',(-0.153816416765014,-0.251338117682815,
-1.72676664304046));
#73799=CARTESIAN_POINT('Ctrl Pts',(-0.139351218207657,-0.259633880163493,
-1.72586850225015));
#73800=CARTESIAN_POINT('Ctrl Pts',(-0.12432501040221,-0.266640079111319,
-1.72497036145984));
#73801=CARTESIAN_POINT('Ctrl Pts',(-0.110777262324531,-0.272956923624333,
-1.72416059060329));
#73802=CARTESIAN_POINT('Ctrl Pts',(-0.0967742142943387,-0.278225957041598,
-1.72335081974673));
#73803=CARTESIAN_POINT('Ctrl Pts',(-0.0824951304211087,-0.282397226361741,
-1.72254104889018));
#73804=CARTESIAN_POINT('Ctrl Pts',(-0.0666579885938232,-0.287023642482648,
-1.72164292012949));
#73805=CARTESIAN_POINT('Ctrl Pts',(-0.050379814436038,-0.290328456021256,
-1.72074479136879));
#73806=CARTESIAN_POINT('Ctrl Pts',(-0.0339042395189861,-0.292239871582642,
-1.7198466626081));
#73807=CARTESIAN_POINT('Ctrl Pts',(-0.0174606908866978,-0.294147571611225,
-1.718950279688));
#73808=CARTESIAN_POINT('Ctrl Pts',(-0.000821272637496952,-0.294667094103919,
-1.7180538967679));
#73809=CARTESIAN_POINT('Ctrl Pts',(0.0157600296568049,-0.293777571412824,
-1.7171575138478));
#73810=CARTESIAN_POINT('Ctrl Pts',(0.0323384600825974,-0.292888202786358,
-1.71626128618052));
#73811=CARTESIAN_POINT('Ctrl Pts',(0.0488580037869914,-0.290590262706318,
-1.71536505851323));
#73812=CARTESIAN_POINT('Ctrl Pts',(0.0650647250257694,-0.286915007549834,
-1.71446883084595));
#73813=CARTESIAN_POINT('Ctrl Pts',(0.0812670967009878,-0.28324073875917,
-1.71357284370845));
#73814=CARTESIAN_POINT('Ctrl Pts',(0.0971560428253877,-0.278190074333859,
-1.71267685657095));
#73815=CARTESIAN_POINT('Ctrl Pts',(0.112489510217748,-0.271845084728364,
-1.71178086943345));
#73816=CARTESIAN_POINT('Ctrl Pts',(0.127859812149806,-0.265484852988423,
-1.71088272992735));
#73817=CARTESIAN_POINT('Ctrl Pts',(0.142671245731315,-0.257824414314113,
-1.70998459042125));
#73818=CARTESIAN_POINT('Ctrl Pts',(0.156702986152284,-0.248993602590422,
-1.70908645091515));
#73819=CARTESIAN_POINT('Ctrl Pts',(0.169354234344561,-0.241031597343466,
-1.70827667354883));
#73820=CARTESIAN_POINT('Ctrl Pts',(0.18137165371886,-0.232119060944684,
-1.70746689618251));
#73821=CARTESIAN_POINT('Ctrl Pts',(0.192616104667109,-0.222379576901453,
-1.70665711881619));
#73822=CARTESIAN_POINT('Ctrl Pts',(0.20508738163451,-0.211577466279802,
-1.70575899067603));
#73823=CARTESIAN_POINT('Ctrl Pts',(0.21668701521377,-0.199688445134471,
-1.70486086253587));
#73824=CARTESIAN_POINT('Ctrl Pts',(0.227222627668846,-0.186878349402131,
-1.70396273439571));
#73825=CARTESIAN_POINT('Ctrl Pts',(0.237737760048888,-0.174093155090843,
-1.70306635211814));
#73826=CARTESIAN_POINT('Ctrl Pts',(0.247192428763082,-0.160391002328869,
-1.70216996984057));
#73827=CARTESIAN_POINT('Ctrl Pts',(0.255431444012423,-0.145974029915354,
-1.701273587563));
#73828=CARTESIAN_POINT('Ctrl Pts',(0.263669032044348,-0.131559554906379,
-1.70037736056278));
#73829=CARTESIAN_POINT('Ctrl Pts',(0.270690947064961,-0.116431164783314,
-1.69948113356255));
#73830=CARTESIAN_POINT('Ctrl Pts',(0.276385831152967,-0.100819206195466,
-1.69858490656233));
#73831=CARTESIAN_POINT('Ctrl Pts',(0.282079186752439,-0.0852114378069836,
-1.69768892010654));
#73832=CARTESIAN_POINT('Ctrl Pts',(0.286445957303159,-0.0691211061119678,
-1.69679293365075));
#73833=CARTESIAN_POINT('Ctrl Pts',(0.289423928892626,-0.0527961114510928,
-1.69589694719497));
#73834=CARTESIAN_POINT('Ctrl Pts',(0.292409054230803,-0.0364319005297542,
-1.69499880838085));
#73835=CARTESIAN_POINT('Ctrl Pts',(0.293998600557534,-0.0198326875387263,
-1.69410066956674));
#73836=CARTESIAN_POINT('Ctrl Pts',(0.294181999376833,-0.00325441894184345,
-1.69320253075262));
#73837=CARTESIAN_POINT('Ctrl Pts',(0.29434735557396,0.0116928934815336,
-1.69239275008248));
#73838=CARTESIAN_POINT('Ctrl Pts',(0.293370361575628,0.0266226975162987,
-1.69158296941234));
#73839=CARTESIAN_POINT('Ctrl Pts',(0.291279467561646,0.0413510795143722,
-1.6907731887422));
#73840=CARTESIAN_POINT('Ctrl Pts',(0.288960454152482,0.0576863481221683,
-1.68987505989398));
#73841=CARTESIAN_POINT('Ctrl Pts',(0.285255596600586,0.0738781613795155,
-1.68897693104575));
#73842=CARTESIAN_POINT('Ctrl Pts',(0.280200000512142,0.0896749670364913,
-1.68807880219753));
#73843=CARTESIAN_POINT('Ctrl Pts',(0.27515423185183,0.105441065736345,-1.6871824191962));
#73844=CARTESIAN_POINT('Ctrl Pts',(0.268763111840153,0.120812915685593,
-1.68628603619486));
#73845=CARTESIAN_POINT('Ctrl Pts',(0.26111240966032,0.135550542313122,-1.68538965319353));
#73846=CARTESIAN_POINT('Ctrl Pts',(0.253463032670157,0.1502856162141,-1.68449342545605));
#73847=CARTESIAN_POINT('Ctrl Pts',(0.24455482305236,0.164385960117459,-1.68359719771857));
#73848=CARTESIAN_POINT('Ctrl Pts',(0.234521011344578,0.177633147914223,
-1.68270096998109));
#73849=CARTESIAN_POINT('Ctrl Pts',(0.224489892579616,0.190876780340376,
-1.68180498277932));
#73850=CARTESIAN_POINT('Ctrl Pts',(0.213334258091221,0.203267086599783,
-1.68090899557755));
#73851=CARTESIAN_POINT('Ctrl Pts',(0.201228725053308,0.214617427562209,
-1.68001300837578));
#73852=CARTESIAN_POINT('Ctrl Pts',(0.189094111877945,0.225995034525584,
-1.67911486881683));
#73853=CARTESIAN_POINT('Ctrl Pts',(0.17600564058815,0.236327162035444,-1.67821672925788));
#73854=CARTESIAN_POINT('Ctrl Pts',(0.162172680545946,0.245466212918484,
-1.67731858969893));
#73855=CARTESIAN_POINT('Ctrl Pts',(0.149700662234219,0.253706127558396,
-1.67650881268869));
#73856=CARTESIAN_POINT('Ctrl Pts',(0.136624244377117,0.260976533262224,
-1.67569903567845));
#73857=CARTESIAN_POINT('Ctrl Pts',(0.123113404217359,0.267201664856365,
-1.67488925866821));
#73858=CARTESIAN_POINT('Ctrl Pts',(0.108128449066995,0.274105996240668,
-1.67399113005173));
#73859=CARTESIAN_POINT('Ctrl Pts',(0.0925129675321822,0.279767919567134,
-1.67309300143525));
#73860=CARTESIAN_POINT('Ctrl Pts',(0.0764973896053433,0.28408060367362,
-1.67219487281876));
#73861=CARTESIAN_POINT('Ctrl Pts',(0.0605129439601607,0.288384904461258,
-1.67129849005205));
#73862=CARTESIAN_POINT('Ctrl Pts',(0.0441306838838317,0.291344904687799,
-1.67040210728534));
#73863=CARTESIAN_POINT('Ctrl Pts',(0.0275987676766963,0.292902625496474,
-1.66950572451862));
#73864=CARTESIAN_POINT('Ctrl Pts',(0.011069715005662,0.294460076488286,
-1.66860949701669));
#73865=CARTESIAN_POINT('Ctrl Pts',(-0.00560816175754345,0.294615603373687,
-1.66771326951477));
#73866=CARTESIAN_POINT('Ctrl Pts',(-0.0221790909419616,0.293362792332273,
-1.66681704201284));
#73867=CARTESIAN_POINT('Ctrl Pts',(-0.0387455726889244,0.292110317530226,
-1.66592105504756));
#73868=CARTESIAN_POINT('Ctrl Pts',(-0.0552043751603669,0.289450325616551,
-1.66502506808228));
#73869=CARTESIAN_POINT('Ctrl Pts',(-0.0713040100637426,0.285428411600579,
-1.664129081117));
#73870=CARTESIAN_POINT('Ctrl Pts',(-0.0874423198831428,0.281396836049563,
-1.66323094179107));
#73871=CARTESIAN_POINT('Ctrl Pts',(-0.103218974013307,0.275997022269512,
-1.66233280246514));
#73872=CARTESIAN_POINT('Ctrl Pts',(-0.118396460284086,0.269324930506255,
-1.66143466313921));
#73873=CARTESIAN_POINT('Ctrl Pts',(-0.13208074832238,0.263309255454575,
-1.66062488495755));
#73874=CARTESIAN_POINT('Ctrl Pts',(-0.145277828378794,0.256260196441748,
-1.65981510677589));
#73875=CARTESIAN_POINT('Ctrl Pts',(-0.157831904283623,0.248279540015292,
-1.65900532859422));
#73876=CARTESIAN_POINT('Ctrl Pts',(-0.171755685256082,0.239428158763435,
-1.65810720004034));
#73877=CARTESIAN_POINT('Ctrl Pts',(-0.184977075898487,0.229373536686353,
-1.65720907148646));
#73878=CARTESIAN_POINT('Ctrl Pts',(-0.197281409381263,0.218251427286381,
-1.65631094293258));
#73879=CARTESIAN_POINT('Ctrl Pts',(-0.209561824739444,0.207150937911481,
-1.65541456023114));
#73880=CARTESIAN_POINT('Ctrl Pts',(-0.220928096626076,0.194987555580086,
-1.6545181775297));
#73881=CARTESIAN_POINT('Ctrl Pts',(-0.231197005359185,0.181938409119529,
-1.65362179482826));
#73882=CARTESIAN_POINT('Ctrl Pts',(-0.241464135351528,0.168891522981793,
-1.65272556739477));
#73883=CARTESIAN_POINT('Ctrl Pts',(-0.250633749860754,0.154959764532739,
-1.65182933996128));
#73884=CARTESIAN_POINT('Ctrl Pts',(-0.258561838122118,0.140354607572789,
-1.6509331125278));
#73885=CARTESIAN_POINT('Ctrl Pts',(-0.266487798563621,0.125753370491381,
-1.65003712563282));
#73886=CARTESIAN_POINT('Ctrl Pts',(-0.273172526015679,0.11047979467552,
-1.64914113873785));
#73887=CARTESIAN_POINT('Ctrl Pts',(-0.278518039277829,0.0947699414204417,
-1.64824515184287));
#73888=CARTESIAN_POINT('Ctrl Pts',(-0.283876393646943,0.079022349617882,
-1.6473470125889));
#73889=CARTESIAN_POINT('Ctrl Pts',(-0.287888877285267,0.0628371482372673,
-1.64644887333492));
#73890=CARTESIAN_POINT('Ctrl Pts',(-0.29050741046383,0.0464659495286565,
-1.64555073408095));
#73891=CARTESIAN_POINT('Ctrl Pts',(-0.292868327118073,0.0317053820485487,
-1.64474095556071));
#73892=CARTESIAN_POINT('Ctrl Pts',(-0.294096737055979,0.0167941996829556,
-1.64393117704048));
#73893=CARTESIAN_POINT('Ctrl Pts',(-0.294193744601594,0.00191849870784247,
-1.64312139852024));
#73894=CARTESIAN_POINT('Ctrl Pts',(-0.294197888987406,0.00128297449510215,
-1.64308680291648));
#73895=CARTESIAN_POINT('Ctrl Pts',(-0.294199974065043,0.000647436838625386,
-1.64305220731272));
#73896=CARTESIAN_POINT('Ctrl Pts',(-0.294199999759561,1.18942896398017E-5,
-1.64301761170896));
#73897=CARTESIAN_POINT('',(-0.294199892933704,0.000250993619749801,-1.54301761464762));
#73898=CARTESIAN_POINT('Ctrl Pts',(-0.294199999759564,1.18942342971948E-5,
-1.64301761170595));
#73899=CARTESIAN_POINT('Ctrl Pts',(-0.29420066603068,-0.0164681041648284,
-1.64212052700963));
#73900=CARTESIAN_POINT('Ctrl Pts',(-0.292812289007885,-0.0330014442052797,
-1.64122344231331));
#73901=CARTESIAN_POINT('Ctrl Pts',(-0.290034021661079,-0.0493346356944172,
-1.640326357617));
#73902=CARTESIAN_POINT('Ctrl Pts',(-0.287261151236874,-0.0656360991461516,
-1.63943101555235));
#73903=CARTESIAN_POINT('Ctrl Pts',(-0.283103815236798,-0.081737401346229,
-1.63853567348771));
#73904=CARTESIAN_POINT('Ctrl Pts',(-0.277612958384786,-0.0973893491961362,
-1.63764033142306));
#73905=CARTESIAN_POINT('Ctrl Pts',(-0.272123042715187,-0.113038614160944,
-1.63674514282813));
#73906=CARTESIAN_POINT('Ctrl Pts',(-0.26530027190556,-0.128237913644052,
-1.63584995423319));
#73907=CARTESIAN_POINT('Ctrl Pts',(-0.257245611679783,-0.142752706704617,
-1.63495476563826));
#73908=CARTESIAN_POINT('Ctrl Pts',(-0.249193019905193,-0.157263772340298,
-1.63405980692936));
#73909=CARTESIAN_POINT('Ctrl Pts',(-0.239909561963817,-0.17108999201756,
-1.63316484822046));
#73910=CARTESIAN_POINT('Ctrl Pts',(-0.229541638621305,-0.184022488134049,
-1.63226988951156));
#73911=CARTESIAN_POINT('Ctrl Pts',(-0.219148990372253,-0.196985825022335,
-1.63137279654977));
#73912=CARTESIAN_POINT('Ctrl Pts',(-0.207667232146339,-0.209050577778784,
-1.63047570358797));
#73913=CARTESIAN_POINT('Ctrl Pts',(-0.195282607322232,-0.220041685317648,
-1.62957861062618));
#73914=CARTESIAN_POINT('Ctrl Pts',(-0.184509228273474,-0.22960284436474,
-1.62879822989954));
#73915=CARTESIAN_POINT('Ctrl Pts',(-0.173053501126384,-0.238351936559686,
-1.62801784917289));
#73916=CARTESIAN_POINT('Ctrl Pts',(-0.161056510020361,-0.246200001178029,
-1.62723746844625));
#73917=CARTESIAN_POINT('Ctrl Pts',(-0.147249350738978,-0.255232222447381,
-1.62633933983237));
#73918=CARTESIAN_POINT('Ctrl Pts',(-0.132635872021187,-0.263128226214613,
-1.62544121121848));
#73919=CARTESIAN_POINT('Ctrl Pts',(-0.11742829531282,-0.269748467020528,
-1.6245430826046));
#73920=CARTESIAN_POINT('Ctrl Pts',(-0.102250280248761,-0.276355838898824,
-1.62364669984142));
#73921=CARTESIAN_POINT('Ctrl Pts',(-0.0864811503842343,-0.281691997354744,
-1.62275031707825));
#73922=CARTESIAN_POINT('Ctrl Pts',(-0.0703578445262541,-0.285663112273215,
-1.62185393431508));
#73923=CARTESIAN_POINT('Ctrl Pts',(-0.0542373314533323,-0.289633539338307,
-1.6209577068181));
#73924=CARTESIAN_POINT('Ctrl Pts',(-0.0377635176204008,-0.292239152005272,
-1.62006147932112));
#73925=CARTESIAN_POINT('Ctrl Pts',(-0.0211884529455285,-0.293436005735109,
-1.61916525182415));
#73926=CARTESIAN_POINT('Ctrl Pts',(-0.00461783683253826,-0.294632538242799,
-1.6182692648646));
#73927=CARTESIAN_POINT('Ctrl Pts',(0.0120531857089837,-0.294421016148064,
-1.61737327790506));
#73928=CARTESIAN_POINT('Ctrl Pts',(0.0285691559034124,-0.292809568373314,
-1.61647729094551));
#73929=CARTESIAN_POINT('Ctrl Pts',(0.0451248011221824,-0.291194249543522,
-1.61557915162652));
#73930=CARTESIAN_POINT('Ctrl Pts',(0.0615238614247141,-0.288172391760294,
-1.61468101230753));
#73931=CARTESIAN_POINT('Ctrl Pts',(0.0775172982348087,-0.283803996579287,
-1.61378287298854));
#73932=CARTESIAN_POINT('Ctrl Pts',(0.0919372621366972,-0.279865374657852,
-1.61297309478312));
#73933=CARTESIAN_POINT('Ctrl Pts',(0.106027226741348,-0.274832972739917,
-1.61216331657769));
#73934=CARTESIAN_POINT('Ctrl Pts',(0.119618125126485,-0.26878456827211,
-1.61135353837226));
#73935=CARTESIAN_POINT('Ctrl Pts',(0.134691850967059,-0.262076255978323,
-1.61045540976337));
#73936=CARTESIAN_POINT('Ctrl Pts',(0.14924770316629,-0.254074518741827,
-1.60955728115447));
#73937=CARTESIAN_POINT('Ctrl Pts',(0.163053390356407,-0.244882077525656,
-1.60865915254558));
#73938=CARTESIAN_POINT('Ctrl Pts',(0.176832240996848,-0.23570750527913,
-1.6077627697877));
#73939=CARTESIAN_POINT('Ctrl Pts',(0.18986313325126,-0.225347201834048,
-1.60686638702982));
#73940=CARTESIAN_POINT('Ctrl Pts',(0.201938798754428,-0.213949436918209,
-1.60597000427194));
#73941=CARTESIAN_POINT('Ctrl Pts',(0.214012372575882,-0.202553646261796,
-1.60507377678066));
#73942=CARTESIAN_POINT('Ctrl Pts',(0.225130437864743,-0.190121253866431,
-1.60417754928937));
#73943=CARTESIAN_POINT('Ctrl Pts',(0.235119460212498,-0.176840265294371,
-1.60328132179808));
#73944=CARTESIAN_POINT('Ctrl Pts',(0.245105801615888,-0.163562841194412,
-1.60238533484446));
#73945=CARTESIAN_POINT('Ctrl Pts',(0.253963234353235,-0.149437912289678,
-1.60148934789083));
#73946=CARTESIAN_POINT('Ctrl Pts',(0.261560138938136,-0.134684571197532,
-1.6005933609372));
#73947=CARTESIAN_POINT('Ctrl Pts',(0.269175292971096,-0.119895789311185,
-1.59969522162438));
#73948=CARTESIAN_POINT('Ctrl Pts',(0.275523530465425,-0.104476299009142,
-1.59879708231157));
#73949=CARTESIAN_POINT('Ctrl Pts',(0.280520305136338,-0.0886679108032643,
-1.59789894299876));
#73950=CARTESIAN_POINT('Ctrl Pts',(0.285025485244197,-0.0744147893853603,
-1.59708916476526));
#73951=CARTESIAN_POINT('Ctrl Pts',(0.288432605244778,-0.0598462025816209,
-1.59627938653177));
#73952=CARTESIAN_POINT('Ctrl Pts',(0.290715399914207,-0.0451463869287753,
-1.59546960829827));
#73953=CARTESIAN_POINT('Ctrl Pts',(0.293247257584567,-0.0288427563342436,
-1.59457147967584));
#73954=CARTESIAN_POINT('Ctrl Pts',(0.294411451733629,-0.0122733479877298,
-1.5936733510534));
#73955=CARTESIAN_POINT('Ctrl Pts',(0.294168413866012,0.00431094926375149,
-1.59277522243096));
#73956=CARTESIAN_POINT('Ctrl Pts',(0.293925848433877,0.0208630086975991,
-1.59187883965921));
#73957=CARTESIAN_POINT('Ctrl Pts',(0.292281426022063,0.0374291163790788,
-1.59098245688746));
#73958=CARTESIAN_POINT('Ctrl Pts',(0.289247418934938,0.0537547266710246,
-1.59008607411571));
#73959=CARTESIAN_POINT('Ctrl Pts',(0.28621393738113,0.0700775091343299,
-1.58918984661024));
#73960=CARTESIAN_POINT('Ctrl Pts',(0.281791440950735,0.0861590914506403,
-1.58829361910478));
#73961=CARTESIAN_POINT('Ctrl Pts',(0.276043878650335,0.101751742293089,
-1.58739739159931));
#73962=CARTESIAN_POINT('Ctrl Pts',(0.270297858931542,0.117340208241988,
-1.58650140463131));
#73963=CARTESIAN_POINT('Ctrl Pts',(0.263227763301797,0.132439264070395,
-1.58560541766331));
#73964=CARTESIAN_POINT('Ctrl Pts',(0.254946382893199,0.146819555406201,
-1.58470943069531));
#73965=CARTESIAN_POINT('Ctrl Pts',(0.246645108774087,0.161234391387805,
-1.5838112913681));
#73966=CARTESIAN_POINT('Ctrl Pts',(0.2371271578167,0.174926338578149,-1.5829131520409));
#73967=CARTESIAN_POINT('Ctrl Pts',(0.226549925487755,0.187693290400836,
-1.58201501271369));
#73968=CARTESIAN_POINT('Ctrl Pts',(0.217013307385266,0.199204197987944,
-1.58120523455056));
#73969=CARTESIAN_POINT('Ctrl Pts',(0.206616457308168,0.209963271222389,
-1.58039545638742));
#73970=CARTESIAN_POINT('Ctrl Pts',(0.19549997222728,0.219848586211358,-1.57958567822428));
#73971=CARTESIAN_POINT('Ctrl Pts',(0.18317062844361,0.230812433688506,-1.57868754960816));
#73972=CARTESIAN_POINT('Ctrl Pts',(0.169876692927069,0.240770943386101,
-1.57778942099204));
#73973=CARTESIAN_POINT('Ctrl Pts',(0.155807567163121,0.249554887779642,
-1.57689129237592));
#73974=CARTESIAN_POINT('Ctrl Pts',(0.141765790037109,0.258321757273228,
-1.5759949096106));
#73975=CARTESIAN_POINT('Ctrl Pts',(0.126952442259669,0.265918123021017,
-1.57509852684527));
#73976=CARTESIAN_POINT('Ctrl Pts',(0.111588094637542,0.272216342520362,
-1.57420214407994));
#73977=CARTESIAN_POINT('Ctrl Pts',(0.0962264083407792,0.27851347107776,
-1.57330591658096));
#73978=CARTESIAN_POINT('Ctrl Pts',(0.0803146216090893,0.283512551370949,
-1.57240968908198));
#73979=CARTESIAN_POINT('Ctrl Pts',(0.0640955857448739,0.287133063035279,
-1.571513461583));
#73980=CARTESIAN_POINT('Ctrl Pts',(0.0478809028898535,0.290752602994466,
-1.57061747462154));
#73981=CARTESIAN_POINT('Ctrl Pts',(0.0313599096841066,0.292994146872166,
-1.56972148766007));
#73982=CARTESIAN_POINT('Ctrl Pts',(0.0147864844490515,0.293828180877257,
-1.56882550069861));
#73983=CARTESIAN_POINT('Ctrl Pts',(-0.00182675382671472,0.294664218416882,
-1.56792736137788));
#73984=CARTESIAN_POINT('Ctrl Pts',(-0.0184918804152472,0.294085979362492,
-1.56702922205715));
#73985=CARTESIAN_POINT('Ctrl Pts',(-0.0349537417671605,0.292116202796892,
-1.56613108273642));
#73986=CARTESIAN_POINT('Ctrl Pts',(-0.0497960452610043,0.290340217628707,
-1.56532130454104));
#73987=CARTESIAN_POINT('Ctrl Pts',(-0.0644727288162011,0.287433823600362,
-1.56451152634567));
#73988=CARTESIAN_POINT('Ctrl Pts',(-0.0788051284892848,0.28344909899978,
-1.5637017481503));
#73989=CARTESIAN_POINT('Ctrl Pts',(-0.0947012570288975,0.279029623134566,
-1.5628036195343));
#73990=CARTESIAN_POINT('Ctrl Pts',(-0.110275281788735,0.273254643519861,
-1.56190549091831));
#73991=CARTESIAN_POINT('Ctrl Pts',(-0.125282334394243,0.266191616488441,
-1.56100736230232));
#73992=CARTESIAN_POINT('Ctrl Pts',(-0.140260215147669,0.259142319107021,
-1.56011097953715));
#73993=CARTESIAN_POINT('Ctrl Pts',(-0.154672575358626,0.250810217452463,
-1.55921459677198));
#73994=CARTESIAN_POINT('Ctrl Pts',(-0.168292601773028,0.241311500323679,
-1.55831821400681));
#73995=CARTESIAN_POINT('Ctrl Pts',(-0.181910269002808,0.231814428509427,
-1.55742198650804));
#73996=CARTESIAN_POINT('Ctrl Pts',(-0.194735197328667,0.221151550187561,
-1.55652575900927));
#73997=CARTESIAN_POINT('Ctrl Pts',(-0.206568099474672,0.209483317425092,
-1.5556295315105));
#73998=CARTESIAN_POINT('Ctrl Pts',(-0.218397825800741,0.197818216287121,
-1.55473354454926));
#73999=CARTESIAN_POINT('Ctrl Pts',(-0.229235498322907,0.185148859962291,
-1.55383755758803));
#74000=CARTESIAN_POINT('Ctrl Pts',(-0.238918719262039,0.171672611636763,
-1.5529415706268));
#74001=CARTESIAN_POINT('Ctrl Pts',(-0.248625201443618,0.158163990376493,
-1.55204343130634));
#74002=CARTESIAN_POINT('Ctrl Pts',(-0.257171250626507,0.143845266693222,
-1.55114529198588));
#74003=CARTESIAN_POINT('Ctrl Pts',(-0.264437691095471,0.128943194966219,
-1.55024715266542));
#74004=CARTESIAN_POINT('Ctrl Pts',(-0.270989241531935,0.115507225189233,
-1.54943737446905));
#74005=CARTESIAN_POINT('Ctrl Pts',(-0.276501037815482,0.101597794258325,
-1.54862759627268));
#74006=CARTESIAN_POINT('Ctrl Pts',(-0.280920015911495,0.0873932758299257,
-1.54781781807631));
#74007=CARTESIAN_POINT('Ctrl Pts',(-0.286835222818169,0.0683792269507376,
-1.54673385579455));
#74008=CARTESIAN_POINT('Ctrl Pts',(-0.290823615892637,0.0487388113954715,
-1.54564989351278));
#74009=CARTESIAN_POINT('Ctrl Pts',(-0.292784009127529,0.0288299150052643,
-1.54456593123101));
#74010=CARTESIAN_POINT('Ctrl Pts',(-0.293717408566058,0.0193507184942863,
-1.54404982570322));
#74011=CARTESIAN_POINT('Ctrl Pts',(-0.294191736941937,0.00981096533160225,
-1.54353372017542));
#74012=CARTESIAN_POINT('Ctrl Pts',(-0.294199892933704,0.000250993619749801,
-1.54301761464762));
#74013=CARTESIAN_POINT('',(-0.29418954747297,-0.000149745958145899,-1.44301760831983));
#74014=CARTESIAN_POINT('Ctrl Pts',(-0.294003481567088,0.000250771656118091,
-1.54301761170896));
#74015=CARTESIAN_POINT('Ctrl Pts',(-0.293449673493068,-0.0681397340478563,
-1.53932303714008));
#74016=CARTESIAN_POINT('Ctrl Pts',(-0.23560419086501,-0.235384398412292,
-1.5303338192132));
#74017=CARTESIAN_POINT('Ctrl Pts',(0.0428872820869395,-0.345127335346264,
-1.51604995792834));
#74018=CARTESIAN_POINT('Ctrl Pts',(0.313287870803062,-0.151006313006851,
-1.50016602785434));
#74019=CARTESIAN_POINT('Ctrl Pts',(0.296698023090229,0.181445528060777,
-1.48428209778035));
#74020=CARTESIAN_POINT('Ctrl Pts',(0.00831503218110857,0.347682407955339,
-1.46839816770636));
#74021=CARTESIAN_POINT('Ctrl Pts',(-0.248008816545998,0.21583064906809,
-1.45464333901591));
#74022=CARTESIAN_POINT('Ctrl Pts',(-0.293521943642023,0.0585543023250566,
-1.44618315368343));
#74023=CARTESIAN_POINT('Ctrl Pts',(-0.293791839002738,-0.000149480667589675,
-1.44301761170896));
#74024=CARTESIAN_POINT('',(-0.294199947499254,-0.000175759597173832,-1.34301761171257));
#74025=CARTESIAN_POINT('Ctrl Pts',(-0.294199961886584,-0.000149752905057487,
-1.44301760823108));
#74026=CARTESIAN_POINT('Ctrl Pts',(-0.294190615311062,-0.0185117483628317,
-1.44202882723622));
#74027=CARTESIAN_POINT('Ctrl Pts',(-0.292458066504274,-0.0368137300704296,
-1.44104004624135));
#74028=CARTESIAN_POINT('Ctrl Pts',(-0.289060276751152,-0.0547521360729214,
-1.44005126524649));
#74029=CARTESIAN_POINT('Ctrl Pts',(-0.285636324511361,-0.0728286651913199,
-1.43905487078185));
#74030=CARTESIAN_POINT('Ctrl Pts',(-0.280521610325117,-0.0905355406692512,
-1.43805847631721));
#74031=CARTESIAN_POINT('Ctrl Pts',(-0.273824486776581,-0.10758155251502,
-1.43706208185257));
#74032=CARTESIAN_POINT('Ctrl Pts',(-0.272857116959456,-0.110043773383792,
-1.43691815708784));
#74033=CARTESIAN_POINT('Ctrl Pts',(-0.271856810329458,-0.11249224522753,
-1.43677423232312));
#74034=CARTESIAN_POINT('Ctrl Pts',(-0.270823972658315,-0.114926132074338,
-1.4366303075584));
#74035=CARTESIAN_POINT('Ctrl Pts',(-0.264378792282731,-0.130114230049183,
-1.43573217894141));
#74036=CARTESIAN_POINT('Ctrl Pts',(-0.256631377181344,-0.144807024088557,
-1.43483405032443));
#74037=CARTESIAN_POINT('Ctrl Pts',(-0.247680393466925,-0.158770471725914,
-1.43393592170744));
#74038=CARTESIAN_POINT('Ctrl Pts',(-0.238746809356209,-0.172706776150528,
-1.43303953894125));
#74039=CARTESIAN_POINT('Ctrl Pts',(-0.22861466703219,-0.18591585399038,
-1.43214315617505));
#74040=CARTESIAN_POINT('Ctrl Pts',(-0.217428609611005,-0.198187889949475,
-1.43124677340886));
#74041=CARTESIAN_POINT('Ctrl Pts',(-0.206244489775594,-0.210457800215719,
-1.43035054590903));
#74042=CARTESIAN_POINT('Ctrl Pts',(-0.194007309544396,-0.221790371912111,
-1.42945431840921));
#74043=CARTESIAN_POINT('Ctrl Pts',(-0.180902028460652,-0.232008827631238,
-1.42855809090938));
#74044=CARTESIAN_POINT('Ctrl Pts',(-0.167800264688979,-0.242224540830199,
-1.42766210394707));
#74045=CARTESIAN_POINT('Ctrl Pts',(-0.153831493606305,-0.251326253328425,
-1.42676611698477));
#74046=CARTESIAN_POINT('Ctrl Pts',(-0.13921248597049,-0.259178555729281,
-1.42587013002246));
#74047=CARTESIAN_POINT('Ctrl Pts',(-0.124558360238736,-0.267049721100588,
-1.42497199070091));
#74048=CARTESIAN_POINT('Ctrl Pts',(-0.109251590984753,-0.273665128883298,
-1.42407385137937));
#74049=CARTESIAN_POINT('Ctrl Pts',(-0.093532481983476,-0.278936040722619,
-1.42317571205783));
#74050=CARTESIAN_POINT('Ctrl Pts',(-0.0793598571488876,-0.283688387438252,
-1.42236593386669));
#74051=CARTESIAN_POINT('Ctrl Pts',(-0.0648527204541803,-0.287348325831189,
-1.42155615567554));
#74052=CARTESIAN_POINT('Ctrl Pts',(-0.0501948238207512,-0.289886390956188,
-1.4207463774844));
#74053=CARTESIAN_POINT('Ctrl Pts',(-0.0339376850445119,-0.29270137034867,
-1.41984824886741));
#74054=CARTESIAN_POINT('Ctrl Pts',(-0.0173910263376684,-0.294153514652302,
-1.41895012025042));
#74055=CARTESIAN_POINT('Ctrl Pts',(-0.000805010551057393,-0.294198898634942,
-1.41805199163343));
#74056=CARTESIAN_POINT('Ctrl Pts',(0.0157487640751522,-0.29424419439674,
-1.41715560886723));
#74057=CARTESIAN_POINT('Ctrl Pts',(0.0323409617841025,-0.292888089443892,
-1.41625922610103));
#74058=CARTESIAN_POINT('Ctrl Pts',(0.0487168620251309,-0.290138427917476,
-1.41536284333484));
#74059=CARTESIAN_POINT('Ctrl Pts',(0.0650899257250815,-0.287389242671921,
-1.41446661583501));
#74060=CARTESIAN_POINT('Ctrl Pts',(0.0812459793976757,-0.28324705834533,
-1.41357038833518));
#74061=CARTESIAN_POINT('Ctrl Pts',(0.096936217163283,-0.277771506461827,
-1.41267416083535));
#74062=CARTESIAN_POINT('Ctrl Pts',(0.112622243843119,-0.272297424155712,
-1.41177817387303));
#74063=CARTESIAN_POINT('Ctrl Pts',(0.127841958827308,-0.265490955779006,
-1.41088218691072));
#74064=CARTESIAN_POINT('Ctrl Pts',(0.142364081094165,-0.257460887154173,
-1.40998619994841));
#74065=CARTESIAN_POINT('Ctrl Pts',(0.156921088716833,-0.249411528525028,
-1.40908806062687));
#74066=CARTESIAN_POINT('Ctrl Pts',(0.170776473709852,-0.240133106685944,
-1.40818992130532));
#74067=CARTESIAN_POINT('Ctrl Pts',(0.183725423100417,-0.229779478863045,
-1.40729178198377));
#74068=CARTESIAN_POINT('Ctrl Pts',(0.195400423362444,-0.220444466121908,
-1.40648200379265));
#74069=CARTESIAN_POINT('Ctrl Pts',(0.206338661513041,-0.210236277728869,
-1.40567222560153));
#74070=CARTESIAN_POINT('Ctrl Pts',(0.216415787233943,-0.199293369272318,
-1.40486244741041));
#74071=CARTESIAN_POINT('Ctrl Pts',(0.227592372484364,-0.187156540513847,
-1.40396431879342));
#74072=CARTESIAN_POINT('Ctrl Pts',(0.23778054528921,-0.174037784004933,
-1.40306619017643));
#74073=CARTESIAN_POINT('Ctrl Pts',(0.246807810200392,-0.160123529888917,
-1.40216806155943));
#74074=CARTESIAN_POINT('Ctrl Pts',(0.255817527226674,-0.146236323359531,
-1.40127167879323));
#74075=CARTESIAN_POINT('Ctrl Pts',(0.263670334362132,-0.131557308898357,
-1.40037529602703));
#74076=CARTESIAN_POINT('Ctrl Pts',(0.270234772888155,-0.116304804380935,
-1.39947891326083));
#74077=CARTESIAN_POINT('Ctrl Pts',(0.276798074359162,-0.101054941816316,
-1.398582685761));
#74078=CARTESIAN_POINT('Ctrl Pts',(0.282073089550326,-0.0852324901730909,
-1.39768645826116));
#74079=CARTESIAN_POINT('Ctrl Pts',(0.285975087319612,-0.0690788638625486,
-1.39679023076133));
#74080=CARTESIAN_POINT('Ctrl Pts',(0.289876037835979,-0.0529295730061226,
-1.39589424379901));
#74081=CARTESIAN_POINT('Ctrl Pts',(0.292404527066775,-0.0364500560782893,
-1.3949982568367));
#74082=CARTESIAN_POINT('Ctrl Pts',(0.29352663098193,-0.019893639797628,
-1.39410226987438));
#74083=CARTESIAN_POINT('Ctrl Pts',(0.294651430439349,-0.00329745133613088,
-1.39320413055283));
#74084=CARTESIAN_POINT('Ctrl Pts',(0.294363069428234,0.0133752105106759,
-1.39230599123128));
#74085=CARTESIAN_POINT('Ctrl Pts',(0.292679846716762,0.0298688353615089,
-1.39140785190973));
#74086=CARTESIAN_POINT('Ctrl Pts',(0.291162223548715,0.0447397772921781,
-1.39059807371863));
#74087=CARTESIAN_POINT('Ctrl Pts',(0.288511482478781,0.0594647810571047,
-1.38978829552753));
#74088=CARTESIAN_POINT('Ctrl Pts',(0.284776587124312,0.0738643041382596,
-1.38897851733643));
#74089=CARTESIAN_POINT('Ctrl Pts',(0.280634197966181,0.089834879651773,
-1.38808038871944));
#74090=CARTESIAN_POINT('Ctrl Pts',(0.275130908931858,0.105506971000544,
-1.38718226010245));
#74091=CARTESIAN_POINT('Ctrl Pts',(0.268329908128366,0.120634573832806,
-1.38628413148546));
#74092=CARTESIAN_POINT('Ctrl Pts',(0.261542127628087,0.135732770478817,
-1.38538774871926));
#74093=CARTESIAN_POINT('Ctrl Pts',(0.253461902951509,0.150287838827411,
-1.38449136595306));
#74094=CARTESIAN_POINT('Ctrl Pts',(0.244201461264651,0.164070979506459,
-1.38359498318686));
#74095=CARTESIAN_POINT('Ctrl Pts',(0.234942623619273,0.177851732747617,
-1.38269875568703));
#74096=CARTESIAN_POINT('Ctrl Pts',(0.2245043707634,0.190860139205912,-1.3818025281872));
#74097=CARTESIAN_POINT('Ctrl Pts',(0.213043665088906,0.202894151629578,
-1.38090630068737));
#74098=CARTESIAN_POINT('Ctrl Pts',(0.201586035340687,0.214924934257797,
-1.38001031372506));
#74099=CARTESIAN_POINT('Ctrl Pts',(0.189107051380983,0.225981276116504,
-1.37911432676275));
#74100=CARTESIAN_POINT('Ctrl Pts',(0.175801222612858,0.235897372023989,
-1.37821833980044));
#74101=CARTESIAN_POINT('Ctrl Pts',(0.162463430295437,0.245837288591269,
-1.37732020047889));
#74102=CARTESIAN_POINT('Ctrl Pts',(0.148295479221592,0.254631034522214,
-1.37642206115735));
#74103=CARTESIAN_POINT('Ctrl Pts',(0.133522017133855,0.26215550907907,-1.3755239218358));
#74104=CARTESIAN_POINT('Ctrl Pts',(0.120202004170434,0.268939707532015,
-1.37471414364468));
#74105=CARTESIAN_POINT('Ctrl Pts',(0.106390521317145,0.274692542094154,
-1.37390436545356));
#74106=CARTESIAN_POINT('Ctrl Pts',(0.0922649925235385,0.27935785500793,
-1.37309458726244));
#74107=CARTESIAN_POINT('Ctrl Pts',(0.0765983053012701,0.284532174446308,
-1.37219645864545));
#74108=CARTESIAN_POINT('Ctrl Pts',(0.0604448964933684,0.288401027160595,
-1.37129833002846));
#74109=CARTESIAN_POINT('Ctrl Pts',(0.0440457536748395,0.290884189297417,
-1.37040020141147));
#74110=CARTESIAN_POINT('Ctrl Pts',(0.0276784887588075,0.293362524474601,
-1.36950381864527));
#74111=CARTESIAN_POINT('Ctrl Pts',(0.011067201584773,0.294460333145734,
-1.36860743587907));
#74112=CARTESIAN_POINT('Ctrl Pts',(-0.005535001596226,0.294147928358045,
-1.36771105311288));
#74113=CARTESIAN_POINT('Ctrl Pts',(-0.0221343290372297,0.293835577683352,
-1.36681482561304));
#74114=CARTESIAN_POINT('Ctrl Pts',(-0.038723785711801,0.29211346023372,
-1.36591859811321));
#74115=CARTESIAN_POINT('Ctrl Pts',(-0.0550485026375527,0.289003983289787,
-1.36502237061338));
#74116=CARTESIAN_POINT('Ctrl Pts',(-0.0713688381903642,0.285895340894973,
-1.36412638365107));
#74117=CARTESIAN_POINT('Ctrl Pts',(-0.0874237993062656,0.28140023694395,
-1.36323039668875));
#74118=CARTESIAN_POINT('Ctrl Pts',(-0.102968625401473,0.275592275259905,
-1.36233440972644));
#74119=CARTESIAN_POINT('Ctrl Pts',(-0.118550793613721,0.26977036156484,
-1.36143627040489));
#74120=CARTESIAN_POINT('Ctrl Pts',(-0.133619643773714,0.262629594100133,
-1.36053813108334));
#74121=CARTESIAN_POINT('Ctrl Pts',(-0.147949969939373,0.254292049413541,
-1.3596399917618));
#74122=CARTESIAN_POINT('Ctrl Pts',(-0.16087044377021,0.246774772647384,
-1.35883021357068));
#74123=CARTESIAN_POINT('Ctrl Pts',(-0.173190523650776,0.238285497304914,
-1.35802043537957));
#74124=CARTESIAN_POINT('Ctrl Pts',(-0.184766856253945,0.228942894255388,
-1.35721065718845));
#74125=CARTESIAN_POINT('Ctrl Pts',(-0.197440381985434,0.218714808711713,
-1.35632412903712));
#74126=CARTESIAN_POINT('Ctrl Pts',(-0.2093075580526,0.207394171215443,-1.35543760088579));
#74127=CARTESIAN_POINT('Ctrl Pts',(-0.220172996192097,0.195134547806878,
-1.35455107273446));
#74128=CARTESIAN_POINT('Ctrl Pts',(-0.231017282860132,0.1828987898947,-1.35366627036488));
#74129=CARTESIAN_POINT('Ctrl Pts',(-0.240863114080798,0.169728227077772,
-1.3527814679953));
#74130=CARTESIAN_POINT('Ctrl Pts',(-0.249550676841476,0.155814311563351,
-1.35189666562572));
#74131=CARTESIAN_POINT('Ctrl Pts',(-0.258235555527538,0.141904694836574,
-1.35101213662115));
#74132=CARTESIAN_POINT('Ctrl Pts',(-0.265762406856247,0.127252844514462,
-1.35012760761657));
#74133=CARTESIAN_POINT('Ctrl Pts',(-0.27201421930744,0.112079902277633,
-1.34924307861199));
#74134=CARTESIAN_POINT('Ctrl Pts',(-0.278265017748795,0.0969094210091772,
-1.34835869307318));
#74135=CARTESIAN_POINT('Ctrl Pts',(-0.283240895905996,0.0812187746302049,
-1.34747430753438));
#74136=CARTESIAN_POINT('Ctrl Pts',(-0.286873342468991,0.0652481829683322,
-1.34658992199557));
#74137=CARTESIAN_POINT('Ctrl Pts',(-0.29051252747974,0.0492479647185263,
-1.34570389585845));
#74138=CARTESIAN_POINT('Ctrl Pts',(-0.292803179103319,0.0329675687853759,
-1.34481786972132));
#74139=CARTESIAN_POINT('Ctrl Pts',(-0.293728134706627,0.0166560163834503,
-1.34393184358419));
#74140=CARTESIAN_POINT('Ctrl Pts',(-0.294046268245785,0.0110457450620725,
-1.34362709962698));
#74141=CARTESIAN_POINT('Ctrl Pts',(-0.294203297540194,0.0054317968864524,
-1.34332235566977));
#74142=CARTESIAN_POINT('Ctrl Pts',(-0.294199947499254,-0.000175759597174776,
-1.34301761171257));
#74143=CARTESIAN_POINT('',(-0.29419988923003,0.000255297940232041,-1.24301761170896));
#74144=CARTESIAN_POINT('Ctrl Pts',(-0.294199947499215,-0.00017575966358228,
-1.34301761170896));
#74145=CARTESIAN_POINT('Ctrl Pts',(-0.294193751549442,-0.010547013571074,
-1.3424539835108));
#74146=CARTESIAN_POINT('Ctrl Pts',(-0.293639176427434,-0.0209017185291566,
-1.34189035531263));
#74147=CARTESIAN_POINT('Ctrl Pts',(-0.292541208478424,-0.0311974572999702,
-1.34132672711446));
#74148=CARTESIAN_POINT('Ctrl Pts',(-0.290791621714033,-0.0476034810816983,
-1.34042859849746));
#74149=CARTESIAN_POINT('Ctrl Pts',(-0.287652041311442,-0.0639143263184607,
-1.33953046988046));
#74150=CARTESIAN_POINT('Ctrl Pts',(-0.28314880433921,-0.0798773722732269,
-1.33863234126347));
#74151=CARTESIAN_POINT('Ctrl Pts',(-0.278654321101896,-0.0958093880437881,
-1.33773595849726));
#74152=CARTESIAN_POINT('Ctrl Pts',(-0.2728015916199,-0.111394175596688,
-1.33683957573106));
#74153=CARTESIAN_POINT('Ctrl Pts',(-0.265667988492458,-0.126388923131623,
-1.33594319296486));
#74154=CARTESIAN_POINT('Ctrl Pts',(-0.258535621007514,-0.141381073360964,
-1.33504696546503));
#74155=CARTESIAN_POINT('Ctrl Pts',(-0.250123111352777,-0.155782651141836,
-1.33415073796519));
#74156=CARTESIAN_POINT('Ctrl Pts',(-0.240556014087382,-0.169370729721494,
-1.33325451046536));
#74157=CARTESIAN_POINT('Ctrl Pts',(-0.230991484524771,-0.182955161411586,
-1.33235852350305));
#74158=CARTESIAN_POINT('Ctrl Pts',(-0.220273447152277,-0.195725886169684,
-1.33146253654073));
#74159=CARTESIAN_POINT('Ctrl Pts',(-0.208569923466897,-0.207490305857919,
-1.33056654957842));
#74160=CARTESIAN_POINT('Ctrl Pts',(-0.196838285324102,-0.219282986289262,
-1.32966841025687));
#74161=CARTESIAN_POINT('Ctrl Pts',(-0.18411701195124,-0.230063988510944,
-1.32877027093533));
#74162=CARTESIAN_POINT('Ctrl Pts',(-0.170610213622442,-0.239678524293907,
-1.32787213161378));
#74163=CARTESIAN_POINT('Ctrl Pts',(-0.158432246957576,-0.248347158666972,
-1.32706235342268));
#74164=CARTESIAN_POINT('Ctrl Pts',(-0.145616531664977,-0.256067884386416,
-1.32625257523158));
#74165=CARTESIAN_POINT('Ctrl Pts',(-0.132330308425864,-0.262759071150581,
-1.32544279704048));
#74166=CARTESIAN_POINT('Ctrl Pts',(-0.117594498751165,-0.270180296346038,
-1.32454466842349));
#74167=CARTESIAN_POINT('Ctrl Pts',(-0.102185341950397,-0.2763817900475,
-1.3236465398065));
#74168=CARTESIAN_POINT('Ctrl Pts',(-0.0863294138337773,-0.281248772987753,
-1.32274841118951));
#74169=CARTESIAN_POINT('Ctrl Pts',(-0.0705043076775544,-0.286106295115977,
-1.32185202842331));
#74170=CARTESIAN_POINT('Ctrl Pts',(-0.0542348825185319,-0.28963416280787,
-1.32095564565711));
#74171=CARTESIAN_POINT('Ctrl Pts',(-0.0377671304889351,-0.29176580309322,
-1.32005926289092));
#74172=CARTESIAN_POINT('Ctrl Pts',(-0.0213022309104615,-0.293897074147864,
-1.31916303539108));
#74173=CARTESIAN_POINT('Ctrl Pts',(-0.00463984835274561,-0.294632443965077,
-1.31826680789125));
#74174=CARTESIAN_POINT('Ctrl Pts',(0.0119646232211581,-0.293956608687704,
-1.31737058039142));
#74175=CARTESIAN_POINT('Ctrl Pts',(0.0285646383390764,-0.293280954797022,
-1.3164745934291));
#74176=CARTESIAN_POINT('Ctrl Pts',(0.0451059826769823,-0.291194890690062,
-1.31557860646679));
#74177=CARTESIAN_POINT('Ctrl Pts',(0.0613357345627556,-0.287735238831894,
-1.31468261950448));
#74178=CARTESIAN_POINT('Ctrl Pts',(0.077604473909099,-0.284267276123298,
-1.31378448018293));
#74179=CARTESIAN_POINT('Ctrl Pts',(0.0935593538175207,-0.27941932684169,
-1.31288634086138));
#74180=CARTESIAN_POINT('Ctrl Pts',(0.108959668941943,-0.273279034219719,
-1.31198820153983));
#74181=CARTESIAN_POINT('Ctrl Pts',(0.122844863615938,-0.267742838517063,
-1.31117842334871));
#74182=CARTESIAN_POINT('Ctrl Pts',(0.136279078635207,-0.261156942152836,
-1.3103686451576));
#74183=CARTESIAN_POINT('Ctrl Pts',(0.149103072629811,-0.253617652643402,
-1.30955886696648));
#74184=CARTESIAN_POINT('Ctrl Pts',(0.163326221779837,-0.245255792896507,
-1.30866073834949));
#74185=CARTESIAN_POINT('Ctrl Pts',(0.176889245284057,-0.235666995742333,
-1.3077626097325));
#74186=CARTESIAN_POINT('Ctrl Pts',(0.189572885590776,-0.224979468060502,
-1.30686448111551));
#74187=CARTESIAN_POINT('Ctrl Pts',(0.202231870471692,-0.214312715608763,
-1.30596809834931));
#74188=CARTESIAN_POINT('Ctrl Pts',(0.214014224319459,-0.202551925530603,
-1.30507171558311));
#74189=CARTESIAN_POINT('Ctrl Pts',(0.224730678981851,-0.189867748510262,
-1.30417533281691));
#74190=CARTESIAN_POINT('Ctrl Pts',(0.23544527740041,-0.177185768571524,
-1.30327910531708));
#74191=CARTESIAN_POINT('Ctrl Pts',(0.245093793381539,-0.163581287668909,
-1.30238287781725));
#74192=CARTESIAN_POINT('Ctrl Pts',(0.253524949710887,-0.149260644089768,
-1.30148665031742));
#74193=CARTESIAN_POINT('Ctrl Pts',(0.261953843211399,-0.134943844012512,
-1.30059066335511));
#74194=CARTESIAN_POINT('Ctrl Pts',(0.269165633287289,-0.119911950590032,
-1.29969467639279));
#74195=CARTESIAN_POINT('Ctrl Pts',(0.275054189477498,-0.104397475308919,
-1.29879868943048));
#74196=CARTESIAN_POINT('Ctrl Pts',(0.280956891284591,-0.0888457308201479,
-1.29790055010894));
#74197=CARTESIAN_POINT('Ctrl Pts',(0.28552975301188,-0.0728098416726041,
-1.29700241078739));
#74198=CARTESIAN_POINT('Ctrl Pts',(0.288715974741864,-0.0565395961150734,
-1.29610427146584));
#74199=CARTESIAN_POINT('Ctrl Pts',(0.291588728230211,-0.0418700568793609,
-1.29529449327473));
#74200=CARTESIAN_POINT('Ctrl Pts',(0.29333489813115,-0.027010613592972,
-1.29448471508361));
#74201=CARTESIAN_POINT('Ctrl Pts',(0.293949117009706,-0.0121472881423871,
-1.2936749368925));
#74202=CARTESIAN_POINT('Ctrl Pts',(0.294630349917656,0.00433769265518017,
-1.29277680827551));
#74203=CARTESIAN_POINT('Ctrl Pts',(0.293922699000598,0.0209328686897962,
-1.29187867965852));
#74204=CARTESIAN_POINT('Ctrl Pts',(0.291815078002818,0.0373844921084808,
-1.29098055104153));
#74205=CARTESIAN_POINT('Ctrl Pts',(0.289711553959215,0.0538041356088827,
-1.29008416827533));
#74206=CARTESIAN_POINT('Ctrl Pts',(0.286213495329414,0.0700799959941093,
-1.28918778550913));
#74207=CARTESIAN_POINT('Ctrl Pts',(0.281361738894204,0.085960525163762,
-1.28829140274293));
#74208=CARTESIAN_POINT('Ctrl Pts',(0.276510822852879,0.101838303597721,
-1.2873951752431));
#74209=CARTESIAN_POINT('Ctrl Pts',(0.270306854263215,0.117320116637753,
-1.28649894774327));
#74210=CARTESIAN_POINT('Ctrl Pts',(0.262841251640155,0.132167002070247,
-1.28560272024343));
#74211=CARTESIAN_POINT('Ctrl Pts',(0.255377652702027,0.14700990276338,-1.28470673328112));
#74212=CARTESIAN_POINT('Ctrl Pts',(0.246653457261611,0.161217511636139,
-1.28381074631881));
#74213=CARTESIAN_POINT('Ctrl Pts',(0.236806547921958,0.174574622615332,
-1.2829147593565));
#74214=CARTESIAN_POINT('Ctrl Pts',(0.226935984123979,0.187963820335056,
-1.28201662003495));
#74215=CARTESIAN_POINT('Ctrl Pts',(0.21593781269343,0.200497815321246,-1.2811184807134));
#74216=CARTESIAN_POINT('Ctrl Pts',(0.203991171264655,0.211993495291894,
-1.28022034139185));
#74217=CARTESIAN_POINT('Ctrl Pts',(0.19321986946998,0.222358202313284,-1.27941056320074));
#74218=CARTESIAN_POINT('Ctrl Pts',(0.18167839813468,0.231879053300413,-1.27860078500963));
#74219=CARTESIAN_POINT('Ctrl Pts',(0.169520180650363,0.240450719176026,
-1.27779100681851));
#74220=CARTESIAN_POINT('Ctrl Pts',(0.1560354472084,0.249957592172443,-1.27689287820152));
#74221=CARTESIAN_POINT('Ctrl Pts',(0.141705372455059,0.258356972804593,
-1.27599474958453));
#74222=CARTESIAN_POINT('Ctrl Pts',(0.126737197104228,0.265502020463431,
-1.27509662096754));
#74223=CARTESIAN_POINT('Ctrl Pts',(0.111798118032371,0.272633179034582,
-1.27420023820134));
#74224=CARTESIAN_POINT('Ctrl Pts',(0.0962240779494825,0.278514447686267,
-1.27330385543514));
#74225=CARTESIAN_POINT('Ctrl Pts',(0.0802486096345411,0.283043814014232,
-1.27240747266894));
#74226=CARTESIAN_POINT('Ctrl Pts',(0.0642759085001157,0.287572395790908,
-1.27151124516911));
#74227=CARTESIAN_POINT('Ctrl Pts',(0.0479026618057446,0.290749273810779,
-1.27061501766928));
#74228=CARTESIAN_POINT('Ctrl Pts',(0.031379238965604,0.29252176562085,-1.26971879016945));
#74229=CARTESIAN_POINT('Ctrl Pts',(0.0148602508288663,0.294293781713781,
-1.26882280320714));
#74230=CARTESIAN_POINT('Ctrl Pts',(-0.00180804505916306,0.294662086143294,
-1.26792681624482));
#74231=CARTESIAN_POINT('Ctrl Pts',(-0.0183700617464465,0.293625919890312,
-1.26703082928251));
#74232=CARTESIAN_POINT('Ctrl Pts',(-0.0349718640679828,0.292587264536374,
-1.26613268996096));
#74233=CARTESIAN_POINT('Ctrl Pts',(-0.0514660855087487,0.290137475934808,
-1.26523455063941));
#74234=CARTESIAN_POINT('Ctrl Pts',(-0.0676017516749918,0.286327859577919,
-1.26433641131787));
#74235=CARTESIAN_POINT('Ctrl Pts',(-0.0821499517671537,0.282893042541959,
-1.26352663312675));
#74236=CARTESIAN_POINT('Ctrl Pts',(-0.0964063859679396,0.278353632009501,
-1.26271685493564));
#74237=CARTESIAN_POINT('Ctrl Pts',(-0.110199385066545,0.272781479450045,
-1.26190707674452));
#74238=CARTESIAN_POINT('Ctrl Pts',(-0.125497262115504,0.26660138010086,
-1.26100894812753));
#74239=CARTESIAN_POINT('Ctrl Pts',(-0.140322554736792,0.25911063006276,
-1.26011081951054));
#74240=CARTESIAN_POINT('Ctrl Pts',(-0.154439540141873,0.250403810755282,
-1.25921269089355));
#74241=CARTESIAN_POINT('Ctrl Pts',(-0.168529083875808,0.24171391642614,
-1.25831630812735));
#74242=CARTESIAN_POINT('Ctrl Pts',(-0.181912352764208,0.231812999331368,
-1.25741992536115));
#74243=CARTESIAN_POINT('Ctrl Pts',(-0.194377048029768,0.22084203222945,
-1.25652354259495));
#74244=CARTESIAN_POINT('Ctrl Pts',(-0.206839584231116,0.209872965456575,
-1.25562731509512));
#74245=CARTESIAN_POINT('Ctrl Pts',(-0.218383235302948,0.197834698089562,
-1.25473108759529));
#74246=CARTESIAN_POINT('Ctrl Pts',(-0.22882803429704,0.18490908771543,-1.25383486009546));
#74247=CARTESIAN_POINT('Ctrl Pts',(-0.239270030022942,0.171986946431744,
-1.25293887313314));
#74248=CARTESIAN_POINT('Ctrl Pts',(-0.248613269914563,0.158178557521689,
-1.25204288617083));
#74249=CARTESIAN_POINT('Ctrl Pts',(-0.256718595612957,0.143698304327195,
-1.25114689920852));
#74250=CARTESIAN_POINT('Ctrl Pts',(-0.264843392099831,0.12918326635568,
-1.25024875988697));
#74251=CARTESIAN_POINT('Ctrl Pts',(-0.271723969716891,0.11399384711777,
-1.24935062056542));
#74252=CARTESIAN_POINT('Ctrl Pts',(-0.277267424873653,0.0983687709790725,
-1.24845248124387));
#74253=CARTESIAN_POINT('Ctrl Pts',(-0.282265501432228,0.0842809278259624,
-1.24764270305276));
#74254=CARTESIAN_POINT('Ctrl Pts',(-0.286177151682841,0.0698396274544479,
-1.24683292486165));
#74255=CARTESIAN_POINT('Ctrl Pts',(-0.288969719865065,0.055228081635216,
-1.24602314667053));
#74256=CARTESIAN_POINT('Ctrl Pts',(-0.2924246417998,0.0371509043356214,
-1.24502130168334));
#74257=CARTESIAN_POINT('Ctrl Pts',(-0.294183848952715,0.0187397706500721,
-1.24401945669615));
#74258=CARTESIAN_POINT('Ctrl Pts',(-0.29419988923003,0.000255297940232041,
-1.24301761170896));
#74259=CARTESIAN_POINT('',(-0.294152882452219,2.44525333549389E-5,-1.14301761352535));
#74260=CARTESIAN_POINT('Ctrl Pts',(-0.294329728545196,0.000254154008116347,
-1.2430175436321));
#74261=CARTESIAN_POINT('Ctrl Pts',(-0.293605515756253,-0.0789850627824231,
-1.23872476795359));
#74262=CARTESIAN_POINT('Ctrl Pts',(-0.219727723116684,-0.257146121866797,
-1.22913734891706));
#74263=CARTESIAN_POINT('Ctrl Pts',(0.081449915577503,-0.338109609170002,
-1.21425528652256));
#74264=CARTESIAN_POINT('Ctrl Pts',(0.328289982877296,-0.114794963753201,
-1.19837135644858));
#74265=CARTESIAN_POINT('Ctrl Pts',(0.274396781387414,0.213678737652817,
-1.18248742637458));
#74266=CARTESIAN_POINT('Ctrl Pts',(-0.030860291423648,0.34640992909257,
-1.16660349630059));
#74267=CARTESIAN_POINT('Ctrl Pts',(-0.260287732143521,0.193505598037348,
-1.15344689759982));
#74268=CARTESIAN_POINT('Ctrl Pts',(-0.293753616556347,0.047664275140288,
-1.14558494225705));
#74269=CARTESIAN_POINT('Ctrl Pts',(-0.293718471850348,2.47272304220616E-5,
-1.14301763027227));
#74270=CARTESIAN_POINT('',(-0.294199878709568,-0.000267146542919366,-1.04301761170896));
#74271=CARTESIAN_POINT('Ctrl Pts',(-0.294199998986285,2.44227394832766E-5,
-1.14301761170896));
#74272=CARTESIAN_POINT('Ctrl Pts',(-0.294201439091654,-0.0173233034906427,
-1.1420842667241));
#74273=CARTESIAN_POINT('Ctrl Pts',(-0.292664192110059,-0.0346450682093256,
-1.14115092173924));
#74274=CARTESIAN_POINT('Ctrl Pts',(-0.289627608697573,-0.0516670908811927,
-1.14021757675438));
#74275=CARTESIAN_POINT('Ctrl Pts',(-0.286578246409207,-0.068760747453864,
-1.13928030396709));
#74276=CARTESIAN_POINT('Ctrl Pts',(-0.282017105962231,-0.0855514630817754,
-1.13834303117979));
#74277=CARTESIAN_POINT('Ctrl Pts',(-0.276034546441971,-0.101777056209027,
-1.1374057583925));
#74278=CARTESIAN_POINT('Ctrl Pts',(-0.27056623117564,-0.116607942270845,
-1.13654905097921));
#74279=CARTESIAN_POINT('Ctrl Pts',(-0.263911154304513,-0.130966526867975,
-1.13569234356592));
#74280=CARTESIAN_POINT('Ctrl Pts',(-0.256172065381413,-0.14467035950125,
-1.13483563615262));
#74281=CARTESIAN_POINT('Ctrl Pts',(-0.248058796926603,-0.159036762849026,
-1.13393750753563));
#74282=CARTESIAN_POINT('Ctrl Pts',(-0.238707297624362,-0.172764475631579,
-1.13303937891864));
#74283=CARTESIAN_POINT('Ctrl Pts',(-0.228241942290027,-0.185632044054026,
-1.13214125030165));
#74284=CARTESIAN_POINT('Ctrl Pts',(-0.217796930310254,-0.1984745995172,
-1.13124486753545));
#74285=CARTESIAN_POINT('Ctrl Pts',(-0.206242802347557,-0.210459680763422,
-1.13034848476925));
#74286=CARTESIAN_POINT('Ctrl Pts',(-0.193746892091351,-0.221395080805654,
-1.12945210200305));
#74287=CARTESIAN_POINT('Ctrl Pts',(-0.181253146306246,-0.232328586679565,
-1.12855587450322));
#74288=CARTESIAN_POINT('Ctrl Pts',(-0.167818500885398,-0.242212212718823,
-1.12765964700339));
#74289=CARTESIAN_POINT('Ctrl Pts',(-0.153646632351437,-0.250891116556689,
-1.12676341950355));
#74290=CARTESIAN_POINT('Ctrl Pts',(-0.13947856738979,-0.259567691073036,
-1.12586743254124));
#74291=CARTESIAN_POINT('Ctrl Pts',(-0.124574352940194,-0.267039780981758,
-1.12497144557893));
#74292=CARTESIAN_POINT('Ctrl Pts',(-0.109164619826008,-0.273197228716258,
-1.12407545861661));
#74293=CARTESIAN_POINT('Ctrl Pts',(-0.0937178691180572,-0.279369468004716,
-1.12317731929506));
#74294=CARTESIAN_POINT('Ctrl Pts',(-0.077763922306269,-0.284220487099293,
-1.12227917997351));
#74295=CARTESIAN_POINT('Ctrl Pts',(-0.0615515421749449,-0.28768915109174,
-1.12138104065197));
#74296=CARTESIAN_POINT('Ctrl Pts',(-0.046934175424128,-0.290816559485957,
-1.12057126246085));
#74297=CARTESIAN_POINT('Ctrl Pts',(-0.032107343124302,-0.292820856883143,
-1.11976148426974));
#74298=CARTESIAN_POINT('Ctrl Pts',(-0.0172569457007118,-0.293693441917048,
-1.11895170607862));
#74299=CARTESIAN_POINT('Ctrl Pts',(-0.000786303435730034,-0.294661229884554,
-1.11805357746163));
#74300=CARTESIAN_POINT('Ctrl Pts',(0.015818668767146,-0.294242260217352,
-1.11715544884464));
#74301=CARTESIAN_POINT('Ctrl Pts',(0.0323044542012235,-0.292421035903303,
-1.11625732022765));
#74302=CARTESIAN_POINT('Ctrl Pts',(0.0487581933102811,-0.290603351823752,
-1.11536093746145));
#74303=CARTESIAN_POINT('Ctrl Pts',(0.0650924206680926,-0.287388843761867,
-1.11446455469525));
#74304=CARTESIAN_POINT('Ctrl Pts',(0.0810549160959561,-0.282813968142801,
-1.11356817192905));
#74305=CARTESIAN_POINT('Ctrl Pts',(0.0970146465904034,-0.278239884957885,
-1.11267194442922));
#74306=CARTESIAN_POINT('Ctrl Pts',(0.112601999852034,-0.272306068347537,
-1.11177571692939));
#74307=CARTESIAN_POINT('Ctrl Pts',(0.127576460117915,-0.265099767679608,
-1.11087948942956));
#74308=CARTESIAN_POINT('Ctrl Pts',(0.142546901404766,-0.257895401102841,
-1.10998350246725));
#74309=CARTESIAN_POINT('Ctrl Pts',(0.156904067496427,-0.249419581509413,
-1.10908751550494));
#74310=CARTESIAN_POINT('Ctrl Pts',(0.170430387212349,-0.239806428426448,
-1.10819152854263));
#74311=CARTESIAN_POINT('Ctrl Pts',(0.183989200145682,-0.230170182419487,
-1.10729338922108));
#74312=CARTESIAN_POINT('Ctrl Pts',(0.19671254767203,-0.219391628116924,
-1.10639524989953));
#74313=CARTESIAN_POINT('Ctrl Pts',(0.208414230163847,-0.207646691919739,
-1.10549711057798));
#74314=CARTESIAN_POINT('Ctrl Pts',(0.218964672677452,-0.197057251105479,
-1.10468733238687));
#74315=CARTESIAN_POINT('Ctrl Pts',(0.228684779260871,-0.18568308335087,
-1.10387755419576));
#74316=CARTESIAN_POINT('Ctrl Pts',(0.237466568876532,-0.173675757277771,
-1.10306777600465));
#74317=CARTESIAN_POINT('Ctrl Pts',(0.247206491053715,-0.160358378175512,
-1.10216964738766));
#74318=CARTESIAN_POINT('Ctrl Pts',(0.255853787998005,-0.146176527344347,
-1.10127151877066));
#74319=CARTESIAN_POINT('Ctrl Pts',(0.263258037584813,-0.131334860745323,
-1.10037339015367));
#74320=CARTESIAN_POINT('Ctrl Pts',(0.27064789422749,-0.116522044507928,
-1.09947700738747));
#74321=CARTESIAN_POINT('Ctrl Pts',(0.276799091300331,-0.101052628874886,
-1.09858062462128));
#74322=CARTESIAN_POINT('Ctrl Pts',(0.281605570911589,-0.0851583374165925,
-1.09768424185508));
#74323=CARTESIAN_POINT('Ctrl Pts',(0.286411217971558,-0.0692667990778169,
-1.09678801435524));
#74324=CARTESIAN_POINT('Ctrl Pts',(0.289872330758011,-0.0529512709053253,
-1.09589178685541));
#74325=CARTESIAN_POINT('Ctrl Pts',(0.291931881098733,-0.0364611683597093,
-1.09499555935558));
#74326=CARTESIAN_POINT('Ctrl Pts',(0.29399087867899,-0.0199754915746974,
-1.09409957239327));
#74327=CARTESIAN_POINT('Ctrl Pts',(0.294648973157355,-0.00331612040945406,
-1.09320358543095));
#74328=CARTESIAN_POINT('Ctrl Pts',(0.293900961216667,0.0132614100275669,
-1.09230759846864));
#74329=CARTESIAN_POINT('Ctrl Pts',(0.293151152385537,0.0298787633663042,
-1.09140945914709));
#74330=CARTESIAN_POINT('Ctrl Pts',(0.290988552942633,0.0464130903492512,
-1.09051131982554));
#74331=CARTESIAN_POINT('Ctrl Pts',(0.287460096417958,0.0626125623767172,
-1.08961318050399));
#74332=CARTESIAN_POINT('Ctrl Pts',(0.284278778026232,0.0772182909543078,
-1.08880340231288));
#74333=CARTESIAN_POINT('Ctrl Pts',(0.279987959623469,0.0915515055811006,
-1.08799362412177));
#74334=CARTESIAN_POINT('Ctrl Pts',(0.27465649665164,0.105439313574433,-1.08718384593065));
#74335=CARTESIAN_POINT('Ctrl Pts',(0.268743347201612,0.120842343592982,
-1.08628571731366));
#74336=CARTESIAN_POINT('Ctrl Pts',(0.261511527442603,0.135795651602018,
-1.08538758869667));
#74337=CARTESIAN_POINT('Ctrl Pts',(0.253051505499328,0.150061905773996,
-1.08448946007968));
#74338=CARTESIAN_POINT('Ctrl Pts',(0.244607928790882,0.164300428114831,
-1.08359307731348));
#74339=CARTESIAN_POINT('Ctrl Pts',(0.234941230979866,0.177853840928105,
-1.08269669454728));
#74340=CARTESIAN_POINT('Ctrl Pts',(0.224188671836702,0.190507426154718,
-1.08180031178108));
#74341=CARTESIAN_POINT('Ctrl Pts',(0.213437975191185,0.20315881959867,-1.08090408428125));
#74342=CARTESIAN_POINT('Ctrl Pts',(0.201602261081292,0.214910059225903,
-1.08000785678142));
#74343=CARTESIAN_POINT('Ctrl Pts',(0.188860230143771,0.225578042969704,
-1.07911162928159));
#74344=CARTESIAN_POINT('Ctrl Pts',(0.176121619026007,0.236243163545008,
-1.07821564231928));
#74345=CARTESIAN_POINT('Ctrl Pts',(0.162477787969324,0.24582510541816,-1.07731965535696));
#74346=CARTESIAN_POINT('Ctrl Pts',(0.148140668069825,0.254181003349632,
-1.07642366839465));
#74347=CARTESIAN_POINT('Ctrl Pts',(0.133769107231204,0.262556973999614,
-1.0755255290731));
#74348=CARTESIAN_POINT('Ctrl Pts',(0.11870163131608,0.269700640752514,-1.07462738975156));
#74349=CARTESIAN_POINT('Ctrl Pts',(0.103175313090077,0.275514962876365,
-1.07372925043001));
#74350=CARTESIAN_POINT('Ctrl Pts',(0.0891765118060444,0.280757257851153,
-1.07291947223889));
#74351=CARTESIAN_POINT('Ctrl Pts',(0.0748054148313669,0.284919437069828,
-1.07210969404778));
#74352=CARTESIAN_POINT('Ctrl Pts',(0.0602446383824871,0.287965663831929,
-1.07129991585666));
#74353=CARTESIAN_POINT('Ctrl Pts',(0.044095216037158,0.291344247571163,
-1.07040178723967));
#74354=CARTESIAN_POINT('Ctrl Pts',(0.0276090592174151,0.293370887834,-1.06950365862268));
#74355=CARTESIAN_POINT('Ctrl Pts',(0.0110346520815367,0.293992987082072,
-1.06860553000569));
#74356=CARTESIAN_POINT('Ctrl Pts',(-0.00550753645972035,0.294613877046257,
-1.06770914723949));
#74357=CARTESIAN_POINT('Ctrl Pts',(-0.0221368555162454,0.293835549883038,
-1.06681276447329));
#74358=CARTESIAN_POINT('Ctrl Pts',(-0.0385984658186121,0.291656987635218,
-1.06591638170709));
#74359=CARTESIAN_POINT('Ctrl Pts',(-0.0550572247336882,0.289478802745662,
-1.06502015420726));
#74360=CARTESIAN_POINT('Ctrl Pts',(-0.0713475433805044,0.285900915149179,
-1.06412392670743));
#74361=CARTESIAN_POINT('Ctrl Pts',(-0.0872186927898397,0.280974268622647,
-1.0632276992076));
#74362=CARTESIAN_POINT('Ctrl Pts',(-0.103085582558728,0.276048944353394,
-1.06233171224529));
#74363=CARTESIAN_POINT('Ctrl Pts',(-0.118532773472252,0.269775824806875,
-1.06143572528297));
#74364=CARTESIAN_POINT('Ctrl Pts',(-0.13332534158677,0.262255587720779,
-1.06053973832066));
#74365=CARTESIAN_POINT('Ctrl Pts',(-0.148153444727958,0.254717285358705,
-1.05964159899911));
#74366=CARTESIAN_POINT('Ctrl Pts',(-0.162323087557588,0.245926265667551,
-1.05874345967756));
#74367=CARTESIAN_POINT('Ctrl Pts',(-0.175624230913873,0.236029170900358,
-1.05784532035602));
#74368=CARTESIAN_POINT('Ctrl Pts',(-0.187616775442742,0.227105776382856,
-1.0570355421649));
#74369=CARTESIAN_POINT('Ctrl Pts',(-0.19890336621151,0.217284114969341,
-1.05622576397379));
#74370=CARTESIAN_POINT('Ctrl Pts',(-0.209354913611055,0.206698234503606,
-1.05541598578268));
#74371=CARTESIAN_POINT('Ctrl Pts',(-0.220789690983753,0.195116486673142,
-1.05453002765775));
#74372=CARTESIAN_POINT('Ctrl Pts',(-0.231301783831298,0.182540831427682,
-1.05364406953283));
#74373=CARTESIAN_POINT('Ctrl Pts',(-0.240714390826723,0.169145564674099,
-1.05275811140791));
#74374=CARTESIAN_POINT('Ctrl Pts',(-0.250111460747171,0.155772409038507,
-1.05187361570437));
#74375=CARTESIAN_POINT('Ctrl Pts',(-0.258412117491872,0.14158293958677,
-1.05098912000084));
#74376=CARTESIAN_POINT('Ctrl Pts',(-0.265479047062119,0.126785312915138,
-1.05010462429731));
#74377=CARTESIAN_POINT('Ctrl Pts',(-0.272538744393056,0.112002830016518,
-1.04922103377962));
#74378=CARTESIAN_POINT('Ctrl Pts',(-0.278366846345738,0.0966141464632306,
-1.04833744326193));
#74379=CARTESIAN_POINT('Ctrl Pts',(-0.282872149058977,0.0808516375020071,
-1.04745385274424));
#74380=CARTESIAN_POINT('Ctrl Pts',(-0.287382011663733,0.0650731750443189,
-1.04656936792995));
#74381=CARTESIAN_POINT('Ctrl Pts',(-0.290566177837302,0.0489209165269241,
-1.04568488311565));
#74382=CARTESIAN_POINT('Ctrl Pts',(-0.292383595975706,0.0326415809101696,
-1.04480039830136));
#74383=CARTESIAN_POINT('Ctrl Pts',(-0.293604671656364,0.0217039213816084,
-1.04420613610389));
#74384=CARTESIAN_POINT('Ctrl Pts',(-0.294209845691427,0.0107091693839332,
-1.04361187390643));
#74385=CARTESIAN_POINT('Ctrl Pts',(-0.294199878709568,-0.000267146542919366,
-1.04301761170896));
#74386=CARTESIAN_POINT('',(-0.294610924535095,0.000132059026951131,-0.943017611708961));
#74387=CARTESIAN_POINT('Ctrl Pts',(-0.294240133891941,-0.000267183096411164,
-1.04301761170896));
#74388=CARTESIAN_POINT('Ctrl Pts',(-0.294438591321936,-0.0217302969209736,
-1.04185575970887));
#74389=CARTESIAN_POINT('Ctrl Pts',(-0.282496855002347,-0.140783416643142,
-1.03539926435079));
#74390=CARTESIAN_POINT('Ctrl Pts',(-0.120486255734729,-0.32624417043023,
-1.0236481256347));
#74391=CARTESIAN_POINT('Ctrl Pts',(0.208874931436236,-0.278070961407654,
-1.00776419556071));
#74392=CARTESIAN_POINT('Ctrl Pts',(0.346894182589261,0.0248318876930918,
-0.991880265486725));
#74393=CARTESIAN_POINT('Ctrl Pts',(0.167137604763724,0.30498724175696,-0.975996335412736));
#74394=CARTESIAN_POINT('Ctrl Pts',(-0.165727020336765,0.305756032305122,
-0.96011240533875));
#74395=CARTESIAN_POINT('Ctrl Pts',(-0.291026760911973,0.112443587052818,
-0.94911949743749));
#74396=CARTESIAN_POINT('Ctrl Pts',(-0.294652539398193,0.00756385498649065,
-0.943421232894227));
#74397=CARTESIAN_POINT('Ctrl Pts',(-0.294610924535095,0.000132059026951131,
-0.943017611708961));
#74398=CARTESIAN_POINT('',(-0.294199939966062,0.0001879467097956,-0.843017611708961));
#74399=CARTESIAN_POINT('Ctrl Pts',(-0.294610924535095,0.000132059026951131,
-0.943017611708961));
#74400=CARTESIAN_POINT('Ctrl Pts',(-0.294106641743307,-0.0899253516050796,
-0.938126589536231));
#74401=CARTESIAN_POINT('Ctrl Pts',(-0.201793630053243,-0.278365916406644,
-0.927940924005507));
#74402=CARTESIAN_POINT('Ctrl Pts',(0.118977978713689,-0.326797241637504,
-0.912460615116783));
#74403=CARTESIAN_POINT('Ctrl Pts',(0.339122181698526,-0.0771254979932333,
-0.896576685042796));
#74404=CARTESIAN_POINT('Ctrl Pts',(0.248610173587816,0.243197816909012,
-0.880692754968808));
#74405=CARTESIAN_POINT('Ctrl Pts',(-0.0696436300603406,0.340737378860454,
-0.864808824894819));
#74406=CARTESIAN_POINT('Ctrl Pts',(-0.270824704599013,0.171070735517887,
-0.852250483857469));
#74407=CARTESIAN_POINT('Ctrl Pts',(-0.294056291535214,0.0366892411458219,
-0.844986786178113));
#74408=CARTESIAN_POINT('Ctrl Pts',(-0.293843481306506,0.000189946096159861,
-0.843017731856754));
#74409=CARTESIAN_POINT('',(-0.294199911255592,-0.000228510835546836,-0.743017611708961));
#74410=CARTESIAN_POINT('Ctrl Pts',(-0.294199939966062,0.0001879467097956,
-0.843017611708961));
#74411=CARTESIAN_POINT('Ctrl Pts',(-0.294210637410069,-0.0165571582630485,
-0.84211534212027));
#74412=CARTESIAN_POINT('Ctrl Pts',(-0.292787354432935,-0.0333086725148639,
-0.841213072531579));
#74413=CARTESIAN_POINT('Ctrl Pts',(-0.289953095943817,-0.0498080530897905,
-0.840310802942887));
#74414=CARTESIAN_POINT('Ctrl Pts',(-0.287118308400922,-0.0663105135036494,
-0.839408364933025));
#74415=CARTESIAN_POINT('Ctrl Pts',(-0.282872182508555,-0.0825599868555481,
-0.838505926923162));
#74416=CARTESIAN_POINT('Ctrl Pts',(-0.277288867949126,-0.0983083094732686,
-0.837603488913299));
#74417=CARTESIAN_POINT('Ctrl Pts',(-0.271690760042274,-0.114098358274486,
-0.83669865983647));
#74418=CARTESIAN_POINT('Ctrl Pts',(-0.264748691178075,-0.12938388715599,
-0.83579383075964));
#74419=CARTESIAN_POINT('Ctrl Pts',(-0.25658515980724,-0.143936429602423,
-0.834889001682811));
#74420=CARTESIAN_POINT('Ctrl Pts',(-0.251027385457895,-0.153843875712752,
-0.834272989370822));
#74421=CARTESIAN_POINT('Ctrl Pts',(-0.24490447653641,-0.163412053346357,
-0.833656977058833));
#74422=CARTESIAN_POINT('Ctrl Pts',(-0.238266280902253,-0.172576995526659,
-0.833040964746843));
#74423=CARTESIAN_POINT('Ctrl Pts',(-0.228587978458964,-0.185939223334441,
-0.832142836129852));
#74424=CARTESIAN_POINT('Ctrl Pts',(-0.217751176956386,-0.198527486544028,
-0.831244707512861));
#74425=CARTESIAN_POINT('Ctrl Pts',(-0.2059043801134,-0.210135732920692,
-0.83034657889587));
#74426=CARTESIAN_POINT('Ctrl Pts',(-0.194080611976174,-0.221721414304158,
-0.829450196129672));
#74427=CARTESIAN_POINT('Ctrl Pts',(-0.18125125798943,-0.232330265407811,
-0.828553813363473));
#74428=CARTESIAN_POINT('Ctrl Pts',(-0.167604216956642,-0.241790128951434,
-0.827657430597274));
#74429=CARTESIAN_POINT('Ctrl Pts',(-0.15395953978733,-0.251248353910849,
-0.826761203097442));
#74430=CARTESIAN_POINT('Ctrl Pts',(-0.139498074974674,-0.259557493260994,
-0.825864975597611));
#74431=CARTESIAN_POINT('Ctrl Pts',(-0.124439628937701,-0.266586606471232,
-0.824968748097779));
#74432=CARTESIAN_POINT('Ctrl Pts',(-0.109385224420607,-0.273613833145455,
-0.824072761135466));
#74433=CARTESIAN_POINT('Ctrl Pts',(-0.0937348787508753,-0.279361390572878,
-0.823176774173154));
#74434=CARTESIAN_POINT('Ctrl Pts',(-0.077730153362982,-0.283745772229592,
-0.822280787210842));
#74435=CARTESIAN_POINT('Ctrl Pts',(-0.0616869810780328,-0.288140686142631,
-0.821382647889294));
#74436=CARTESIAN_POINT('Ctrl Pts',(-0.0452885024722155,-0.291165699290351,
-0.820484508567746));
#74437=CARTESIAN_POINT('Ctrl Pts',(-0.0287887795740931,-0.292788056741791,
-0.819586369246198));
#74438=CARTESIAN_POINT('Ctrl Pts',(-0.013912339536594,-0.294250802722118,
-0.818776591055083));
#74439=CARTESIAN_POINT('Ctrl Pts',(0.00104585912408567,-0.294574000697571,
-0.817966812863969));
#74440=CARTESIAN_POINT('Ctrl Pts',(0.0159001287712503,-0.293770022134761,
-0.817157034672855));
#74441=CARTESIAN_POINT('Ctrl Pts',(0.032375065736724,-0.292878325911485,
-0.816258906055864));
#74442=CARTESIAN_POINT('Ctrl Pts',(0.0488274363991952,-0.290593563992844,
-0.815360777438873));
#74443=CARTESIAN_POINT('Ctrl Pts',(0.0650035903451627,-0.286928864428517,
-0.814462648821881));
#74444=CARTESIAN_POINT('Ctrl Pts',(0.0811482998513748,-0.283271288586248,
-0.813566266055683));
#74445=CARTESIAN_POINT('Ctrl Pts',(0.0970170808011161,-0.278239207841102,
-0.812669883289484));
#74446=CARTESIAN_POINT('Ctrl Pts',(0.112363417068298,-0.271897227835695,
-0.811773500523286));
#74447=CARTESIAN_POINT('Ctrl Pts',(0.127707095129677,-0.26555634635229,
-0.810877273023454));
#74448=CARTESIAN_POINT('Ctrl Pts',(0.142527758658779,-0.257906268324901,
-0.809981045523622));
#74449=CARTESIAN_POINT('Ctrl Pts',(0.156596237021465,-0.249060752730568,
-0.80908481802379));
#74450=CARTESIAN_POINT('Ctrl Pts',(0.170660939560616,-0.2402176111745,-0.808188831061478));
#74451=CARTESIAN_POINT('Ctrl Pts',(0.183973193177795,-0.230180099550807,
-0.807292844099165));
#74452=CARTESIAN_POINT('Ctrl Pts',(0.196331900105423,-0.219105967515707,
-0.806396857136852));
#74453=CARTESIAN_POINT('Ctrl Pts',(0.2087202953858,-0.208005232961414,-0.805498717815304));
#74454=CARTESIAN_POINT('Ctrl Pts',(0.220149994497017,-0.195863454534986,
-0.804600578493756));
#74455=CARTESIAN_POINT('Ctrl Pts',(0.230455776249653,-0.182876393209102,
-0.803702439172208));
#74456=CARTESIAN_POINT('Ctrl Pts',(0.239747650133175,-0.171167030556742,
-0.802892660981095));
#74457=CARTESIAN_POINT('Ctrl Pts',(0.248126161128695,-0.158771357214758,
-0.802082882789981));
#74458=CARTESIAN_POINT('Ctrl Pts',(0.255501069045883,-0.145852129625902,
-0.801273104598868));
#74459=CARTESIAN_POINT('Ctrl Pts',(0.263680612432935,-0.131523356470108,
-0.800374975981877));
#74460=CARTESIAN_POINT('Ctrl Pts',(0.270677196238584,-0.116458548058095,
-0.799476847364886));
#74461=CARTESIAN_POINT('Ctrl Pts',(0.276364382311608,-0.100877986644874,
-0.798578718747895));
#74462=CARTESIAN_POINT('Ctrl Pts',(0.2820405131993,-0.0853277119132891,
-0.797682335981696));
#74463=CARTESIAN_POINT('Ctrl Pts',(0.286411968193491,-0.0692643863955023,
-0.796785953215497));
#74464=CARTESIAN_POINT('Ctrl Pts',(0.289399437368199,-0.0529301960224028,
-0.795889570449299));
#74465=CARTESIAN_POINT('Ctrl Pts',(0.292386389070347,-0.0365988349656295,
-0.794993342949467));
#74466=CARTESIAN_POINT('Ctrl Pts',(0.293989636672718,-0.0199974688051808,
-0.794097115449635));
#74467=CARTESIAN_POINT('Ctrl Pts',(0.294180579340224,-0.00338034599560538,
-0.793200887949803));
#74468=CARTESIAN_POINT('Ctrl Pts',(0.294371470760837,0.0132323169625333,
-0.792304900987491));
#74469=CARTESIAN_POINT('Ctrl Pts',(0.293150811423026,0.0298599363575227,
-0.791408914025179));
#74470=CARTESIAN_POINT('Ctrl Pts',(0.290542184814657,0.0462480144776586,
-0.790512927062866));
#74471=CARTESIAN_POINT('Ctrl Pts',(0.287927291707098,0.0626754603930689,
-0.789614787741318));
#74472=CARTESIAN_POINT('Ctrl Pts',(0.283917922998519,0.0788614348057531,
-0.78871664841977));
#74473=CARTESIAN_POINT('Ctrl Pts',(0.278589050834782,0.0945609896044634,
-0.787818509098222));
#74474=CARTESIAN_POINT('Ctrl Pts',(0.27378444607258,0.108715984025915,-0.787008730907108));
#74475=CARTESIAN_POINT('Ctrl Pts',(0.267908051971126,0.122475350162049,
-0.786198952715993));
#74476=CARTESIAN_POINT('Ctrl Pts',(0.261047741200663,0.135675041234678,
-0.785389174524879));
#74477=CARTESIAN_POINT('Ctrl Pts',(0.253438939812809,0.150314877695889,
-0.784491045907888));
#74478=CARTESIAN_POINT('Ctrl Pts',(0.244570447328582,0.164359466636021,
-0.783592917290896));
#74479=CARTESIAN_POINT('Ctrl Pts',(0.234558862771465,0.177583163321744,
-0.782694788673905));
#74480=CARTESIAN_POINT('Ctrl Pts',(0.224566739494724,0.190781154778953,
-0.781798405907706));
#74481=CARTESIAN_POINT('Ctrl Pts',(0.213436354176119,0.203160757685192,
-0.780902023141507));
#74482=CARTESIAN_POINT('Ctrl Pts',(0.201328255727785,0.214524062626102,
-0.780005640375309));
#74483=CARTESIAN_POINT('Ctrl Pts',(0.189222254575975,0.225885399279419,
-0.779109412875477));
#74484=CARTESIAN_POINT('Ctrl Pts',(0.176139415511457,0.23623020876436,-0.778213185375645));
#74485=CARTESIAN_POINT('Ctrl Pts',(0.162277907574574,0.245396659947152,
-0.777316957875813));
#74486=CARTESIAN_POINT('Ctrl Pts',(0.148420119912662,0.254560650956125,
-0.776420970913501));
#74487=CARTESIAN_POINT('Ctrl Pts',(0.133784744616074,0.262546483780045,
-0.775524983951189));
#74488=CARTESIAN_POINT('Ctrl Pts',(0.118598442542028,0.269236047784477,
-0.774628996988877));
#74489=CARTESIAN_POINT('Ctrl Pts',(0.103375659605088,0.275941681604068,
-0.773730857667329));
#74490=CARTESIAN_POINT('Ctrl Pts',(0.0876000447295265,0.28134453089193,
-0.77283271834578));
#74491=CARTESIAN_POINT('Ctrl Pts',(0.0715180844246416,0.285374847525548,
-0.771934579024232));
#74492=CARTESIAN_POINT('Ctrl Pts',(0.0570183064805997,0.289008651808344,
-0.771124800833118));
#74493=CARTESIAN_POINT('Ctrl Pts',(0.0422701359153877,0.291527308014146,
-0.770315022642004));
#74494=CARTESIAN_POINT('Ctrl Pts',(0.0274590616356825,0.292915755694513,
-0.76950524445089));
#74495=CARTESIAN_POINT('Ctrl Pts',(0.0110320328456341,0.294455689232631,
-0.768607115833899));
#74496=CARTESIAN_POINT('Ctrl Pts',(-0.00557746613309338,0.294614374820569,
-0.767708987216908));
#74497=CARTESIAN_POINT('Ctrl Pts',(-0.0221166107849677,0.293367509324714,
-0.766810858599917));
#74498=CARTESIAN_POINT('Ctrl Pts',(-0.0386236053881212,0.292123067580951,
-0.765914475833718));
#74499=CARTESIAN_POINT('Ctrl Pts',(-0.0550597320389343,0.289478490833111,
-0.765018093067519));
#74500=CARTESIAN_POINT('Ctrl Pts',(-0.0711716553977228,0.285461443049579,
-0.76412171030132));
#74501=CARTESIAN_POINT('Ctrl Pts',(-0.087280787940025,0.281445091076406,
-0.763225482801488));
#74502=CARTESIAN_POINT('Ctrl Pts',(-0.10306505022713,0.276056879376787,
-0.762329255301656));
#74503=CARTESIAN_POINT('Ctrl Pts',(-0.118281038042414,0.269375641140043,
-0.761433027801824));
#74504=CARTESIAN_POINT('Ctrl Pts',(-0.133492942055352,0.262696196073529,
-0.760537040839512));
#74505=CARTESIAN_POINT('Ctrl Pts',(-0.148136153775957,0.254724741597121,
-0.759641053877199));
#74506=CARTESIAN_POINT('Ctrl Pts',(-0.161988569885976,0.245587750562393,
-0.758745066914886));
#74507=CARTESIAN_POINT('Ctrl Pts',(-0.175874262569211,0.236428810450427,
-0.757846927593338));
#74508=CARTESIAN_POINT('Ctrl Pts',(-0.188964716392098,0.226099201365837,
-0.75694878827179));
#74509=CARTESIAN_POINT('Ctrl Pts',(-0.201067726873874,0.214768268628709,
-0.756050648950241));
#74510=CARTESIAN_POINT('Ctrl Pts',(-0.211980013753884,0.204552100607387,
-0.755240870759128));
#74511=CARTESIAN_POINT('Ctrl Pts',(-0.222089754032483,0.193522807085033,
-0.754431092568016));
#74512=CARTESIAN_POINT('Ctrl Pts',(-0.231283761504503,0.181828110214918,
-0.753621314376903));
#74513=CARTESIAN_POINT('Ctrl Pts',(-0.241474226249487,0.168865928432832,
-0.752723771479215));
#74514=CARTESIAN_POINT('Ctrl Pts',(-0.250605506517791,0.155001277538237,
-0.751826228581528));
#74515=CARTESIAN_POINT('Ctrl Pts',(-0.258519464715208,0.140432639950129,
-0.750928685683841));
#74516=CARTESIAN_POINT('Ctrl Pts',(-0.266417571192186,0.125893183457555,
-0.750032940571629));
#74517=CARTESIAN_POINT('Ctrl Pts',(-0.273102759340644,0.110653192248535,
-0.749137195459416));
#74518=CARTESIAN_POINT('Ctrl Pts',(-0.278460120528183,0.0949399877576883,
-0.748241450347204));
#74519=CARTESIAN_POINT('Ctrl Pts',(-0.283815402235698,0.0792328824066407,
-0.747346052921848));
#74520=CARTESIAN_POINT('Ctrl Pts',(-0.28784357491228,0.06305365788728,-0.746450655496491));
#74521=CARTESIAN_POINT('Ctrl Pts',(-0.29047804426146,0.0466491779352817,
-0.745555258071135));
#74522=CARTESIAN_POINT('Ctrl Pts',(-0.292966827964608,0.031151862555292,
-0.74470937595041));
#74523=CARTESIAN_POINT('Ctrl Pts',(-0.294212092345077,0.015454226645856,
-0.743863493829685));
#74524=CARTESIAN_POINT('Ctrl Pts',(-0.294199911255592,-0.000228510835546836,
-0.743017611708961));
#74525=CARTESIAN_POINT('',(-0.294239083931547,-6.59995884866487E-5,-0.643017618234341));
#74526=CARTESIAN_POINT('Ctrl Pts',(-0.293927949640422,-0.000230402592847965,
-0.743017498174503));
#74527=CARTESIAN_POINT('Ctrl Pts',(-0.294163664674453,-0.0328317124483067,
-0.741257460217307));
#74528=CARTESIAN_POINT('Ctrl Pts',(-0.274118262007807,-0.163224061780253,
-0.734202778902116));
#74529=CARTESIAN_POINT('Ctrl Pts',(-0.0830108472164328,-0.33772976742521,
-0.721853454228924));
#74530=CARTESIAN_POINT('Ctrl Pts',(0.2388379518494,-0.252801561144413,-0.70596952415494));
#74531=CARTESIAN_POINT('Ctrl Pts',(0.341896895248078,0.0637080024832001,
-0.690085594080949));
#74532=CARTESIAN_POINT('Ctrl Pts',(0.131757823904318,0.321857223626676,
-0.674201664006963));
#74533=CARTESIAN_POINT('Ctrl Pts',(-0.195025494420267,0.28561555261962,
-0.658512362449674));
#74534=CARTESIAN_POINT('Ctrl Pts',(-0.294378853579128,0.0937945108140465,
-0.648117704250382));
#74535=CARTESIAN_POINT('Ctrl Pts',(-0.294665467861281,-6.47855231172667E-5,
-0.643017689409085));
#74536=CARTESIAN_POINT('',(-0.294199877779988,0.000268168305674158,-0.543017614213059));
#74537=CARTESIAN_POINT('Ctrl Pts',(-0.294199992571974,-6.61108953689901E-5,
-0.64301761170896));
#74538=CARTESIAN_POINT('Ctrl Pts',(-0.294199189049575,-0.00364186466996765,
-0.642823009092302));
#74539=CARTESIAN_POINT('Ctrl Pts',(-0.294133197574971,-0.00721680678781066,
-0.642628406475644));
#74540=CARTESIAN_POINT('Ctrl Pts',(-0.294002091898632,-0.0107893447080197,
-0.642433803858986));
#74541=CARTESIAN_POINT('Ctrl Pts',(-0.293397013910515,-0.0272772963938953,
-0.641535675242002));
#74542=CARTESIAN_POINT('Ctrl Pts',(-0.291398688453342,-0.0437669092700093,
-0.640637546625017));
#74543=CARTESIAN_POINT('Ctrl Pts',(-0.288015830853521,-0.0600043429907858,
-0.639739418008031));
#74544=CARTESIAN_POINT('Ctrl Pts',(-0.284639549109885,-0.076210213151524,
-0.638843035241837));
#74545=CARTESIAN_POINT('Ctrl Pts',(-0.2798841721558,-0.0921640978031815,
-0.637946652475643));
#74546=CARTESIAN_POINT('Ctrl Pts',(-0.273810009185595,-0.107618394662737,
-0.637050269709449));
#74547=CARTESIAN_POINT('Ctrl Pts',(-0.267736898347642,-0.123070014616149,
-0.636154042209622));
#74548=CARTESIAN_POINT('Ctrl Pts',(-0.260345694194456,-0.138021464794339,
-0.635257814709794));
#74549=CARTESIAN_POINT('Ctrl Pts',(-0.251746153444292,-0.152241631054067,
-0.634361587209967));
#74550=CARTESIAN_POINT('Ctrl Pts',(-0.243148920715475,-0.16645798077891,
-0.633465600247659));
#74551=CARTESIAN_POINT('Ctrl Pts',(-0.233344414141136,-0.179942764306823,
-0.63256961328535));
#74552=CARTESIAN_POINT('Ctrl Pts',(-0.222486862627603,-0.192492171160612,
-0.631673626323042));
#74553=CARTESIAN_POINT('Ctrl Pts',(-0.211603228869283,-0.205071724470632,
-0.630775487001498));
#74554=CARTESIAN_POINT('Ctrl Pts',(-0.199662037835341,-0.216710829325282,
-0.629877347679954));
#74555=CARTESIAN_POINT('Ctrl Pts',(-0.186856147860634,-0.227240885420482,
-0.62897920835841));
#74556=CARTESIAN_POINT('Ctrl Pts',(-0.175310132480963,-0.236734968991724,
-0.628169430167271));
#74557=CARTESIAN_POINT('Ctrl Pts',(-0.163062027674604,-0.245327762063203,
-0.627359651976133));
#74558=CARTESIAN_POINT('Ctrl Pts',(-0.150272996084734,-0.25292620790997,
-0.626549873784995));
#74559=CARTESIAN_POINT('Ctrl Pts',(-0.136088623894679,-0.261353678215219,
-0.625651745168002));
#74560=CARTESIAN_POINT('Ctrl Pts',(-0.121147757200918,-0.268611166753299,
-0.624753616551009));
#74561=CARTESIAN_POINT('Ctrl Pts',(-0.105668446312975,-0.27456842399264,
-0.623855487934016));
#74562=CARTESIAN_POINT('Ctrl Pts',(-0.0902192252881835,-0.280514101061752,
-0.622959105167816));
#74563=CARTESIAN_POINT('Ctrl Pts',(-0.074234343983909,-0.285164220968364,
-0.622062722401616));
#74564=CARTESIAN_POINT('Ctrl Pts',(-0.0579545725884968,-0.288435274396327,
-0.621166339635415));
#74565=CARTESIAN_POINT('Ctrl Pts',(-0.0416776210832624,-0.291705761230865,
-0.620270112135582));
#74566=CARTESIAN_POINT('Ctrl Pts',(-0.0251066440073686,-0.293597448313603,
-0.619373884635749));
#74567=CARTESIAN_POINT('Ctrl Pts',(-0.00849535403158956,-0.294077317996268,
-0.618477657135916));
#74568=CARTESIAN_POINT('Ctrl Pts',(0.00811147765822207,-0.294557058887232,
-0.617581670173603));
#74569=CARTESIAN_POINT('Ctrl Pts',(0.0247578090422277,-0.293625722525604,
-0.616685683211289));
#74570=CARTESIAN_POINT('Ctrl Pts',(0.0411887707946803,-0.291302463361406,
-0.615789696248976));
#74571=CARTESIAN_POINT('Ctrl Pts',(0.057659203358391,-0.288973623213857,
-0.614891556927427));
#74572=CARTESIAN_POINT('Ctrl Pts',(0.0739124495281757,-0.285246319352522,
-0.613993417605877));
#74573=CARTESIAN_POINT('Ctrl Pts',(0.0897022945351791,-0.280191253173835,
-0.613095278284328));
#74574=CARTESIAN_POINT('Ctrl Pts',(0.103938696194503,-0.275633516698123,
-0.612285500093223));
#74575=CARTESIAN_POINT('Ctrl Pts',(0.11779816678023,-0.269997273340848,
-0.611475721902117));
#74576=CARTESIAN_POINT('Ctrl Pts',(0.131115156296434,-0.26336752986912,
-0.610665943711012));
#74577=CARTESIAN_POINT('Ctrl Pts',(0.145885088986696,-0.25601445170442,
-0.609767815094021));
#74578=CARTESIAN_POINT('Ctrl Pts',(0.160081768982187,-0.247391522124171,
-0.608869686477029));
#74579=CARTESIAN_POINT('Ctrl Pts',(0.173477558121661,-0.237611398775702,
-0.607971557860038));
#74580=CARTESIAN_POINT('Ctrl Pts',(0.186847307506206,-0.227850286775689,
-0.607075175093839));
#74581=CARTESIAN_POINT('Ctrl Pts',(0.199418585369986,-0.216936853845187,
-0.60617879232764));
#74582=CARTESIAN_POINT('Ctrl Pts',(0.210990720430563,-0.205028183165612,
-0.60528240956144));
#74583=CARTESIAN_POINT('Ctrl Pts',(0.222560851031175,-0.193121575238805,
-0.604386182061608));
#74584=CARTESIAN_POINT('Ctrl Pts',(0.233131594441001,-0.180220600661988,
-0.603489954561776));
#74585=CARTESIAN_POINT('Ctrl Pts',(0.242537698025042,-0.166520584423409,
-0.602593727061943));
#74586=CARTESIAN_POINT('Ctrl Pts',(0.251941277115219,-0.15282424511722,
-0.601697740099631));
#74587=CARTESIAN_POINT('Ctrl Pts',(0.260180397664757,-0.138329948703318,
-0.600801753137317));
#74588=CARTESIAN_POINT('Ctrl Pts',(0.26713302548195,-0.123262267936543,
-0.599905766175004));
#74589=CARTESIAN_POINT('Ctrl Pts',(0.274102355051873,-0.108158391261543,
-0.599007626853456));
#74590=CARTESIAN_POINT('Ctrl Pts',(0.279778710291323,-0.0924791120585587,
-0.598109487531907));
#74591=CARTESIAN_POINT('Ctrl Pts',(0.284088067458913,-0.076469666714718,
-0.597211348210358));
#74592=CARTESIAN_POINT('Ctrl Pts',(0.287973459589404,-0.0620352695335585,
-0.596401570019246));
#74593=CARTESIAN_POINT('Ctrl Pts',(0.290748191564568,-0.047333125929017,
-0.595591791828134));
#74594=CARTESIAN_POINT('Ctrl Pts',(0.29239397973829,-0.0325484348748805,
-0.594782013637021));
#74595=CARTESIAN_POINT('Ctrl Pts',(0.294219330769654,-0.0161506678384154,
-0.593883885020032));
#74596=CARTESIAN_POINT('Ctrl Pts',(0.294666815678933,0.000453560378974142,
-0.592985756403042));
#74597=CARTESIAN_POINT('Ctrl Pts',(0.293707738630449,0.01701188609731,-0.592087627786052));
#74598=CARTESIAN_POINT('Ctrl Pts',(0.29275052590896,0.0335380244813062,
-0.591191245019855));
#74599=CARTESIAN_POINT('Ctrl Pts',(0.290392157559051,0.0500176526379714,
-0.590294862253658));
#74600=CARTESIAN_POINT('Ctrl Pts',(0.28665588810683,0.0661969924821711,
-0.58939847948746));
#74601=CARTESIAN_POINT('Ctrl Pts',(0.282920265830129,0.0823735298323798,
-0.58850225198763));
#74602=CARTESIAN_POINT('Ctrl Pts',(0.277807342070079,0.0982491013777121,
-0.5876060244878));
#74603=CARTESIAN_POINT('Ctrl Pts',(0.271391705529629,0.113578968870645,
-0.58670979698797));
#74604=CARTESIAN_POINT('Ctrl Pts',(0.264977790874861,0.12890472199719,-0.585813810025659));
#74605=CARTESIAN_POINT('Ctrl Pts',(0.257262173147636,0.143684335627127,
-0.584917823063348));
#74606=CARTESIAN_POINT('Ctrl Pts',(0.248367443912265,0.157693540782392,
-0.584021836101037));
#74607=CARTESIAN_POINT('Ctrl Pts',(0.239451347566184,0.171736399152903,
-0.583123696779491));
#74608=CARTESIAN_POINT('Ctrl Pts',(0.229350930809813,0.185004495718582,
-0.582225557457944));
#74609=CARTESIAN_POINT('Ctrl Pts',(0.218232171105833,0.197302710306864,
-0.581327418136398));
#74610=CARTESIAN_POINT('Ctrl Pts',(0.2082073020186,0.208390996638846,-0.580517639945277));
#74611=CARTESIAN_POINT('Ctrl Pts',(0.197355474857132,0.218690997190556,
-0.579707861754155));
#74612=CARTESIAN_POINT('Ctrl Pts',(0.185822421239044,0.228086974123599,
-0.578898083563034));
#74613=CARTESIAN_POINT('Ctrl Pts',(0.173031059839962,0.238508094204016,
-0.577999954946041));
#74614=CARTESIAN_POINT('Ctrl Pts',(0.159319426709137,0.247883154434612,
-0.577101826329047));
#74615=CARTESIAN_POINT('Ctrl Pts',(0.144884055439066,0.256051265334756,
-0.576203697712053));
#74616=CARTESIAN_POINT('Ctrl Pts',(0.13047674474283,0.264203498438984,-0.575307314945851));
#74617=CARTESIAN_POINT('Ctrl Pts',(0.115349136709595,0.271152996309403,
-0.57441093217965));
#74618=CARTESIAN_POINT('Ctrl Pts',(0.0997271091365789,0.276781761868915,
-0.573514549413449));
#74619=CARTESIAN_POINT('Ctrl Pts',(0.0841077875230671,0.282409552445405,
-0.572618321913614));
#74620=CARTESIAN_POINT('Ctrl Pts',(0.0679949407084323,0.286716747448818,
-0.571722094413779));
#74621=CARTESIAN_POINT('Ctrl Pts',(0.0516346710183764,0.289633390251925,
-0.570825866913945));
#74622=CARTESIAN_POINT('Ctrl Pts',(0.0352787922432276,0.292549250260458,
-0.56992987995163));
#74623=CARTESIAN_POINT('Ctrl Pts',(0.0186764037705013,0.294075170627267,
-0.569033892989315));
#74624=CARTESIAN_POINT('Ctrl Pts',(0.00208242171189055,0.294192629954956,
-0.568137906027));
#74625=CARTESIAN_POINT('Ctrl Pts',(-0.0145514227688778,0.29431037144598,
-0.567239766705449));
#74626=CARTESIAN_POINT('Ctrl Pts',(-0.031176025375635,0.293012914973375,
-0.566341627383898));
#74627=CARTESIAN_POINT('Ctrl Pts',(-0.0475374527293351,0.290333998332965,
-0.565443488062348));
#74628=CARTESIAN_POINT('Ctrl Pts',(-0.0622892030740751,0.287918640025931,
-0.564633709871247));
#74629=CARTESIAN_POINT('Ctrl Pts',(-0.0768266663317771,0.284381080679814,
-0.563823931680146));
#74630=CARTESIAN_POINT('Ctrl Pts',(-0.0909735945032452,0.279781066377193,
-0.563014153489045));
#74631=CARTESIAN_POINT('Ctrl Pts',(-0.10666401587162,0.274679169920671,
-0.562116024872055));
#74632=CARTESIAN_POINT('Ctrl Pts',(-0.121974090607168,0.268236946000983,
-0.561217896255065));
#74633=CARTESIAN_POINT('Ctrl Pts',(-0.136662092220278,0.260532363728532,
-0.560319767638075));
#74634=CARTESIAN_POINT('Ctrl Pts',(-0.151321542177458,0.252842758209756,
-0.559423384871878));
#74635=CARTESIAN_POINT('Ctrl Pts',(-0.165360595717803,0.243895969895092,
-0.558527002105681));
#74636=CARTESIAN_POINT('Ctrl Pts',(-0.178557669351488,0.2338178750989,-0.557630619339483));
#74637=CARTESIAN_POINT('Ctrl Pts',(-0.191752457062515,0.223741525973444,
-0.556734391839652));
#74638=CARTESIAN_POINT('Ctrl Pts',(-0.204104895076259,0.212534696074499,
-0.555838164339822));
#74639=CARTESIAN_POINT('Ctrl Pts',(-0.215422811901074,0.20036629485179,
-0.554941936839991));
#74640=CARTESIAN_POINT('Ctrl Pts',(-0.226737691122558,0.188201159492991,
-0.55404594987768));
#74641=CARTESIAN_POINT('Ctrl Pts',(-0.237018069032917,0.175075552231487,
-0.553149962915369));
#74642=CARTESIAN_POINT('Ctrl Pts',(-0.246110223385262,0.16119366595886,
-0.552253975953058));
#74643=CARTESIAN_POINT('Ctrl Pts',(-0.255224219107198,0.147278432319156,
-0.551355836631511));
#74644=CARTESIAN_POINT('Ctrl Pts',(-0.263143876780439,0.132603970575454,
-0.550457697309964));
#74645=CARTESIAN_POINT('Ctrl Pts',(-0.269759925279849,0.117401970652158,
-0.549559557988417));
#74646=CARTESIAN_POINT('Ctrl Pts',(-0.275725070839879,0.103695580447476,
-0.548749779797297));
#74647=CARTESIAN_POINT('Ctrl Pts',(-0.280630983945998,0.0895610772477883,
-0.547940001606177));
#74648=CARTESIAN_POINT('Ctrl Pts',(-0.284432353931144,0.0751789600698787,
-0.547130223415058));
#74649=CARTESIAN_POINT('Ctrl Pts',(-0.289819157500309,0.0547985076411929,
-0.545982711842335));
#74650=CARTESIAN_POINT('Ctrl Pts',(-0.29301713345713,0.0338165504288796,
-0.544835200269612));
#74651=CARTESIAN_POINT('Ctrl Pts',(-0.293928020853791,0.0126474723551179,
-0.543687688696889));
#74652=CARTESIAN_POINT('Ctrl Pts',(-0.294105321143291,0.0085270029264237,
-0.543464330535613));
#74653=CARTESIAN_POINT('Ctrl Pts',(-0.29419611198676,0.00439951374748332,
-0.543240972374336));
#74654=CARTESIAN_POINT('Ctrl Pts',(-0.294199877779988,0.000268168305674158,
-0.543017614213059));
#74655=CARTESIAN_POINT('',(-0.293740379894572,-8.66858914495487E-5,-0.443017611708961));
#74656=CARTESIAN_POINT('Ctrl Pts',(-0.294123668879967,0.000268052534830647,
-0.543017611708961));
#74657=CARTESIAN_POINT('Ctrl Pts',(-0.293474798752899,-0.0722898843115431,
-0.539093838919663));
#74658=CARTESIAN_POINT('Ctrl Pts',(-0.229758782171269,-0.243774078952558,
-0.52987542277237));
#74659=CARTESIAN_POINT('Ctrl Pts',(0.0577531094952713,-0.342953021424431,
-0.515362363267081));
#74660=CARTESIAN_POINT('Ctrl Pts',(0.319517415892196,-0.137334691550856,
-0.499478433193093));
#74661=CARTESIAN_POINT('Ctrl Pts',(0.288584649791592,0.194090433725029,
-0.483594503119105));
#74662=CARTESIAN_POINT('Ctrl Pts',(-0.00670892406185214,0.347717107571907,
-0.467710573045117));
#74663=CARTESIAN_POINT('Ctrl Pts',(-0.252926720822328,0.207297382700659,
-0.454184942575068));
#74664=CARTESIAN_POINT('Ctrl Pts',(-0.293596658076772,0.0543905486936848,
-0.445953955463017));
#74665=CARTESIAN_POINT('Ctrl Pts',(-0.293740379894572,-8.66858914495487E-5,
-0.443017611708961));
#74666=CARTESIAN_POINT('',(-0.29419991353495,-0.000225557150586184,-0.343017611708961));
#74667=CARTESIAN_POINT('Ctrl Pts',(-0.293740379894572,-8.66858914495487E-5,
-0.443017611708961));
#74668=CARTESIAN_POINT('Ctrl Pts',(-0.293855808854661,-0.0438396152167057,
-0.440659312105021));
#74669=CARTESIAN_POINT('Ctrl Pts',(-0.26416141467023,-0.185673782245695,
-0.433006369143085));
#74670=CARTESIAN_POINT('Ctrl Pts',(-0.0444810415613786,-0.344925547768942,
-0.420058782823151));
#74671=CARTESIAN_POINT('Ctrl Pts',(0.265767271674193,-0.224321095562353,
-0.404174852749164));
#74672=CARTESIAN_POINT('Ctrl Pts',(0.332556860575699,0.101774903304964,
-0.388290922675176));
#74673=CARTESIAN_POINT('Ctrl Pts',(0.0947044659440234,0.334639000613301,
-0.372406992601186));
#74674=CARTESIAN_POINT('Ctrl Pts',(-0.213699718700967,0.264631837550187,
-0.357315928117542));
#74675=CARTESIAN_POINT('Ctrl Pts',(-0.293736313474251,0.0827916910960814,
-0.347519506991888));
#74676=CARTESIAN_POINT('Ctrl Pts',(-0.294441777086296,-0.000223575550274286,
-0.343017729224232));
#74677=CARTESIAN_POINT('',(-0.29419991634408,0.000221862877645845,-0.24301761170896));
#74678=CARTESIAN_POINT('Ctrl Pts',(-0.29419991353495,-0.000225557150586184,
-0.343017611708961));
#74679=CARTESIAN_POINT('Ctrl Pts',(-0.294188713844001,-0.0148335981727865,
-0.342224785290378));
#74680=CARTESIAN_POINT('Ctrl Pts',(-0.293089342069403,-0.0294007671736424,
-0.341431958871795));
#74681=CARTESIAN_POINT('Ctrl Pts',(-0.29092083917617,-0.0438030288111792,
-0.340639132453213));
#74682=CARTESIAN_POINT('Ctrl Pts',(-0.288464318379726,-0.0601181812321631,
-0.339741003798971));
#74683=CARTESIAN_POINT('Ctrl Pts',(-0.284623211539265,-0.0762782108728595,
-0.338842875144731));
#74684=CARTESIAN_POINT('Ctrl Pts',(-0.279434741703112,-0.0920318701826437,
-0.337944746490492));
#74685=CARTESIAN_POINT('Ctrl Pts',(-0.274256357608409,-0.107754906333829,
-0.337048363686894));
#74686=CARTESIAN_POINT('Ctrl Pts',(-0.267735991130414,-0.123072376354419,
-0.336151980883297));
#74687=CARTESIAN_POINT('Ctrl Pts',(-0.259961429584258,-0.13774503667468,
-0.3352555980797));
#74688=CARTESIAN_POINT('Ctrl Pts',(-0.252188214706506,-0.152415155474376,
-0.334359370542789));
#74689=CARTESIAN_POINT('Ctrl Pts',(-0.243161558549959,-0.1664399642326,
-0.333463143005878));
#74690=CARTESIAN_POINT('Ctrl Pts',(-0.233016526606927,-0.179602166824466,
-0.332566915468968));
#74691=CARTESIAN_POINT('Ctrl Pts',(-0.222874217479038,-0.192760836825726,
-0.331670928469684));
#74692=CARTESIAN_POINT('Ctrl Pts',(-0.211614620329887,-0.205056739759931,
-0.330774941470401));
#74693=CARTESIAN_POINT('Ctrl Pts',(-0.199413918088511,-0.216304713939823,
-0.329878954471117));
#74694=CARTESIAN_POINT('Ctrl Pts',(-0.18718390707091,-0.227579708233123,
-0.328980815113556));
#74695=CARTESIAN_POINT('Ctrl Pts',(-0.174008877979855,-0.237801226458742,
-0.328082675755996));
#74696=CARTESIAN_POINT('Ctrl Pts',(-0.160099435859406,-0.246823440210811,
-0.327184536398434));
#74697=CARTESIAN_POINT('Ctrl Pts',(-0.147558441841444,-0.254958024453204,
-0.326374758392032));
#74698=CARTESIAN_POINT('Ctrl Pts',(-0.134421234178903,-0.262118040987156,
-0.325564980385629));
#74699=CARTESIAN_POINT('Ctrl Pts',(-0.12085842293712,-0.268229158752646,
-0.324755202379225));
#74700=CARTESIAN_POINT('Ctrl Pts',(-0.105815845975774,-0.275007027858723,
-0.323857073830079));
#74701=CARTESIAN_POINT('Ctrl Pts',(-0.0901532297157309,-0.280537222332166,
-0.322958945280933));
#74702=CARTESIAN_POINT('Ctrl Pts',(-0.0741018957635367,-0.284714855678888,
-0.322060816731786));
#74703=CARTESIAN_POINT('Ctrl Pts',(-0.058081763614756,-0.28888436822426,
-0.321164434033202));
#74704=CARTESIAN_POINT('Ctrl Pts',(-0.041675154056802,-0.291706277349181,
-0.320268051334619));
#74705=CARTESIAN_POINT('Ctrl Pts',(-0.0251307049024998,-0.293124696453751,
-0.319371668636035));
#74706=CARTESIAN_POINT('Ctrl Pts',(-0.00858912146014023,-0.29454286986984,
-0.318475441202494));
#74707=CARTESIAN_POINT('Ctrl Pts',(0.00808947256198928,-0.294557915573295,
-0.317579213768953));
#74708=CARTESIAN_POINT('Ctrl Pts',(0.0246492605735305,-0.293165574297492,
-0.316682986335411));
#74709=CARTESIAN_POINT('Ctrl Pts',(0.0412046041325439,-0.291773606709727,
-0.315786999438783));
#74710=CARTESIAN_POINT('Ctrl Pts',(0.0576404169237435,-0.288975079092548,
-0.314891012542154));
#74711=CARTESIAN_POINT('Ctrl Pts',(0.0737056036461875,-0.284817703085941,
-0.313995025645526));
#74712=CARTESIAN_POINT('Ctrl Pts',(0.0898093825526996,-0.280650340129113,
-0.313096886387282));
#74713=CARTESIAN_POINT('Ctrl Pts',(0.105539994156818,-0.275117833834768,
-0.312198747129039));
#74714=CARTESIAN_POINT('Ctrl Pts',(0.120660743004417,-0.268318141573808,
-0.311300607870795));
#74715=CARTESIAN_POINT('Ctrl Pts',(0.134293882340815,-0.262187416636001,
-0.310490829348942));
#74716=CARTESIAN_POINT('Ctrl Pts',(0.147431126491672,-0.255027447201575,
-0.309681050827089));
#74717=CARTESIAN_POINT('Ctrl Pts',(0.159917541947552,-0.246941328613606,
-0.308871272305237));
#74718=CARTESIAN_POINT('Ctrl Pts',(0.173766275644202,-0.237972981904336,
-0.307973143683613));
#74719=CARTESIAN_POINT('Ctrl Pts',(0.186902508977528,-0.227807353077535,
-0.30707501506199));
#74720=CARTESIAN_POINT('Ctrl Pts',(0.199112726159464,-0.216581998978092,
-0.306176886440368));
#74721=CARTESIAN_POINT('Ctrl Pts',(0.211299208177787,-0.205378465589304,
-0.305280503670556));
#74722=CARTESIAN_POINT('Ctrl Pts',(0.222562626326639,-0.193119776588182,
-0.304384120900744));
#74723=CARTESIAN_POINT('Ctrl Pts',(0.232721259355089,-0.179984597797094,
-0.303487738130932));
#74724=CARTESIAN_POINT('Ctrl Pts',(0.242878132744514,-0.166851694230745,
-0.302591510629068));
#74725=CARTESIAN_POINT('Ctrl Pts',(0.251930076201204,-0.152843193943631,
-0.301695283127205));
#74726=CARTESIAN_POINT('Ctrl Pts',(0.259734865287855,-0.138171776256586,
-0.300799055625341));
#74727=CARTESIAN_POINT('Ctrl Pts',(0.267537559648178,-0.123504296229425,
-0.29990306866186));
#74728=CARTESIAN_POINT('Ctrl Pts',(0.274093401812665,-0.108174956070798,
-0.299007081698379));
#74729=CARTESIAN_POINT('Ctrl Pts',(0.279306402374615,-0.0924206340194086,
-0.298111094734898));
#74730=CARTESIAN_POINT('Ctrl Pts',(0.284531925710785,-0.0766284666204733,
-0.297212955413612));
#74731=CARTESIAN_POINT('Ctrl Pts',(0.28840793992237,-0.060410041305751,
-0.296314816092326));
#74732=CARTESIAN_POINT('Ctrl Pts',(0.290888486288432,-0.0440173664003702,
-0.295416676771039));
#74733=CARTESIAN_POINT('Ctrl Pts',(0.293124990440893,-0.0292374429135893,
-0.294606898591108));
#74734=CARTESIAN_POINT('Ctrl Pts',(0.294227760402243,-0.0143164490420228,
-0.293797120411177));
#74735=CARTESIAN_POINT('Ctrl Pts',(0.294199467913316,0.000559535094423254,
-0.292987342231246));
#74736=CARTESIAN_POINT('Ctrl Pts',(0.294168088578443,0.0170585602944459,
-0.292089213376404));
#74737=CARTESIAN_POINT('Ctrl Pts',(0.292744361366393,0.0336076926620605,
-0.291191084521562));
#74738=CARTESIAN_POINT('Ctrl Pts',(0.289928169666838,0.049952942191998,
-0.29029295566672));
#74739=CARTESIAN_POINT('Ctrl Pts',(0.287117452289695,0.0662664186129436,
-0.289396572661394));
#74740=CARTESIAN_POINT('Ctrl Pts',(0.282919710800327,0.0823760166686528,
-0.288500189656069));
#74741=CARTESIAN_POINT('Ctrl Pts',(0.277386608168404,0.0980321865961808,
-0.287603806650743));
#74742=CARTESIAN_POINT('Ctrl Pts',(0.271854463958668,0.113685644623779,
-0.286707578913342));
#74743=CARTESIAN_POINT('Ctrl Pts',(0.264987630655919,0.128885068807038,
-0.285811351175941));
#74744=CARTESIAN_POINT('Ctrl Pts',(0.256887762185586,0.143395668132903,
-0.28491512343854));
#74745=CARTESIAN_POINT('Ctrl Pts',(0.248790067633381,0.157902372968997,
-0.284019136239084));
#74746=CARTESIAN_POINT('Ctrl Pts',(0.239460390207801,0.171719933886316,
-0.283123149039629));
#74747=CARTESIAN_POINT('Ctrl Pts',(0.22904577855072,0.184639300605517,-0.282227161840174));
#74748=CARTESIAN_POINT('Ctrl Pts',(0.218606148761602,0.197589702415902,
-0.281329022287198));
#74749=CARTESIAN_POINT('Ctrl Pts',(0.207076898786055,0.20963699823115,-0.280430882734223));
#74750=CARTESIAN_POINT('Ctrl Pts',(0.194644907688949,0.220605983397461,
-0.279532743181248));
#74751=CARTESIAN_POINT('Ctrl Pts',(0.18343602537139,0.230495796132352,-0.278722966173252));
#74752=CARTESIAN_POINT('Ctrl Pts',(0.171494140039145,0.239509279579548,
-0.277913189165257));
#74753=CARTESIAN_POINT('Ctrl Pts',(0.15897708025623,0.247547829627335,-0.277103412157261));
#74754=CARTESIAN_POINT('Ctrl Pts',(0.145094340803253,0.256463429442994,
-0.276205284049544));
#74755=CARTESIAN_POINT('Ctrl Pts',(0.130414881329146,0.264236061930519,
-0.275307155941827));
#74756=CARTESIAN_POINT('Ctrl Pts',(0.115152090863427,0.270727974117528,
-0.27440902783411));
#74757=CARTESIAN_POINT('Ctrl Pts',(0.0999189693705288,0.277207266831928,
-0.27351264557611));
#74758=CARTESIAN_POINT('Ctrl Pts',(0.0841054616494478,0.282410413744088,
-0.27261626331811));
#74759=CARTESIAN_POINT('Ctrl Pts',(0.0679492881810552,0.286245583783729,
-0.27171988106011));
#74760=CARTESIAN_POINT('Ctrl Pts',(0.0517959130334674,0.290080089554932,
-0.270823654059488));
#74761=CARTESIAN_POINT('Ctrl Pts',(0.035300745405137,0.292546854929202,
-0.269927427058865));
#74762=CARTESIAN_POINT('Ctrl Pts',(0.0187161961879273,0.293604059917868,
-0.269031200058243));
#74763=CARTESIAN_POINT('Ctrl Pts',(0.00213609800764407,0.294660981169039,
-0.268135213591109));
#74764=CARTESIAN_POINT('Ctrl Pts',(-0.014532543310271,0.294309053444057,
-0.267239227123975));
#74765=CARTESIAN_POINT('Ctrl Pts',(-0.0310343467477303,0.292558557082068,
-0.266343240656841));
#74766=CARTESIAN_POINT('Ctrl Pts',(-0.0475757915097962,0.29080385560427,
-0.265445101813421));
#74767=CARTESIAN_POINT('Ctrl Pts',(-0.0639488101679096,0.287643985310027,
-0.264546962970001));
#74768=CARTESIAN_POINT('Ctrl Pts',(-0.0799048785991908,0.283141043255916,
-0.263648824126582));
#74769=CARTESIAN_POINT('Ctrl Pts',(-0.094291202113307,0.279081096945536,
-0.262839043445477));
#74770=CARTESIAN_POINT('Ctrl Pts',(-0.108338323302757,0.273930182240347,
-0.262029262764373));
#74771=CARTESIAN_POINT('Ctrl Pts',(-0.121877834764577,0.267767498761703,
-0.261219482083269));
#74772=CARTESIAN_POINT('Ctrl Pts',(-0.136894524488037,0.260932458522351,
-0.260321353279546));
#74773=CARTESIAN_POINT('Ctrl Pts',(-0.151382464382951,0.252808400843108,
-0.259423224475822));
#74774=CARTESIAN_POINT('Ctrl Pts',(-0.165110236460511,0.243499999622082,
-0.258525095672099));
#74775=CARTESIAN_POINT('Ctrl Pts',(-0.178811323349849,0.234209692847645,
-0.257628712726046));
#74776=CARTESIAN_POINT('Ctrl Pts',(-0.191754490863578,0.223739996567545,
-0.256732329779993));
#74777=CARTESIAN_POINT('Ctrl Pts',(-0.203733726773965,0.212240921065641,
-0.255835946833939));
#74778=CARTESIAN_POINT('Ctrl Pts',(-0.215710887536314,0.200743837534187,
-0.254939719167181));
#74779=CARTESIAN_POINT('Ctrl Pts',(-0.226723842192841,0.188218236884438,
-0.254043491500424));
#74780=CARTESIAN_POINT('Ctrl Pts',(-0.236600645961076,0.174853579691128,
-0.253147263833665));
#74781=CARTESIAN_POINT('Ctrl Pts',(-0.246474798830406,0.161492509524142,
-0.252251276711217));
#74782=CARTESIAN_POINT('Ctrl Pts',(-0.255212944291058,0.14729347302781,
-0.251355289588768));
#74783=CARTESIAN_POINT('Ctrl Pts',(-0.262685312828353,0.132476663696934,
-0.250459302466319));
#74784=CARTESIAN_POINT('Ctrl Pts',(-0.27017563152706,0.117624261351904,
-0.249561162999083));
#74785=CARTESIAN_POINT('Ctrl Pts',(-0.276393765841537,0.10215184385304,
-0.248663023531846));
#74786=CARTESIAN_POINT('Ctrl Pts',(-0.281257209132088,0.0863019253042985,
-0.24776488406461));
#74787=CARTESIAN_POINT('Ctrl Pts',(-0.285642169789093,0.0720113774144976,
-0.246955106712834));
#74788=CARTESIAN_POINT('Ctrl Pts',(-0.28892645453844,0.0574146248080487,
-0.246145329361058));
#74789=CARTESIAN_POINT('Ctrl Pts',(-0.291085350888058,0.0426961180715054,
-0.245335552009283));
#74790=CARTESIAN_POINT('Ctrl Pts',(-0.293145255725698,0.0286524965540629,
-0.244562905242508));
#74791=CARTESIAN_POINT('Ctrl Pts',(-0.294189181828774,0.014456301457929,
-0.243790258475734));
#74792=CARTESIAN_POINT('Ctrl Pts',(-0.29419991634408,0.000221862877645845,
-0.24301761170896));
#74793=CARTESIAN_POINT('',(-0.293744537661632,9.25662168771693E-5,-0.14301761170896));
#74794=CARTESIAN_POINT('Ctrl Pts',(-0.29445204848288,0.000219819995411468,
-0.243017490604234));
#74795=CARTESIAN_POINT('Ctrl Pts',(-0.293751335212956,-0.0831599735004281,
-0.238495534381254));
#74796=CARTESIAN_POINT('Ctrl Pts',(-0.213104386102375,-0.265350741380069,
-0.228678934800286));
#74797=CARTESIAN_POINT('Ctrl Pts',(0.0959768626644768,-0.334276361929609,
-0.213567691861301));
#74798=CARTESIAN_POINT('Ctrl Pts',(0.332941212592535,-0.100509168556688,
-0.197683761787325));
#74799=CARTESIAN_POINT('Ctrl Pts',(0.264912791059908,0.225330331614917,
-0.181799831713324));
#74800=CARTESIAN_POINT('Ctrl Pts',(-0.0457940858542747,0.344753966870199,
-0.165915901639349));
#74801=CARTESIAN_POINT('Ctrl Pts',(-0.264522476343154,0.184916985358244,
-0.152988494971215));
#74802=CARTESIAN_POINT('Ctrl Pts',(-0.293866212551352,0.0434698093785783,
-0.145355731661092));
#74803=CARTESIAN_POINT('Ctrl Pts',(-0.293744537661632,9.25662168771693E-5,
-0.14301761170896));
#74804=CARTESIAN_POINT('',(-0.294186798250996,-0.000261260174532603,-0.0430176117089603));
#74805=CARTESIAN_POINT('Ctrl Pts',(-0.293744537661632,9.25662168771693E-5,
-0.14301761170896));
#74806=CARTESIAN_POINT('Ctrl Pts',(-0.293590681286969,-0.0547574146716426,
-0.140061088303096));
#74807=CARTESIAN_POINT('Ctrl Pts',(-0.252507336188254,-0.208049626619383,
-0.131809921539239));
#74808=CARTESIAN_POINT('Ctrl Pts',(-0.00537683585382717,-0.347740876544168,
-0.118264111417372));
#74809=CARTESIAN_POINT('Ctrl Pts',(0.289302873605603,-0.192989859491775,
-0.102380181343396));
#74810=CARTESIAN_POINT('Ctrl Pts',(0.319027026718357,0.138546274126025,
-0.0864962512693962));
#74811=CARTESIAN_POINT('Ctrl Pts',(0.0563826028718357,0.343175568089735,
-0.0706123211954191));
#74812=CARTESIAN_POINT('Ctrl Pts',(-0.230176223724105,0.243028826433064,
-0.0561194413419322));
#74813=CARTESIAN_POINT('Ctrl Pts',(-0.293533328381349,0.0719298853820162,
-0.0469212048464487));
#74814=CARTESIAN_POINT('Ctrl Pts',(-0.294186798250996,-0.000261260174532603,
-0.0430176117089603));
#74815=CARTESIAN_POINT('',(-0.288932402895451,-0.0555047265699091,-0.0399922440470373));
#74816=CARTESIAN_POINT('Origin',(0.000858955019862939,0.000109716591558141,
-0.0410049673081075));
#74817=CARTESIAN_POINT('',(-0.2942,-3.60291088309151E-17,-0.04));
#74818=CARTESIAN_POINT('Origin',(0.,0.,-0.04));
#74819=CARTESIAN_POINT('',(-0.221686865784453,0.193412961144454,-0.04));
#74820=CARTESIAN_POINT('Origin',(0.,0.,-0.04));
#74821=CARTESIAN_POINT('',(-0.293768185304944,0.000119558705670028,-0.128582388291039));
#74822=CARTESIAN_POINT('Ctrl Pts',(-0.221686865784453,0.193412961144454,
-0.04));
#74823=CARTESIAN_POINT('Ctrl Pts',(-0.157343740137231,0.267162030364559,
-0.0452946433579961));
#74824=CARTESIAN_POINT('Ctrl Pts',(0.0496182053170372,0.34411773810001,
-0.0558839300739825));
#74825=CARTESIAN_POINT('Ctrl Pts',(0.316630310046587,0.144421010344727,
-0.0717678601479819));
#74826=CARTESIAN_POINT('Ctrl Pts',(0.292700980788135,-0.18764014656629,
-0.087651790221959));
#74827=CARTESIAN_POINT('Ctrl Pts',(0.00108527138476461,-0.347774759775002,
-0.103535720295958));
#74828=CARTESIAN_POINT('Ctrl Pts',(-0.250450798406577,-0.211692488319999,
-0.117179252985643));
#74829=CARTESIAN_POINT('Ctrl Pts',(-0.293565247741175,-0.0565344194021568,
-0.125528142317339));
#74830=CARTESIAN_POINT('Ctrl Pts',(-0.293768185304944,0.000119558705670028,
-0.128582388291039));
#74831=CARTESIAN_POINT('',(-0.294499934166686,0.000202248616450143,-0.228582388291039));
#74832=CARTESIAN_POINT('Ctrl Pts',(-0.293768185304944,0.000119558705670028,
-0.128582388291039));
#74833=CARTESIAN_POINT('Ctrl Pts',(-0.293917047181479,0.0416772542730101,
-0.130822785675335));
#74834=CARTESIAN_POINT('Ctrl Pts',(-0.266241884141502,0.181253034476232,
-0.13835782641764));
#74835=CARTESIAN_POINT('Ctrl Pts',(-0.0521444580392835,0.343851119474212,
-0.151187510517905));
#74836=CARTESIAN_POINT('Ctrl Pts',(0.260721659465963,0.230172071351022,
-0.167071440591914));
#74837=CARTESIAN_POINT('Ctrl Pts',(0.33473384718524,-0.0943598456158883,
-0.182955370665886));
#74838=CARTESIAN_POINT('Ctrl Pts',(0.102118851543616,-0.332451723718594,
-0.198839300739887));
#74839=CARTESIAN_POINT('Ctrl Pts',(-0.210188708599208,-0.268822006024866,
-0.214048306614925));
#74840=CARTESIAN_POINT('Ctrl Pts',(-0.293831058097356,-0.0849440524174718,
-0.223962669131982));
#74841=CARTESIAN_POINT('Ctrl Pts',(-0.294499934166686,0.000202248616450143,
-0.228582388291039));
#74842=CARTESIAN_POINT('',(-0.294199900939987,-0.000241426803754268,-0.328582388291039));
#74843=CARTESIAN_POINT('Ctrl Pts',(-0.294499934166686,0.000202248616450143,
-0.228582388291039));
#74844=CARTESIAN_POINT('Ctrl Pts',(-0.294597654532305,0.0126418141050379,
-0.229257312489979));
#74845=CARTESIAN_POINT('Ctrl Pts',(-0.288230516942064,0.122566455283741,
-0.235226880046917));
#74846=CARTESIAN_POINT('Ctrl Pts',(-0.149881191576857,0.313827796561115,
-0.246491090961838));
#74847=CARTESIAN_POINT('Ctrl Pts',(0.182509282439241,0.296044952328845,
-0.262375021035839));
#74848=CARTESIAN_POINT('Ctrl Pts',(0.347709976704713,0.00706718636026016,
-0.278258951109817));
#74849=CARTESIAN_POINT('Ctrl Pts',(0.194387712086192,-0.288384529274392,
-0.294142881183814));
#74850=CARTESIAN_POINT('Ctrl Pts',(-0.137005426269588,-0.319658767853967,
-0.310026811257793));
#74851=CARTESIAN_POINT('Ctrl Pts',(-0.285807358002809,-0.130626349168447,
-0.321506646960211));
#74852=CARTESIAN_POINT('Ctrl Pts',(-0.294536173334788,-0.0166712251748063,
-0.327691839304621));
#74853=CARTESIAN_POINT('Ctrl Pts',(-0.294390515183554,-0.000241583225926489,
-0.328582388291039));
#74854=CARTESIAN_POINT('',(-0.294157183091672,-5.80760838105538E-5,-0.42858238548701));
#74855=CARTESIAN_POINT('Ctrl Pts',(-0.294199900939987,-0.000241426803754268,
-0.328582388291039));
#74856=CARTESIAN_POINT('Ctrl Pts',(-0.294213270623952,0.0160507149000982,
-0.329466063430325));
#74857=CARTESIAN_POINT('Ctrl Pts',(-0.292869010815876,0.0323914039133056,
-0.330349738569611));
#74858=CARTESIAN_POINT('Ctrl Pts',(-0.290169337604126,0.0485324171495974,
-0.331233413708898));
#74859=CARTESIAN_POINT('Ctrl Pts',(-0.287471170605857,0.0646644249212218,
-0.332116595824287));
#74860=CARTESIAN_POINT('Ctrl Pts',(-0.283419155016342,0.0805961649708263,
-0.332999777939676));
#74861=CARTESIAN_POINT('Ctrl Pts',(-0.278067392711698,0.0960841563969761,
-0.333882960055066));
#74862=CARTESIAN_POINT('Ctrl Pts',(-0.272718393432816,0.111564151631051,
-0.334765686198235));
#74863=CARTESIAN_POINT('Ctrl Pts',(-0.26607124562374,0.126600080193668,
-0.335648412341405));
#74864=CARTESIAN_POINT('Ctrl Pts',(-0.258229490017853,0.140965139254781,
-0.336531138484574));
#74865=CARTESIAN_POINT('Ctrl Pts',(-0.250369454528004,0.155363684645478,
-0.337415922346994));
#74866=CARTESIAN_POINT('Ctrl Pts',(-0.24130966072791,0.169087525650376,
-0.338300706209414));
#74867=CARTESIAN_POINT('Ctrl Pts',(-0.231199034706483,0.181935830310553,
-0.339185490071835));
#74868=CARTESIAN_POINT('Ctrl Pts',(-0.221260465597484,0.194565489792372,
-0.340055217183148));
#74869=CARTESIAN_POINT('Ctrl Pts',(-0.210307190680362,0.206348733223679,
-0.340924944294462));
#74870=CARTESIAN_POINT('Ctrl Pts',(-0.198515397572668,0.217129631617993,
-0.341794671405776));
#74871=CARTESIAN_POINT('Ctrl Pts',(-0.186338536628284,0.228262586496369,
-0.342692799959873));
#74872=CARTESIAN_POINT('Ctrl Pts',(-0.173183301635518,0.238403611496796,
-0.34359092851397));
#74873=CARTESIAN_POINT('Ctrl Pts',(-0.159236740552278,0.247380881351584,
-0.344489057068068));
#74874=CARTESIAN_POINT('Ctrl Pts',(-0.145317289883835,0.256340700488015,
-0.345385439769729));
#74875=CARTESIAN_POINT('Ctrl Pts',(-0.130610188431077,0.264140775701221,
-0.34628182247139));
#74876=CARTESIAN_POINT('Ctrl Pts',(-0.115334224409597,0.270650432624514,
-0.347178205173051));
#74877=CARTESIAN_POINT('Ctrl Pts',(-0.100060906431591,0.277158961970183,
-0.348074432606764));
#74878=CARTESIAN_POINT('Ctrl Pts',(-0.0842196265633046,0.282377158592839,
-0.348970660040477));
#74879=CARTESIAN_POINT('Ctrl Pts',(-0.068052101713687,0.286221158289093,
-0.349866887474189));
#74880=CARTESIAN_POINT('Ctrl Pts',(-0.0518889160665153,0.290064126294161,
-0.350762874369396));
#74881=CARTESIAN_POINT('Ctrl Pts',(-0.0354004320327606,0.292533456912791,
-0.351658861264602));
#74882=CARTESIAN_POINT('Ctrl Pts',(-0.0188400964165087,0.293596135476979,
-0.352554848159809));
#74883=CARTESIAN_POINT('Ctrl Pts',(-0.00223997920574037,0.294661366830478,
-0.353452987414012));
#74884=CARTESIAN_POINT('Ctrl Pts',(0.0144315393077484,0.294313172550085,
-0.354351126668216));
#74885=CARTESIAN_POINT('Ctrl Pts',(0.0309190160886215,0.292570768266605,
-0.355249265922419));
#74886=CARTESIAN_POINT('Ctrl Pts',(0.0457844219475074,0.29099978519937,
-0.356059044441533));
#74887=CARTESIAN_POINT('Ctrl Pts',(0.0604998238938433,0.28829621433199,
-0.356868822960646));
#74888=CARTESIAN_POINT('Ctrl Pts',(0.0748858560541141,0.28450966339132,
-0.357678601479759));
#74889=CARTESIAN_POINT('Ctrl Pts',(0.0908414629000977,0.280309984324951,
-0.358576730132563));
#74890=CARTESIAN_POINT('Ctrl Pts',(0.106493703337533,0.274750485260366,
-0.359474858785367));
#74891=CARTESIAN_POINT('Ctrl Pts',(0.121596801359752,0.267895236798038,
-0.36037298743817));
#74892=CARTESIAN_POINT('Ctrl Pts',(0.13667054084219,0.261053314084136,-0.361269370240835));
#74893=CARTESIAN_POINT('Ctrl Pts',(0.151196517023994,0.252920904648086,
-0.362165753043499));
#74894=CARTESIAN_POINT('Ctrl Pts',(0.164946334766074,0.243611056085799,
-0.363062135846163));
#74895=CARTESIAN_POINT('Ctrl Pts',(0.178693770849512,0.234302820118071,
-0.363958363382926));
#74896=CARTESIAN_POINT('Ctrl Pts',(0.191664632259472,0.223817948321669,
-0.364854590919689));
#74897=CARTESIAN_POINT('Ctrl Pts',(0.203657436356593,0.212314127218752,
-0.365750818456452));
#74898=CARTESIAN_POINT('Ctrl Pts',(0.21564702172256,0.200813393609558,-0.366646805456017));
#74899=CARTESIAN_POINT('Ctrl Pts',(0.226658506983278,0.188294809460885,
-0.367542792455582));
#74900=CARTESIAN_POINT('Ctrl Pts',(0.236526786088971,0.174953477994643,
-0.368438779455147));
#74901=CARTESIAN_POINT('Ctrl Pts',(0.246418770984156,0.161580097698824,
-0.369336918813697));
#74902=CARTESIAN_POINT('Ctrl Pts',(0.25516161318444,0.14738067742214,-0.370235058172247));
#74903=CARTESIAN_POINT('Ctrl Pts',(0.262633018972394,0.132580305269848,
-0.371133197530796));
#74904=CARTESIAN_POINT('Ctrl Pts',(0.269369367887219,0.119236033292566,
-0.371942975538448));
#74905=CARTESIAN_POINT('Ctrl Pts',(0.275072596195384,0.105403996273835,
-0.372752753546101));
#74906=CARTESIAN_POINT('Ctrl Pts',(0.279687183289654,0.0912618184319138,
-0.373562531553753));
#74907=CARTESIAN_POINT('Ctrl Pts',(0.284805243636515,0.0755766621758177,
-0.374460660167658));
#74908=CARTESIAN_POINT('Ctrl Pts',(0.288616098892701,0.059409472625499,
-0.375358788781564));
#74909=CARTESIAN_POINT('Ctrl Pts',(0.291040390595721,0.0430015237159115,
-0.37625691739547));
#74910=CARTESIAN_POINT('Ctrl Pts',(0.293459969776135,0.026625469825425,
-0.377153300158664));
#74911=CARTESIAN_POINT('Ctrl Pts',(0.294498155584544,0.0100103497840362,
-0.378049682921857));
#74912=CARTESIAN_POINT('Ctrl Pts',(0.29412616962601,-0.00659062524587472,
-0.378946065685051));
#74913=CARTESIAN_POINT('Ctrl Pts',(0.293754248100716,-0.023188724751655,
-0.379842293182046));
#74914=CARTESIAN_POINT('Ctrl Pts',(0.291972604312582,-0.0397718940807069,
-0.380738520679042));
#74915=CARTESIAN_POINT('Ctrl Pts',(0.288804560090822,-0.0560853463103032,
-0.381634748176038));
#74916=CARTESIAN_POINT('Ctrl Pts',(0.285637366136683,-0.0723944201918616,
-0.382530735135603));
#74917=CARTESIAN_POINT('Ctrl Pts',(0.281084671958776,-0.088433145512489,
-0.383426722095167));
#74918=CARTESIAN_POINT('Ctrl Pts',(0.275220959321368,-0.103957027421074,
-0.384322709054731));
#74919=CARTESIAN_POINT('Ctrl Pts',(0.269343160745391,-0.119518201137842,
-0.385220848373739));
#74920=CARTESIAN_POINT('Ctrl Pts',(0.262148359134826,-0.134561326912255,
-0.386118987692747));
#74921=CARTESIAN_POINT('Ctrl Pts',(0.253759438487147,-0.148861638371637,
-0.387017127011756));
#74922=CARTESIAN_POINT('Ctrl Pts',(0.246195840097746,-0.161755050678741,
-0.387826905217082));
#74923=CARTESIAN_POINT('Ctrl Pts',(0.237662404096809,-0.17404458450177,
-0.388636683422409));
#74924=CARTESIAN_POINT('Ctrl Pts',(0.228278315073844,-0.185587313324609,
-0.389446461627736));
#74925=CARTESIAN_POINT('Ctrl Pts',(0.217870380203778,-0.198389405197028,
-0.390344590236663));
#74926=CARTESIAN_POINT('Ctrl Pts',(0.206348879583428,-0.210354172454429,
-0.391242718845589));
#74927=CARTESIAN_POINT('Ctrl Pts',(0.19387356937472,-0.22128415916623,-0.392140847454516));
#74928=CARTESIAN_POINT('Ctrl Pts',(0.181422509627243,-0.232192899334694,
-0.393037230212426));
#74929=CARTESIAN_POINT('Ctrl Pts',(0.168021865344104,-0.242070286298685,
-0.393933612970336));
#74930=CARTESIAN_POINT('Ctrl Pts',(0.153868837590726,-0.250754901883251,
-0.394829995728246));
#74931=CARTESIAN_POINT('Ctrl Pts',(0.139718261348546,-0.259438013165506,
-0.395726223219565));
#74932=CARTESIAN_POINT('Ctrl Pts',(0.124816205105695,-0.266928305295534,
-0.396622450710884));
#74933=CARTESIAN_POINT('Ctrl Pts',(0.109389430956506,-0.273107290995704,
-0.397518678202204));
#74934=CARTESIAN_POINT('Ctrl Pts',(0.0939667971847902,-0.279284618323684,
-0.398414665155865));
#74935=CARTESIAN_POINT('Ctrl Pts',(0.0780204640726392,-0.284151053523581,
-0.399310652109527));
#74936=CARTESIAN_POINT('Ctrl Pts',(0.0617962714351649,-0.287636682008244,
-0.400206639063189));
#74937=CARTESIAN_POINT('Ctrl Pts',(0.0455331046921821,-0.291130683744837,
-0.401104778376037));
#74938=CARTESIAN_POINT('Ctrl Pts',(0.0289915280435265,-0.293237112583825,
-0.402002917688885));
#74939=CARTESIAN_POINT('Ctrl Pts',(0.0124270340977167,-0.293937423312402,
-0.402901057001733));
#74940=CARTESIAN_POINT('Ctrl Pts',(-0.00250780557758506,-0.294568835807611,
-0.403710835235065));
#74941=CARTESIAN_POINT('Ctrl Pts',(-0.0174607700916445,-0.294057914770964,
-0.404520613468396));
#74942=CARTESIAN_POINT('Ctrl Pts',(-0.0322471498142642,-0.292427360773332,
-0.405330391701728));
#74943=CARTESIAN_POINT('Ctrl Pts',(-0.048646789004516,-0.290618906118236,
-0.406228520324142));
#74944=CARTESIAN_POINT('Ctrl Pts',(-0.0649462617435838,-0.287420808342489,
-0.407126648946555));
#74945=CARTESIAN_POINT('Ctrl Pts',(-0.080893043439246,-0.282860310971929,
-0.408024777568969));
#74946=CARTESIAN_POINT('Ctrl Pts',(-0.0968088265684688,-0.278308678642819,
-0.408921160340696));
#74947=CARTESIAN_POINT('Ctrl Pts',(-0.112372509131877,-0.272400054959249,
-0.409817543112423));
#74948=CARTESIAN_POINT('Ctrl Pts',(-0.12734155857147,-0.265212683445926,
-0.41071392588415));
#74949=CARTESIAN_POINT('Ctrl Pts',(-0.142308015158101,-0.258026556887908,
-0.41161015338959));
#74950=CARTESIAN_POINT('Ctrl Pts',(-0.156679308818926,-0.249562415881682,
-0.41250638089503));
#74951=CARTESIAN_POINT('Ctrl Pts',(-0.170232964834833,-0.239946614236464,
-0.41340260840047));
#74952=CARTESIAN_POINT('Ctrl Pts',(-0.183782983200655,-0.230333393365145,
-0.414298595368445));
#74953=CARTESIAN_POINT('Ctrl Pts',(-0.196515160067304,-0.219569592394035,
-0.41519458233642));
#74954=CARTESIAN_POINT('Ctrl Pts',(-0.208237501543953,-0.207823922950973,
-0.416090569304395));
#74955=CARTESIAN_POINT('Ctrl Pts',(-0.219988002681964,-0.196050037807606,
-0.416988708631577));
#74956=CARTESIAN_POINT('Ctrl Pts',(-0.230723280434877,-0.183290154585397,
-0.417886847958758));
#74957=CARTESIAN_POINT('Ctrl Pts',(-0.240289280095377,-0.169748937761759,
-0.41878498728594));
#74958=CARTESIAN_POINT('Ctrl Pts',(-0.248914153097114,-0.15753993927359,
-0.419594765449198));
#74959=CARTESIAN_POINT('Ctrl Pts',(-0.25658883481505,-0.144696598236817,
-0.420404543612457));
#74960=CARTESIAN_POINT('Ctrl Pts',(-0.263232295687335,-0.131386447197478,
-0.421214321775715));
#74961=CARTESIAN_POINT('Ctrl Pts',(-0.271109781837181,-0.115603930753049,
-0.422174516527839));
#74962=CARTESIAN_POINT('Ctrl Pts',(-0.277581946799669,-0.0990750858031063,
-0.423134711279964));
#74963=CARTESIAN_POINT('Ctrl Pts',(-0.282524234881432,-0.0820591049467478,
-0.424094906032089));
#74964=CARTESIAN_POINT('Ctrl Pts',(-0.287441843801891,-0.0651280928597843,
-0.425050306081684));
#74965=CARTESIAN_POINT('Ctrl Pts',(-0.290844538262862,-0.0477153541178306,
-0.426005706131278));
#74966=CARTESIAN_POINT('Ctrl Pts',(-0.292656388079449,-0.0300978158059859,
-0.426961106180873));
#74967=CARTESIAN_POINT('Ctrl Pts',(-0.293681269090984,-0.0201323758890031,
-0.427501532523213));
#74968=CARTESIAN_POINT('Ctrl Pts',(-0.294198011145814,-0.010101755355635,
-0.428041958865554));
#74969=CARTESIAN_POINT('Ctrl Pts',(-0.2941999942651,-5.80897158011377E-5,
-0.428582385207895));
#74970=CARTESIAN_POINT('',(-0.294177705196902,0.000269677437982729,-0.528582388291039));
#74971=CARTESIAN_POINT('Ctrl Pts',(-0.293727096099073,-5.79391349403435E-5,
-0.428582388291039));
#74972=CARTESIAN_POINT('Ctrl Pts',(-0.293634468529128,0.0526122281426488,
-0.43142100947726));
#74973=CARTESIAN_POINT('Ctrl Pts',(-0.254942151327534,0.203650636832815,
-0.439554274021477));
#74974=CARTESIAN_POINT('Ctrl Pts',(-0.0131124674156837,0.347534563923677,
-0.452982181923692));
#74975=CARTESIAN_POINT('Ctrl Pts',(0.284960711564284,0.199373024186178,
-0.468866111997679));
#74976=CARTESIAN_POINT('Ctrl Pts',(0.321992827127266,-0.131426135938866,
-0.484750042071667));
#74977=CARTESIAN_POINT('Ctrl Pts',(0.064060245340413,-0.341831091167,-0.500633972145656));
#74978=CARTESIAN_POINT('Ctrl Pts',(-0.227177597425987,-0.247332674255593,
-0.515244754218778));
#74979=CARTESIAN_POINT('Ctrl Pts',(-0.293497987656841,-0.0740605286863558,
-0.524560892933907));
#74980=CARTESIAN_POINT('Ctrl Pts',(-0.294177705196902,0.000269677437982729,
-0.528582388291039));
#74981=CARTESIAN_POINT('',(-0.294228348185738,-9.78338538022252E-5,-0.62858238829104));
#74982=CARTESIAN_POINT('Ctrl Pts',(-0.294177705196902,0.000269677437982729,
-0.528582388291039));
#74983=CARTESIAN_POINT('Ctrl Pts',(-0.294392894063339,0.0238015592200154,
-0.529855536291904));
#74984=CARTESIAN_POINT('Ctrl Pts',(-0.281052382088353,0.144954516849035,
-0.536423327650765));
#74985=CARTESIAN_POINT('Ctrl Pts',(-0.11361603957044,0.328699871423913,
-0.548285762367618));
#74986=CARTESIAN_POINT('Ctrl Pts',(0.214662148711559,0.273628163448583,
-0.564169692441609));
#74987=CARTESIAN_POINT('Ctrl Pts',(0.34629696365299,-0.0321033158226767,
-0.580053622515595));
#74988=CARTESIAN_POINT('Ctrl Pts',(0.160703037897489,-0.308426236776979,
-0.595937552589584));
#74989=CARTESIAN_POINT('Ctrl Pts',(-0.172104486846384,-0.302212268991917,
-0.611821482663572));
#74990=CARTESIAN_POINT('Ctrl Pts',(-0.29209425334131,-0.108297247891136,
-0.622703094564057));
#74991=CARTESIAN_POINT('Ctrl Pts',(-0.294667300158824,-0.00547889421475271,
-0.628290063106547));
#74992=CARTESIAN_POINT('Ctrl Pts',(-0.294643988261876,-9.79720582637844E-5,
-0.62858238829104));
#74993=CARTESIAN_POINT('',(-0.294199924273098,-0.000211086956616954,-0.728582384448469));
#74994=CARTESIAN_POINT('Ctrl Pts',(-0.294199983736203,-9.78244223404861E-5,
-0.62858238829104));
#74995=CARTESIAN_POINT('Ctrl Pts',(-0.294205426299557,0.016270297276697,
-0.629472949926511));
#74996=CARTESIAN_POINT('Ctrl Pts',(-0.292840578471788,0.0326939988902729,
-0.630363511561983));
#74997=CARTESIAN_POINT('Ctrl Pts',(-0.290103784633613,0.0489227364448709,
-0.631254073197454));
#74998=CARTESIAN_POINT('Ctrl Pts',(-0.287372108214987,0.0651211285428017,
-0.632142969607924));
#74999=CARTESIAN_POINT('Ctrl Pts',(-0.283273643069613,0.0811244831776327,
-0.633031866018394));
#75000=CARTESIAN_POINT('Ctrl Pts',(-0.277858538679389,0.0966864648384387,
-0.633920762428863));
#75001=CARTESIAN_POINT('Ctrl Pts',(-0.272443978612943,0.112246882216077,
-0.634809569487879));
#75002=CARTESIAN_POINT('Ctrl Pts',(-0.265713259877918,0.127365239426204,
-0.635698376546894));
#75003=CARTESIAN_POINT('Ctrl Pts',(-0.257766513752171,0.141809958705487,
-0.63658718360591));
#75004=CARTESIAN_POINT('Ctrl Pts',(-0.249820840153935,0.156252728462466,
-0.637475870707649));
#75005=CARTESIAN_POINT('Ctrl Pts',(-0.240659870035023,0.170021343875504,
-0.638364557809388));
#75006=CARTESIAN_POINT('Ctrl Pts',(-0.230429021010939,0.182910104357142,
-0.639253244911127));
#75007=CARTESIAN_POINT('Ctrl Pts',(-0.220175002415835,0.195828053721404,
-0.640143944602326));
#75008=CARTESIAN_POINT('Ctrl Pts',(-0.208846804315949,0.207861565752943,
-0.641034644293525));
#75009=CARTESIAN_POINT('Ctrl Pts',(-0.196629205242875,0.21883920043163,
-0.641925343984725));
#75010=CARTESIAN_POINT('Ctrl Pts',(-0.189020928018026,0.225675313436242,
-0.642480010260333));
#75011=CARTESIAN_POINT('Ctrl Pts',(-0.181068483165117,0.232102714295101,
-0.643034676535941));
#75012=CARTESIAN_POINT('Ctrl Pts',(-0.172822401357768,0.238088339884453,
-0.643589342811549));
#75013=CARTESIAN_POINT('Ctrl Pts',(-0.159470152672527,0.247780404949165,
-0.64448747142854));
#75014=CARTESIAN_POINT('Ctrl Pts',(-0.145257359119195,0.256376749337958,
-0.645385600045531));
#75015=CARTESIAN_POINT('Ctrl Pts',(-0.130389215186783,0.263727686379293,
-0.646283728662523));
#75016=CARTESIAN_POINT('Ctrl Pts',(-0.115549973084665,0.271064334109479,
-0.647180111428722));
#75017=CARTESIAN_POINT('Ctrl Pts',(-0.100058581207752,0.27715997379475,
-0.648076494194921));
#75018=CARTESIAN_POINT('Ctrl Pts',(-0.0841471422624768,0.281909379852921,
-0.648972876961119));
#75019=CARTESIAN_POINT('Ctrl Pts',(-0.0682384594069048,0.286657963245765,
-0.649869104460951));
#75020=CARTESIAN_POINT('Ctrl Pts',(-0.0519106148113616,0.290060499378108,
-0.650765331960784));
#75021=CARTESIAN_POINT('Ctrl Pts',(-0.0354132269970851,0.292060855565502,
-0.651661559460616));
#75022=CARTESIAN_POINT('Ctrl Pts',(-0.0189202668986979,0.294060674879484,
-0.652557546422929));
#75023=CARTESIAN_POINT('Ctrl Pts',(-0.00225864120250119,0.294658976746293,
-0.653453533385241));
#75024=CARTESIAN_POINT('Ctrl Pts',(0.0143160979546571,0.29385147496542,
-0.654349520347554));
#75025=CARTESIAN_POINT('Ctrl Pts',(0.0309306533082596,0.293042033386325,
-0.655247659669103));
#75026=CARTESIAN_POINT('Ctrl Pts',(0.0474571125141693,0.290820108264942,
-0.656145798990651));
#75027=CARTESIAN_POINT('Ctrl Pts',(0.0636438170329757,0.287233536609974,
-0.6570439383122));
#75028=CARTESIAN_POINT('Ctrl Pts',(0.0782380342004271,0.283999820595795,
-0.657853716503312));
#75029=CARTESIAN_POINT('Ctrl Pts',(0.0925557573170437,0.279657589733852,
-0.658663494694424));
#75030=CARTESIAN_POINT('Ctrl Pts',(0.106424341927058,0.274276319512627,
-0.659473272885536));
#75031=CARTESIAN_POINT('Ctrl Pts',(0.121806051205136,0.268307928619306,
-0.660371401502527));
#75032=CARTESIAN_POINT('Ctrl Pts',(0.136733308829178,0.261022489904615,
-0.661269530119518));
#75033=CARTESIAN_POINT('Ctrl Pts',(0.150969109178701,0.252511322664528,
-0.662167658736509));
#75034=CARTESIAN_POINT('Ctrl Pts',(0.165177236895546,0.244016700079389,
-0.663064041502708));
#75035=CARTESIAN_POINT('Ctrl Pts',(0.178695869870208,0.234301423039947,
-0.663960424268907));
#75036=CARTESIAN_POINT('Ctrl Pts',(0.191310784034313,0.223503521028588,
-0.664856807035106));
#75037=CARTESIAN_POINT('Ctrl Pts',(0.203923513114135,0.212707489368914,
-0.665753034534938));
#75038=CARTESIAN_POINT('Ctrl Pts',(0.215632200183979,0.200829677770462,
-0.66664926203477));
#75039=CARTESIAN_POINT('Ctrl Pts',(0.226254385690265,0.188049442849269,
-0.667545489534601));
#75040=CARTESIAN_POINT('Ctrl Pts',(0.236873720319788,0.175272638001366,
-0.668441476496914));
#75041=CARTESIAN_POINT('Ctrl Pts',(0.246406634503134,0.161594506435376,
-0.669337463459226));
#75042=CARTESIAN_POINT('Ctrl Pts',(0.254711024514696,0.147227490607814,
-0.670233450421538));
#75043=CARTESIAN_POINT('Ctrl Pts',(0.263035363511333,0.132825962024479,
-0.671131589743086));
#75044=CARTESIAN_POINT('Ctrl Pts',(0.270124908995877,0.117732945428985,
-0.672029729064634));
#75045=CARTESIAN_POINT('Ctrl Pts',(0.275883471685441,0.102185860327095,
-0.672927868386182));
#75046=CARTESIAN_POINT('Ctrl Pts',(0.281075492974673,0.0881683352629315,
-0.673737646577296));
#75047=CARTESIAN_POINT('Ctrl Pts',(0.28518606934168,0.0737823933043825,
-0.674547424768411));
#75048=CARTESIAN_POINT('Ctrl Pts',(0.288180019703266,0.0592107781052175,
-0.675357202959525));
#75049=CARTESIAN_POINT('Ctrl Pts',(0.291500623452659,0.0430493344534132,
-0.676255331576516));
#75050=CARTESIAN_POINT('Ctrl Pts',(0.293468083934822,0.0265560104497036,
-0.677153460193507));
#75051=CARTESIAN_POINT('Ctrl Pts',(0.294030695728291,0.00997947741802725,
-0.678051588810499));
#75052=CARTESIAN_POINT('Ctrl Pts',(0.294592213874118,-0.00656483288654887,
-0.678947971576698));
#75053=CARTESIAN_POINT('Ctrl Pts',(0.293754211203151,-0.0231912515321944,
-0.679844354342896));
#75054=CARTESIAN_POINT('Ctrl Pts',(0.291516584350613,-0.0396449372373334,
-0.680740737109095));
#75055=CARTESIAN_POINT('Ctrl Pts',(0.289279345087178,-0.0560957729278373,
-0.681636964608927));
#75056=CARTESIAN_POINT('Ctrl Pts',(0.285643016641729,-0.0723731460790802,
-0.682533192108759));
#75057=CARTESIAN_POINT('Ctrl Pts',(0.280659442297586,-0.0882265121673074,
-0.683429419608591));
#75058=CARTESIAN_POINT('Ctrl Pts',(0.275677205489516,-0.104075623387933,
-0.684325406570904));
#75059=CARTESIAN_POINT('Ctrl Pts',(0.26934868833006,-0.119500201389496,
-0.685221393533216));
#75060=CARTESIAN_POINT('Ctrl Pts',(0.261775411020823,-0.134265685060924,
-0.686117380495529));
#75061=CARTESIAN_POINT('Ctrl Pts',(0.254183941021239,-0.149066638696185,
-0.687015519817077));
#75062=CARTESIAN_POINT('Ctrl Pts',(0.245342124890783,-0.163204640416536,
-0.687913659138625));
#75063=CARTESIAN_POINT('Ctrl Pts',(0.235397357742065,-0.176470178693326,
-0.688811798460173));
#75064=CARTESIAN_POINT('Ctrl Pts',(0.226430980967861,-0.188430621056992,
-0.689621576651286));
#75065=CARTESIAN_POINT('Ctrl Pts',(0.216568876661155,-0.199681890440784,
-0.690431354842399));
#75066=CARTESIAN_POINT('Ctrl Pts',(0.205945555088724,-0.210095379147656,
-0.691241133033512));
#75067=CARTESIAN_POINT('Ctrl Pts',(0.194163181574088,-0.221645026091718,
-0.692139261650503));
#75068=CARTESIAN_POINT('Ctrl Pts',(0.181368533382261,-0.232237363656557,
-0.693037390267494));
#75069=CARTESIAN_POINT('Ctrl Pts',(0.167742570550849,-0.241694166303189,
-0.693935518884485));
#75070=CARTESIAN_POINT('Ctrl Pts',(0.154143094903518,-0.251132586096761,
-0.694831901650684));
#75071=CARTESIAN_POINT('Ctrl Pts',(0.139716117178592,-0.259439351964486,
-0.695728284416883));
#75072=CARTESIAN_POINT('Ctrl Pts',(0.124675749403214,-0.266476260688916,
-0.696624667183082));
#75073=CARTESIAN_POINT('Ctrl Pts',(0.10963798683551,-0.273511950519706,
-0.697520894682914));
#75074=CARTESIAN_POINT('Ctrl Pts',(0.0939877373242821,-0.279277837398947,
-0.698417122182746));
#75075=CARTESIAN_POINT('Ctrl Pts',(0.0779636554399853,-0.283681702671207,
-0.699313349682578));
#75076=CARTESIAN_POINT('Ctrl Pts',(0.0619438742415205,-0.288084385994878,
-0.70020933664489));
#75077=CARTESIAN_POINT('Ctrl Pts',(0.0455512261481134,-0.291125573994551,
-0.701105323607202));
#75078=CARTESIAN_POINT('Ctrl Pts',(0.0290378567090644,-0.292763458918192,
-0.702001310569515));
#75079=CARTESIAN_POINT('Ctrl Pts',(0.0124848184972283,-0.294405278404377,
-0.702899449891063));
#75080=CARTESIAN_POINT('Ctrl Pts',(-0.00418872658918546,-0.294637009672879,
-0.703797589212611));
#75081=CARTESIAN_POINT('Ctrl Pts',(-0.0207268217851637,-0.293468974269319,
-0.704695728534159));
#75082=CARTESIAN_POINT('Ctrl Pts',(-0.0356378589605347,-0.29241585302904,
-0.705505506725273));
#75083=CARTESIAN_POINT('Ctrl Pts',(-0.0504383662596673,-0.290225613820241,
-0.706315284916387));
#75084=CARTESIAN_POINT('Ctrl Pts',(-0.0649473615191108,-0.286941597248823,
-0.707125063107501));
#75085=CARTESIAN_POINT('Ctrl Pts',(-0.0810393531154373,-0.283299279767532,
-0.708023191724492));
#75086=CARTESIAN_POINT('Ctrl Pts',(-0.0968754466213217,-0.278287415851489,
-0.708921320341483));
#75087=CARTESIAN_POINT('Ctrl Pts',(-0.112207786762964,-0.271961491005174,
-0.709819448958474));
#75088=CARTESIAN_POINT('Ctrl Pts',(-0.127510322734392,-0.265647862973248,
-0.710715831724673));
#75089=CARTESIAN_POINT('Ctrl Pts',(-0.142310300624418,-0.25802548146143,
-0.711612214490872));
#75090=CARTESIAN_POINT('Ctrl Pts',(-0.156375532443047,-0.249199383733494,
-0.712508597257071));
#75091=CARTESIAN_POINT('Ctrl Pts',(-0.170438327961547,-0.24037481481243,
-0.713404824756903));
#75092=CARTESIAN_POINT('Ctrl Pts',(-0.183765933494337,-0.230347318014614,
-0.714301052256735));
#75093=CARTESIAN_POINT('Ctrl Pts',(-0.196151505051165,-0.219267478359566,
-0.715197279756567));
#75094=CARTESIAN_POINT('Ctrl Pts',(-0.20853375245797,-0.208190612410582,
-0.716093266718879));
#75095=CARTESIAN_POINT('Ctrl Pts',(-0.219973884915605,-0.196062500219674,
-0.71698925368119));
#75096=CARTESIAN_POINT('Ctrl Pts',(-0.230300111938318,-0.183072385796434,
-0.717885240643502));
#75097=CARTESIAN_POINT('Ctrl Pts',(-0.240651144846651,-0.170051066239714,
-0.71878337996505));
#75098=CARTESIAN_POINT('Ctrl Pts',(-0.249882453865169,-0.156164247347902,
-0.719681519286598));
#75099=CARTESIAN_POINT('Ctrl Pts',(-0.257863992289351,-0.141632628587475,
-0.720579658608146));
#75100=CARTESIAN_POINT('Ctrl Pts',(-0.265060287554879,-0.128530665816827,
-0.72138943679926));
#75101=CARTESIAN_POINT('Ctrl Pts',(-0.271241047516034,-0.114905308191939,
-0.722199214990374));
#75102=CARTESIAN_POINT('Ctrl Pts',(-0.276344608604166,-0.100932142033202,
-0.723008993181488));
#75103=CARTESIAN_POINT('Ctrl Pts',(-0.282853432122522,-0.0831114731023674,
-0.724041743303208));
#75104=CARTESIAN_POINT('Ctrl Pts',(-0.287644757357304,-0.0646316025977172,
-0.725074493424929));
#75105=CARTESIAN_POINT('Ctrl Pts',(-0.290611796733505,-0.0458085537790022,
-0.726107243546649));
#75106=CARTESIAN_POINT('Ctrl Pts',(-0.292982115349434,-0.0307711318352943,
-0.726932290513922));
#75107=CARTESIAN_POINT('Ctrl Pts',(-0.29418894365814,-0.0155151878871746,
-0.727757337481196));
#75108=CARTESIAN_POINT('Ctrl Pts',(-0.294199924273098,-0.000211086956616954,
-0.728582384448469));
#75109=CARTESIAN_POINT('',(-0.294199926155906,0.000208446298696108,-0.828582392147458));
#75110=CARTESIAN_POINT('Ctrl Pts',(-0.293886246767337,-0.000210790693305624,
-0.728582388291039));
#75111=CARTESIAN_POINT('Ctrl Pts',(-0.293464789150248,0.0634728800831282,
-0.732019233279185));
#75112=CARTESIAN_POINT('Ctrl Pts',(-0.241834069345054,0.225887162901957,
-0.740750721625328));
#75113=CARTESIAN_POINT('Ctrl Pts',(0.0260766885068273,0.34680284923634,
-0.754776853329467));
#75114=CARTESIAN_POINT('Ctrl Pts',(0.30558513020711,0.166041976976387,-0.770660783403452));
#75115=CARTESIAN_POINT('Ctrl Pts',(0.305159306794442,-0.166823281944281,
-0.786544713477441));
#75116=CARTESIAN_POINT('Ctrl Pts',(0.0251892979955619,-0.346868432101308,
-0.802428643551431));
#75117=CARTESIAN_POINT('Ctrl Pts',(-0.242152253072789,-0.225385360111962,
-0.816441201822627));
#75118=CARTESIAN_POINT('Ctrl Pts',(-0.29346671564659,-0.0632269917679521,
-0.825159116735832));
#75119=CARTESIAN_POINT('Ctrl Pts',(-0.293880751489893,0.000208148696046392,
-0.828582388291039));
#75120=CARTESIAN_POINT('',(-0.294226564582519,0.000102116486780654,-0.92858238829104));
#75121=CARTESIAN_POINT('Ctrl Pts',(-0.294199926155906,0.000208446298696108,
-0.828582392147458));
#75122=CARTESIAN_POINT('Ctrl Pts',(-0.294186382166594,0.0193243561534274,
-0.82961286660516));
#75123=CARTESIAN_POINT('Ctrl Pts',(-0.29230559241569,0.0383650065048286,
-0.830643341062863));
#75124=CARTESIAN_POINT('Ctrl Pts',(-0.2886255007607,0.0569996518466133,
-0.831673815520566));
#75125=CARTESIAN_POINT('Ctrl Pts',(-0.285622442753231,0.072206045098832,
-0.83251471158018));
#75126=CARTESIAN_POINT('Ctrl Pts',(-0.281422252442576,0.0871423322379511,
-0.833355607639793));
#75127=CARTESIAN_POINT('Ctrl Pts',(-0.276085466300458,0.101638847384545,
-0.834196503699406));
#75128=CARTESIAN_POINT('Ctrl Pts',(-0.270385451058139,0.117122015548989,
-0.835094632316397));
#75129=CARTESIAN_POINT('Ctrl Pts',(-0.26336068465324,0.132173702975884,
-0.835992760933389));
#75130=CARTESIAN_POINT('Ctrl Pts',(-0.255098351272925,0.146555351924913,
-0.83689088955038));
#75131=CARTESIAN_POINT('Ctrl Pts',(-0.246852078845356,0.160909044729651,
-0.83778727231658));
#75132=CARTESIAN_POINT('Ctrl Pts',(-0.237373346872821,0.174594573058873,
-0.838683655082779));
#75133=CARTESIAN_POINT('Ctrl Pts',(-0.226796438815704,0.187395345034275,
-0.839580037848979));
#75134=CARTESIAN_POINT('Ctrl Pts',(-0.216221362830944,0.200193899732153,
-0.840476265348811));
#75135=CARTESIAN_POINT('Ctrl Pts',(-0.204548950046839,0.212107360231338,
-0.841372492848643));
#75136=CARTESIAN_POINT('Ctrl Pts',(-0.191955357163281,0.222950175726141,
-0.842268720348476));
#75137=CARTESIAN_POINT('Ctrl Pts',(-0.179365144260358,0.233790081129539,
-0.843164707310788));
#75138=CARTESIAN_POINT('Ctrl Pts',(-0.165854849107379,0.243559403564761,
-0.844060694273101));
#75139=CARTESIAN_POINT('Ctrl Pts',(-0.151634410991388,0.252112366621105,
-0.844956681235414));
#75140=CARTESIAN_POINT('Ctrl Pts',(-0.13737981223177,0.260685875790062,
-0.845854820556962));
#75141=CARTESIAN_POINT('Ctrl Pts',(-0.122412358134403,0.268036802464494,
-0.84675295987851));
#75142=CARTESIAN_POINT('Ctrl Pts',(-0.106967759667312,0.274064843407096,
-0.847651099200059));
#75143=CARTESIAN_POINT('Ctrl Pts',(-0.0930426383536563,0.27949983102353,
-0.84846087739117));
#75144=CARTESIAN_POINT('Ctrl Pts',(-0.0787303505568327,0.283859943650873,
-0.849270655582282));
#75145=CARTESIAN_POINT('Ctrl Pts',(-0.0642130005341933,0.287106827787839,
-0.850080433773393));
#75146=CARTESIAN_POINT('Ctrl Pts',(-0.0481117426325573,0.290707961519855,
-0.850978562390384));
#75147=CARTESIAN_POINT('Ctrl Pts',(-0.0316551246912963,0.292961927663236,
-0.851876691007376));
#75148=CARTESIAN_POINT('Ctrl Pts',(-0.0150908813271618,0.293812704457737,
-0.852774819624367));
#75149=CARTESIAN_POINT('Ctrl Pts',(0.0014411631994639,0.294661827447524,
-0.853671202390565));
#75150=CARTESIAN_POINT('Ctrl Pts',(0.0180796399818894,0.29411306901486,
-0.854567585156764));
#75151=CARTESIAN_POINT('Ctrl Pts',(0.0345697480681757,0.292161894364243,
-0.855463967922963));
#75152=CARTESIAN_POINT('Ctrl Pts',(0.0510569998309474,0.290211057685093,
-0.856360195422795));
#75153=CARTESIAN_POINT('Ctrl Pts',(0.0673951441060099,0.28685832701963,
-0.857256422922626));
#75154=CARTESIAN_POINT('Ctrl Pts',(0.0833327727470031,0.282151181082583,
-0.858152650422458));
#75155=CARTESIAN_POINT('Ctrl Pts',(0.0992661239052585,0.27744529849129,
-0.859048637384771));
#75156=CARTESIAN_POINT('Ctrl Pts',(0.114798416563009,0.27138595688038,-0.859944624347083));
#75157=CARTESIAN_POINT('Ctrl Pts',(0.129693359735733,0.264070582307946,
-0.860840611309396));
#75158=CARTESIAN_POINT('Ctrl Pts',(0.144624083862702,0.25673763458469,-0.861738750630944));
#75159=CARTESIAN_POINT('Ctrl Pts',(0.158913698638014,0.24814300168371,-0.862636889952492));
#75160=CARTESIAN_POINT('Ctrl Pts',(0.172350161151186,0.238430413226082,
-0.86353502927404));
#75161=CARTESIAN_POINT('Ctrl Pts',(0.18446471180924,0.229673372838747,-0.864344807465154));
#75162=CARTESIAN_POINT('Ctrl Pts',(0.195885772560792,0.220008408513269,
-0.865154585656267));
#75163=CARTESIAN_POINT('Ctrl Pts',(0.206482416149396,0.209567773813408,
-0.865964363847381));
#75164=CARTESIAN_POINT('Ctrl Pts',(0.218235200992725,0.197988019127006,
-0.866862492464372));
#75165=CARTESIAN_POINT('Ctrl Pts',(0.229048423692114,0.185379496124944,
-0.867760621081363));
#75166=CARTESIAN_POINT('Ctrl Pts',(0.23874073893431,0.17192003831171,-0.868658749698355));
#75167=CARTESIAN_POINT('Ctrl Pts',(0.248414213516132,0.158486744017422,
-0.869555132464553));
#75168=CARTESIAN_POINT('Ctrl Pts',(0.256970594749501,0.144206394384238,
-0.870451515230752));
#75169=CARTESIAN_POINT('Ctrl Pts',(0.264267977109875,0.129290665843496,
-0.871347897996951));
#75170=CARTESIAN_POINT('Ctrl Pts',(0.271564095458836,0.114377520921123,
-0.872244125496783));
#75171=CARTESIAN_POINT('Ctrl Pts',(0.277601253414187,0.098829901003913,
-0.873140352996615));
#75172=CARTESIAN_POINT('Ctrl Pts',(0.282283096289123,0.0828848209832521,
-0.874036580496447));
#75173=CARTESIAN_POINT('Ctrl Pts',(0.286963682609365,0.0669440204451968,
-0.874932567458759));
#75174=CARTESIAN_POINT('Ctrl Pts',(0.290289463263858,0.0506067342873947,
-0.875828554421072));
#75175=CARTESIAN_POINT('Ctrl Pts',(0.29221425225179,0.0341243429376654,
-0.876724541383384));
#75176=CARTESIAN_POINT('Ctrl Pts',(0.294143665009407,0.0176023572313884,
-0.877622680704933));
#75177=CARTESIAN_POINT('Ctrl Pts',(0.294665298255285,0.000935362784691756,
-0.878520820026481));
#75178=CARTESIAN_POINT('Ctrl Pts',(0.293785021130875,-0.0156205428564806,
-0.879418959348029));
#75179=CARTESIAN_POINT('Ctrl Pts',(0.29299134781051,-0.0305476382421383,
-0.880228737539143));
#75180=CARTESIAN_POINT('Ctrl Pts',(0.291058806445921,-0.0453839938585814,
-0.881038515730256));
#75181=CARTESIAN_POINT('Ctrl Pts',(0.288027583983001,-0.0599479012552985,
-0.88184829392137));
#75182=CARTESIAN_POINT('Ctrl Pts',(0.284665641579156,-0.0761007961489109,
-0.882746422538361));
#75183=CARTESIAN_POINT('Ctrl Pts',(0.279929909993913,-0.0920216467478163,
-0.883644551155352));
#75184=CARTESIAN_POINT('Ctrl Pts',(0.27387155637594,-0.107461670414247,
-0.884542679772343));
#75185=CARTESIAN_POINT('Ctrl Pts',(0.267824979447033,-0.122871680587019,
-0.885439062538542));
#75186=CARTESIAN_POINT('Ctrl Pts',(0.260461107918113,-0.137801966637939,
-0.886335445304741));
#75187=CARTESIAN_POINT('Ctrl Pts',(0.25188092564397,-0.152018549186396,
-0.88723182807094));
#75188=CARTESIAN_POINT('Ctrl Pts',(0.243302229580607,-0.166232669218608,
-0.888128055570772));
#75189=CARTESIAN_POINT('Ctrl Pts',(0.233508003272942,-0.179732628192698,
-0.889024283070604));
#75190=CARTESIAN_POINT('Ctrl Pts',(0.222645212152586,-0.192308994863813,
-0.889920510570435));
#75191=CARTESIAN_POINT('Ctrl Pts',(0.211785336484869,-0.204881986177619,
-0.890816497532748));
#75192=CARTESIAN_POINT('Ctrl Pts',(0.199857991045912,-0.216531285158395,
-0.89171248449506));
#75193=CARTESIAN_POINT('Ctrl Pts',(0.187049403959069,-0.227081836522777,
-0.892608471457372));
#75194=CARTESIAN_POINT('Ctrl Pts',(0.174210047807639,-0.237657732649556,
-0.89350661077892));
#75195=CARTESIAN_POINT('Ctrl Pts',(0.160485852256959,-0.247129124396079,
-0.894404750100469));
#75196=CARTESIAN_POINT('Ctrl Pts',(0.14609522201564,-0.255362146968185,
-0.895302889422017));
#75197=CARTESIAN_POINT('Ctrl Pts',(0.133120376970759,-0.262785184759634,
-0.89611266761313));
#75198=CARTESIAN_POINT('Ctrl Pts',(0.119604557020921,-0.26920194213287,
-0.896922445804244));
#75199=CARTESIAN_POINT('Ctrl Pts',(0.105722249667185,-0.27454771156451,
-0.897732223995358));
#75200=CARTESIAN_POINT('Ctrl Pts',(0.090325320432641,-0.28047672837316,
-0.898630352612349));
#75201=CARTESIAN_POINT('Ctrl Pts',(0.0743788480752792,-0.285125454735937,
-0.89952848122934));
#75202=CARTESIAN_POINT('Ctrl Pts',(0.0581196400357285,-0.288402058664839,
-0.900426609846331));
#75203=CARTESIAN_POINT('Ctrl Pts',(0.0418920378827949,-0.291672293281533,
-0.90132299261253));
#75204=CARTESIAN_POINT('Ctrl Pts',(0.0253536605572101,-0.293575480317353,
-0.902219375378729));
#75205=CARTESIAN_POINT('Ctrl Pts',(0.008755874039357,-0.294069676556096,
-0.903115758144927));
#75206=CARTESIAN_POINT('Ctrl Pts',(-0.00783903750352962,-0.294563787192954,
-0.904011985644759));
#75207=CARTESIAN_POINT('Ctrl Pts',(-0.0244925507017758,-0.2936493149825,
-0.904908213144591));
#75208=CARTESIAN_POINT('Ctrl Pts',(-0.040949009134943,-0.291336263878815,
-0.905804440644423));
#75209=CARTESIAN_POINT('Ctrl Pts',(-0.0574010508372113,-0.289023833572388,
-0.906700427606735));
#75210=CARTESIAN_POINT('Ctrl Pts',(-0.0736553602296598,-0.285313690429837,
-0.907596414569047));
#75211=CARTESIAN_POINT('Ctrl Pts',(-0.0894638911694246,-0.280267465426912,
-0.90849240153136));
#75212=CARTESIAN_POINT('Ctrl Pts',(-0.105310397703702,-0.275209118273279,
-0.909390540852908));
#75213=CARTESIAN_POINT('Ctrl Pts',(-0.120708237687313,-0.268808545723231,
-0.910288680174456));
#75214=CARTESIAN_POINT('Ctrl Pts',(-0.135426542626646,-0.261176743896147,
-0.911186819496004));
#75215=CARTESIAN_POINT('Ctrl Pts',(-0.148696824935961,-0.254295777290848,
-0.911996597687118));
#75216=CARTESIAN_POINT('Ctrl Pts',(-0.161414623626742,-0.246414802696017,
-0.912806375878232));
#75217=CARTESIAN_POINT('Ctrl Pts',(-0.173430991634858,-0.237645389478841,
-0.913616154069346));
#75218=CARTESIAN_POINT('Ctrl Pts',(-0.186644434147676,-0.228002364453471,
-0.914506602628278));
#75219=CARTESIAN_POINT('Ctrl Pts',(-0.199096911507697,-0.217220371107064,
-0.915397051187209));
#75220=CARTESIAN_POINT('Ctrl Pts',(-0.210584816913836,-0.205445065371174,
-0.916287499746141));
#75221=CARTESIAN_POINT('Ctrl Pts',(-0.222050403937057,-0.193692636371566,
-0.917176218366393));
#75222=CARTESIAN_POINT('Ctrl Pts',(-0.232554531148838,-0.180951245852864,
-0.918064936986646));
#75223=CARTESIAN_POINT('Ctrl Pts',(-0.241927388344893,-0.167406029666256,
-0.918953655606898));
#75224=CARTESIAN_POINT('Ctrl Pts',(-0.251298231000653,-0.153863724799348,
-0.919842183211814));
#75225=CARTESIAN_POINT('Ctrl Pts',(-0.259537787311925,-0.139518569562698,
-0.92073071081673));
#75226=CARTESIAN_POINT('Ctrl Pts',(-0.266517539952699,-0.124587482908844,
-0.921619238421645));
#75227=CARTESIAN_POINT('Ctrl Pts',(-0.273495931809403,-0.109659307244236,
-0.922507592797756));
#75228=CARTESIAN_POINT('Ctrl Pts',(-0.279214680733987,-0.0941461641430382,
-0.923395947173867));
#75229=CARTESIAN_POINT('Ctrl Pts',(-0.283592790252211,-0.0782864567914893,
-0.924284301549977));
#75230=CARTESIAN_POINT('Ctrl Pts',(-0.287980331297603,-0.0623925837206593,
-0.925174569660406));
#75231=CARTESIAN_POINT('Ctrl Pts',(-0.291021293038947,-0.0461514454841997,
-0.926064837770835));
#75232=CARTESIAN_POINT('Ctrl Pts',(-0.292685522236561,-0.0298131694576637,
-0.926955105881264));
#75233=CARTESIAN_POINT('Ctrl Pts',(-0.293699512991103,-0.0198584944286457,
-0.927497533351189));
#75234=CARTESIAN_POINT('Ctrl Pts',(-0.294203442548764,-0.00986790586406562,
-0.928039960821115));
#75235=CARTESIAN_POINT('Ctrl Pts',(-0.294199982280943,0.000102107260926923,
-0.92858238829104));
#75236=CARTESIAN_POINT('',(-0.294185285097018,-0.000269622437996053,-1.02858238829104));
#75237=CARTESIAN_POINT('Ctrl Pts',(-0.294640422509188,0.00010226012342875,
-0.92858238829104));
#75238=CARTESIAN_POINT('Ctrl Pts',(-0.294665749914346,0.00573321420193211,
-0.928888286908471));
#75239=CARTESIAN_POINT('Ctrl Pts',(-0.29196650606935,0.108802724357824,
-0.934488828883914));
#75240=CARTESIAN_POINT('Ctrl Pts',(-0.17133070467475,0.302651614166351,
-0.945384014217309));
#75241=CARTESIAN_POINT('Ctrl Pts',(0.161491629393738,0.308014063895984,
-0.961267944291316));
#75242=CARTESIAN_POINT('Ctrl Pts',(0.346377967474509,0.0312171999089644,
-0.977151874365297));
#75243=CARTESIAN_POINT('Ctrl Pts',(0.213961360511507,-0.274176487193874,
-0.993035804439286));
#75244=CARTESIAN_POINT('Ctrl Pts',(-0.114456655868126,-0.32840810563904,
-1.00891973451328));
#75245=CARTESIAN_POINT('Ctrl Pts',(-0.281231284280514,-0.144445699392593,
-1.0207685957972));
#75246=CARTESIAN_POINT('Ctrl Pts',(-0.294398628936313,-0.0235490913753662,
-1.02732281372311));
#75247=CARTESIAN_POINT('Ctrl Pts',(-0.294185285097018,-0.000269622437996053,
-1.02858238829104));
#75248=CARTESIAN_POINT('',(-0.294156470823094,5.4011646819036E-5,-1.12858239090245));
#75249=CARTESIAN_POINT('Ctrl Pts',(-0.294185285097018,-0.000269622437996053,
-1.02858238829104));
#75250=CARTESIAN_POINT('Ctrl Pts',(-0.293501834438824,0.0743065566550019,
-1.03261745708111));
#75251=CARTESIAN_POINT('Ctrl Pts',(-0.226814830045291,0.247826008594651,
-1.04194716922918));
#75252=CARTESIAN_POINT('Ctrl Pts',(0.0649346204485502,0.341666072341295,
-1.05657152473523));
#75253=CARTESIAN_POINT('Ctrl Pts',(0.322328030805379,0.130601877777676,
-1.07245545480923));
#75254=CARTESIAN_POINT('Ctrl Pts',(0.284449677226377,-0.20010145188811,
-1.08833938488322));
#75255=CARTESIAN_POINT('Ctrl Pts',(-0.0140016018153781,-0.347499877796429,
-1.10422331495721));
#75256=CARTESIAN_POINT('Ctrl Pts',(-0.25521828530379,-0.203143761611344,
-1.11763764942648));
#75257=CARTESIAN_POINT('Ctrl Pts',(-0.293639961408326,-0.0523650648297256,
-1.12575734053776));
#75258=CARTESIAN_POINT('Ctrl Pts',(-0.293725670975061,5.38840834055088E-5,
-1.12858238829104));
#75259=CARTESIAN_POINT('',(-0.294199899345979,0.000243361492577376,-1.22858238829104));
#75260=CARTESIAN_POINT('Ctrl Pts',(-0.294199995039683,5.40245347011106E-5,
-1.12858239116628));
#75261=CARTESIAN_POINT('Ctrl Pts',(-0.294196741129914,0.0177737558262076,
-1.1295358325691));
#75262=CARTESIAN_POINT('Ctrl Pts',(-0.292588338013046,0.0354528612017167,
-1.13048927397193));
#75263=CARTESIAN_POINT('Ctrl Pts',(-0.289421898081706,0.0528072429765333,
-1.13144271537476));
#75264=CARTESIAN_POINT('Ctrl Pts',(-0.286238793401952,0.0702529596297707,
-1.13240117467196));
#75265=CARTESIAN_POINT('Ctrl Pts',(-0.281481430394538,0.0873699267563183,
-1.13335963396916));
#75266=CARTESIAN_POINT('Ctrl Pts',(-0.275247570906157,0.103886547301661,
-1.13431809326636));
#75267=CARTESIAN_POINT('Ctrl Pts',(-0.271620306077327,0.113496991185887,
-1.13487578721264));
#75268=CARTESIAN_POINT('Ctrl Pts',(-0.267494065615411,0.122904544285773,
-1.13543348115891));
#75269=CARTESIAN_POINT('Ctrl Pts',(-0.262895278083352,0.132059504623776,
-1.13599117510519));
#75270=CARTESIAN_POINT('Ctrl Pts',(-0.255489239854686,0.146802952928902,
-1.13688930372218));
#75271=CARTESIAN_POINT('Ctrl Pts',(-0.246815415719676,0.160968594895102,
-1.13778743233917));
#75272=CARTESIAN_POINT('Ctrl Pts',(-0.236987279564667,0.174329198141156,
-1.13868556095616));
#75273=CARTESIAN_POINT('Ctrl Pts',(-0.227178248089065,0.187663830029297,
-1.13958194372236));
#75274=CARTESIAN_POINT('Ctrl Pts',(-0.216219768717126,0.200195860004963,
-1.14047832648855));
#75275=CARTESIAN_POINT('Ctrl Pts',(-0.204269643802464,0.211725181829688,
-1.14137470925475));
#75276=CARTESIAN_POINT('Ctrl Pts',(-0.192321588821037,0.223252506610316,
-1.14227093675458));
#75277=CARTESIAN_POINT('Ctrl Pts',(-0.179382760267418,0.23377688198026,
-1.14316716425441));
#75278=CARTESIAN_POINT('Ctrl Pts',(-0.165649074942735,0.243133757365398,
-1.14406339175424));
#75279=CARTESIAN_POINT('Ctrl Pts',(-0.151919075586849,0.252488121468976,
-1.14495937871655));
#75280=CARTESIAN_POINT('Ctrl Pts',(-0.137395303356355,0.260675170764054,
-1.14585536567886));
#75281=CARTESIAN_POINT('Ctrl Pts',(-0.122302767525096,0.267573677808006,
-1.14675135264117));
#75282=CARTESIAN_POINT('Ctrl Pts',(-0.10717397607824,0.274488756594597,
-1.14764949196272));
#75283=CARTESIAN_POINT('Ctrl Pts',(-0.0914744261301407,0.280108804330703,
-1.14854763128427));
#75284=CARTESIAN_POINT('Ctrl Pts',(-0.0754496181504297,0.284360677873989,
-1.14944577060581));
#75285=CARTESIAN_POINT('Ctrl Pts',(-0.0610013697467702,0.288194241758942,
-1.15025554879693));
#75286=CARTESIAN_POINT('Ctrl Pts',(-0.0462893626626646,0.290916191733231,
-1.15106532698805));
#75287=CARTESIAN_POINT('Ctrl Pts',(-0.0314988602969082,0.292508908924149,
-1.15187510517916));
#75288=CARTESIAN_POINT('Ctrl Pts',(-0.0150946479087731,0.294275398690888,
-1.15277323379615));
#75289=CARTESIAN_POINT('Ctrl Pts',(0.00151107934364759,0.294663290245999,
-1.15367136241314));
#75290=CARTESIAN_POINT('Ctrl Pts',(0.0180658564198836,0.293644793639894,
-1.15456949103014));
#75291=CARTESIAN_POINT('Ctrl Pts',(0.0345884530599,0.292628276865045,-1.15546587379634));
#75292=CARTESIAN_POINT('Ctrl Pts',(0.0510595112019997,0.290210780404567,
-1.15636225656253));
#75293=CARTESIAN_POINT('Ctrl Pts',(0.067225337852934,0.286416469412216,
-1.15725863932873));
#75294=CARTESIAN_POINT('Ctrl Pts',(0.0833883643505557,0.282622815649015,
-1.15815486682857));
#75295=CARTESIAN_POINT('Ctrl Pts',(0.0992454840209208,0.277452949400478,
-1.1590510943284));
#75296=CARTESIAN_POINT('Ctrl Pts',(0.114552227882036,0.27098233722378,-1.15994732182823));
#75297=CARTESIAN_POINT('Ctrl Pts',(0.12985486358289,0.264513461687614,-1.16084330879055));
#75298=CARTESIAN_POINT('Ctrl Pts',(0.144606691656802,0.256744851487481,
-1.16173929575286));
#75299=CARTESIAN_POINT('Ctrl Pts',(0.158583884535607,0.247799902271162,
-1.16263528271517));
#75300=CARTESIAN_POINT('Ctrl Pts',(0.172594653729077,0.238833465304609,
-1.16353342203672));
#75301=CARTESIAN_POINT('Ctrl Pts',(0.185826415731223,0.228685496076821,
-1.16443156135827));
#75302=CARTESIAN_POINT('Ctrl Pts',(0.198084647298157,0.217522671243171,
-1.16532970067982));
#75303=CARTESIAN_POINT('Ctrl Pts',(0.20913688423552,0.207458072261,-1.16613947887093));
#75304=CARTESIAN_POINT('Ctrl Pts',(0.219397872621403,0.196569349588083,
-1.16694925706205));
#75305=CARTESIAN_POINT('Ctrl Pts',(0.228752398375091,0.18500264927196,-1.16775903525316));
#75306=CARTESIAN_POINT('Ctrl Pts',(0.239127544766995,0.17217397016936,-1.16865716387015));
#75307=CARTESIAN_POINT('Ctrl Pts',(0.248453335307034,0.158428779437926,
-1.16955529248714));
#75308=CARTESIAN_POINT('Ctrl Pts',(0.256569586884884,0.143964186816444,
-1.17045342110413));
#75309=CARTESIAN_POINT('Ctrl Pts',(0.264670061474919,0.129527711571482,
-1.17134980387033));
#75310=CARTESIAN_POINT('Ctrl Pts',(0.271565223520873,0.1143752600927,-1.17224618663653));
#75311=CARTESIAN_POINT('Ctrl Pts',(0.277137887352363,0.0987331321992221,
-1.17314256940273));
#75312=CARTESIAN_POINT('Ctrl Pts',(0.282709585918454,0.0830937137469134,
-1.17403879690256));
#75313=CARTESIAN_POINT('Ctrl Pts',(0.286958926216699,0.0669655127220728,
-1.17493502440239));
#75314=CARTESIAN_POINT('Ctrl Pts',(0.289816835300472,0.0505948809309715,
-1.17583125190223));
#75315=CARTESIAN_POINT('Ctrl Pts',(0.292673977353148,0.0342286428358504,
-1.17672723886454));
#75316=CARTESIAN_POINT('Ctrl Pts',(0.29414030402327,0.0176208849480362,
-1.17762322582685));
#75317=CARTESIAN_POINT('Ctrl Pts',(0.294198208894361,0.00102658820850397,
-1.17851921278916));
#75318=CARTESIAN_POINT('Ctrl Pts',(0.294256252865784,-0.01560757170912,
-1.17941735211071));
#75319=CARTESIAN_POINT('Ctrl Pts',(0.292899141155415,-0.0322274108459776,
-1.18031549143226));
#75320=CARTESIAN_POINT('Ctrl Pts',(0.290161522676543,-0.048579118539039,
-1.18121363075381));
#75321=CARTESIAN_POINT('Ctrl Pts',(0.287693237760616,-0.0633221054672461,
-1.18202340894492));
#75322=CARTESIAN_POINT('Ctrl Pts',(0.284103528081797,-0.0778467792510078,
-1.18283318713603));
#75323=CARTESIAN_POINT('Ctrl Pts',(0.27945277186965,-0.0919771074472861,
-1.18364296532715));
#75324=CARTESIAN_POINT('Ctrl Pts',(0.274294597334179,-0.107649117708652,
-1.18454109394414));
#75325=CARTESIAN_POINT('Ctrl Pts',(0.267797468983183,-0.122935973521103,
-1.18543922256113));
#75326=CARTESIAN_POINT('Ctrl Pts',(0.260040222950703,-0.137596229773017,
-1.18633735117812));
#75327=CARTESIAN_POINT('Ctrl Pts',(0.252298056043723,-0.152227988302547,
-1.18723373394432));
#75328=CARTESIAN_POINT('Ctrl Pts',(0.243300940961319,-0.166234842540761,
-1.18813011671052));
#75329=CARTESIAN_POINT('Ctrl Pts',(0.233175548442287,-0.179395662178991,
-1.18902649947671));
#75330=CARTESIAN_POINT('Ctrl Pts',(0.223051909786638,-0.192554202174274,
-1.18992272697655));
#75331=CARTESIAN_POINT('Ctrl Pts',(0.211800820724213,-0.204866340744693,
-1.19081895447638));
#75332=CARTESIAN_POINT('Ctrl Pts',(0.199591879296107,-0.216140513830814,
-1.19171518197621));
#75333=CARTESIAN_POINT('Ctrl Pts',(0.187386214612451,-0.227411661053939,
-1.19261116893852));
#75334=CARTESIAN_POINT('Ctrl Pts',(0.174223796905752,-0.237644866616127,
-1.19350715590083));
#75335=CARTESIAN_POINT('Ctrl Pts',(0.160309369442262,-0.246687142082891,
-1.19440314286315));
#75336=CARTESIAN_POINT('Ctrl Pts',(0.146361516440544,-0.255751139099109,
-1.19530128218469));
#75337=CARTESIAN_POINT('Ctrl Pts',(0.131658726552284,-0.263618080984681,
-1.19619942150624));
#75338=CARTESIAN_POINT('Ctrl Pts',(0.116433080370029,-0.270179528823977,
-1.19709756082779));
#75339=CARTESIAN_POINT('Ctrl Pts',(0.102705370282942,-0.276095445469563,
-1.19790733901891));
#75340=CARTESIAN_POINT('Ctrl Pts',(0.0885533514090525,-0.280950600039411,
-1.19871711721002));
#75341=CARTESIAN_POINT('Ctrl Pts',(0.0741576842169672,-0.284700329946378,
-1.19952689540113));
#75342=CARTESIAN_POINT('Ctrl Pts',(0.0581913852875117,-0.288859172173035,
-1.20042502401813));
#75343=CARTESIAN_POINT('Ctrl Pts',(0.0418230963952611,-0.291684018395409,
-1.20132315263512));
#75344=CARTESIAN_POINT('Ctrl Pts',(0.0252984543023825,-0.293110266299068,
-1.20222128125211));
#75345=CARTESIAN_POINT('Ctrl Pts',(0.00880593406704758,-0.294533741753452,
-1.20311766401831));
#75346=CARTESIAN_POINT('Ctrl Pts',(-0.00784156235179397,-0.294563882115743,
-1.2040140467845));
#75347=CARTESIAN_POINT('Ctrl Pts',(-0.024389545782722,-0.29318729518264,
-1.2049104295507));
#75348=CARTESIAN_POINT('Ctrl Pts',(-0.0409346628652968,-0.291810946694161,
-1.20580665705053));
#75349=CARTESIAN_POINT('Ctrl Pts',(-0.0573795104557058,-0.289028367136229,
-1.20670288455037));
#75350=CARTESIAN_POINT('Ctrl Pts',(-0.0734711814793199,-0.284878264337652,
-1.2075991120502));
#75351=CARTESIAN_POINT('Ctrl Pts',(-0.0895585336769281,-0.280729275380631,
-1.20849509901251));
#75352=CARTESIAN_POINT('Ctrl Pts',(-0.105292133518021,-0.275213699979629,
-1.20939108597482));
#75353=CARTESIAN_POINT('Ctrl Pts',(-0.120432445137094,-0.26842068876728,
-1.21028707293713));
#75354=CARTESIAN_POINT('Ctrl Pts',(-0.135609127139796,-0.261611359236656,
-1.21118521225868));
#75355=CARTESIAN_POINT('Ctrl Pts',(-0.150188959871209,-0.253518814355502,
-1.21208335158023));
#75356=CARTESIAN_POINT('Ctrl Pts',(-0.163955030769725,-0.24427932349116,
-1.21298149090178));
#75357=CARTESIAN_POINT('Ctrl Pts',(-0.17636676213866,-0.235948836205473,
-1.21379126909289));
#75358=CARTESIAN_POINT('Ctrl Pts',(-0.18811699407947,-0.226686859448853,
-1.214601047284));
#75359=CARTESIAN_POINT('Ctrl Pts',(-0.199070279684257,-0.216621014092428,
-1.21541082547512));
#75360=CARTESIAN_POINT('Ctrl Pts',(-0.211037652827153,-0.205623243037651,
-1.21629557532331));
#75361=CARTESIAN_POINT('Ctrl Pts',(-0.222134545065787,-0.193590312477439,
-1.2171803251715));
#75362=CARTESIAN_POINT('Ctrl Pts',(-0.232176184747201,-0.180687186142885,
-1.21806507501969));
#75363=CARTESIAN_POINT('Ctrl Pts',(-0.242203172990491,-0.167802886350917,
-1.21894853395743));
#75364=CARTESIAN_POINT('Ctrl Pts',(-0.251177400380996,-0.154051495304126,
-1.21983199289516));
#75365=CARTESIAN_POINT('Ctrl Pts',(-0.258951788135257,-0.139633847693004,
-1.2207154518329));
#75366=CARTESIAN_POINT('Ctrl Pts',(-0.266718384557415,-0.125230649152887,
-1.22159802538619));
#75367=CARTESIAN_POINT('Ctrl Pts',(-0.273287117552961,-0.110163223906686,
-1.22248059893948));
#75368=CARTESIAN_POINT('Ctrl Pts',(-0.278555812509406,-0.0946588575740512,
-1.22336317249277));
#75369=CARTESIAN_POINT('Ctrl Pts',(-0.283832396389795,-0.0791312762388782,
-1.22424706754137));
#75370=CARTESIAN_POINT('Ctrl Pts',(-0.287804785773448,-0.0631662223080026,
-1.22513096258996));
#75371=CARTESIAN_POINT('Ctrl Pts',(-0.290420181564497,-0.0470080646277298,
-1.22601485763856));
#75372=CARTESIAN_POINT('Ctrl Pts',(-0.292952574549606,-0.0313627059780524,
-1.22687070118938));
#75373=CARTESIAN_POINT('Ctrl Pts',(-0.294212952872461,-0.0155370569154584,
-1.22772654474021));
#75374=CARTESIAN_POINT('Ctrl Pts',(-0.294199899345979,0.000243361492577376,
-1.22858238829104));
#75375=CARTESIAN_POINT('',(-0.294199932671572,-0.000199037792005543,-1.32858238829104));
#75376=CARTESIAN_POINT('Ctrl Pts',(-0.294383220786406,0.000243513135659165,
-1.22858238829104));
#75377=CARTESIAN_POINT('Ctrl Pts',(-0.294531804372818,0.0169246405636604,
-1.2294865107104));
#75378=CARTESIAN_POINT('Ctrl Pts',(-0.285648723188225,0.131134112473027,
-1.23568527648771));
#75379=CARTESIAN_POINT('Ctrl Pts',(-0.136187107091055,0.320008252681217,
-1.24717868562313));
#75380=CARTESIAN_POINT('Ctrl Pts',(0.195124888317045,0.287886241215498,
-1.26306261569707));
#75381=CARTESIAN_POINT('Ctrl Pts',(0.347690809990289,-0.00795679396688126,
-1.27894654577109));
#75382=CARTESIAN_POINT('Ctrl Pts',(0.181751144316383,-0.296510929750662,
-1.29483047584506));
#75383=CARTESIAN_POINT('Ctrl Pts',(-0.150683445319157,-0.313443311028766,
-1.31071440591904));
#75384=CARTESIAN_POINT('Ctrl Pts',(-0.288377247002049,-0.122059486604382,
-1.32196504340104));
#75385=CARTESIAN_POINT('Ctrl Pts',(-0.294601083516667,-0.0123879459390851,
-1.32792103752504));
#75386=CARTESIAN_POINT('Ctrl Pts',(-0.294506364479898,-0.000199245105141105,
-1.32858238829104));
#75387=CARTESIAN_POINT('',(-0.294199973927967,-0.00012385791773357,-1.42858238828812));
#75388=CARTESIAN_POINT('Ctrl Pts',(-0.294199932671572,-0.000199037792005543,
-1.32858238829104));
#75389=CARTESIAN_POINT('Ctrl Pts',(-0.29421095546823,0.0160938782514552,
-1.32946735688903));
#75390=CARTESIAN_POINT('Ctrl Pts',(-0.292864222061912,0.0324398188035349,
-1.33035232548702));
#75391=CARTESIAN_POINT('Ctrl Pts',(-0.290159642085904,0.0485903499120993,
-1.33123729408502));
#75392=CARTESIAN_POINT('Ctrl Pts',(-0.287459443285101,0.0647147186194478,
-1.33212082911384));
#75393=CARTESIAN_POINT('Ctrl Pts',(-0.283405838901624,0.0806434996177015,
-1.33300436414265));
#75394=CARTESIAN_POINT('Ctrl Pts',(-0.278050516457775,0.0961329823607096,
-1.33388789917147));
#75395=CARTESIAN_POINT('Ctrl Pts',(-0.272694507482042,0.111624450796248,
-1.33477154746611));
#75396=CARTESIAN_POINT('Ctrl Pts',(-0.266036680896201,0.126675727872778,
-1.33565519576074));
#75397=CARTESIAN_POINT('Ctrl Pts',(-0.258178495635449,0.14105851406922,
-1.33653884405538));
#75398=CARTESIAN_POINT('Ctrl Pts',(-0.250319312112871,0.155443127377896,
-1.33742260460397));
#75399=CARTESIAN_POINT('Ctrl Pts',(-0.241259888122196,0.169158383239423,
-1.33830636515255));
#75400=CARTESIAN_POINT('Ctrl Pts',(-0.231146528751372,0.182002533625747,
-1.33919012570114));
#75401=CARTESIAN_POINT('Ctrl Pts',(-0.221011611213856,0.194874063275963,
-1.34007577012002));
#75402=CARTESIAN_POINT('Ctrl Pts',(-0.209818833944237,0.206870188509988,
-1.34096141453889));
#75403=CARTESIAN_POINT('Ctrl Pts',(-0.197752936199888,0.217824278317002,
-1.34184705895777));
#75404=CARTESIAN_POINT('Ctrl Pts',(-0.19486827810482,0.220443130598484,
-1.34205879466085));
#75405=CARTESIAN_POINT('Ctrl Pts',(-0.191933860052037,0.22300260765447,
-1.34227053036394));
#75406=CARTESIAN_POINT('Ctrl Pts',(-0.188952462317281,0.225500791537938,
-1.34248226606702));
#75407=CARTESIAN_POINT('Ctrl Pts',(-0.176306136803009,0.236097447668901,
-1.34338039468402));
#75408=CARTESIAN_POINT('Ctrl Pts',(-0.162725190941781,0.245660843872892,
-1.34427852330101));
#75409=CARTESIAN_POINT('Ctrl Pts',(-0.148403919238009,0.254027393709416,
-1.345176651918));
#75410=CARTESIAN_POINT('Ctrl Pts',(-0.134110486312648,0.262377680009309,
-1.3460730346842));
#75411=CARTESIAN_POINT('Ctrl Pts',(-0.119080226176381,0.269535286151918,
-1.3469694174504));
#75412=CARTESIAN_POINT('Ctrl Pts',(-0.103537366684782,0.275379109047838,
-1.34786580021659));
#75413=CARTESIAN_POINT('Ctrl Pts',(-0.0879971994396348,0.281221919709718,
-1.34876202771643));
#75414=CARTESIAN_POINT('Ctrl Pts',(-0.0719453289797071,0.285751071507304,
-1.34965825521626));
#75415=CARTESIAN_POINT('Ctrl Pts',(-0.0556268687501311,0.288893218115372,
-1.35055448271609));
#75416=CARTESIAN_POINT('Ctrl Pts',(-0.039312788214266,0.292034521406144,
-1.3514504696784));
#75417=CARTESIAN_POINT('Ctrl Pts',(-0.0227330394533085,0.29378941940524,
-1.35234645664072));
#75418=CARTESIAN_POINT('Ctrl Pts',(-0.00614225869613748,0.294135874483392,
-1.35324244360303));
#75419=CARTESIAN_POINT('Ctrl Pts',(0.0104883767929551,0.294483161823417,
-1.35414058292458));
#75420=CARTESIAN_POINT('Ctrl Pts',(0.0271293018715402,0.293415258429718,
-1.35503872224613));
#75421=CARTESIAN_POINT('Ctrl Pts',(0.0435261417414881,0.290962394451757,
-1.35593686156767));
#75422=CARTESIAN_POINT('Ctrl Pts',(0.0583098206332988,0.288750849196508,
-1.35674663975879));
#75423=CARTESIAN_POINT('Ctrl Pts',(0.072894719894761,0.285414252481799,
-1.3575564179499));
#75424=CARTESIAN_POINT('Ctrl Pts',(0.0871037837793806,0.281009912371993,
-1.35836619614102));
#75425=CARTESIAN_POINT('Ctrl Pts',(0.102863120145144,0.276125039038795,
-1.35926432475801));
#75426=CARTESIAN_POINT('Ctrl Pts',(0.118260643424989,0.269894716873243,
-1.360162453375));
#75427=CARTESIAN_POINT('Ctrl Pts',(0.133053574128968,0.262393571589525,
-1.36106058199199));
#75428=CARTESIAN_POINT('Ctrl Pts',(0.147817749207858,0.254907007603174,
-1.36195696475819));
#75429=CARTESIAN_POINT('Ctrl Pts',(0.161978936831009,0.246154818702195,
-1.36285334752439));
#75430=CARTESIAN_POINT('Ctrl Pts',(0.175313837441747,0.236259811227912,
-1.36374973029059));
#75431=CARTESIAN_POINT('Ctrl Pts',(0.188646428256217,0.226366517711012,
-1.36464595779042));
#75432=CARTESIAN_POINT('Ctrl Pts',(0.201152350907598,0.215331226146877,
-1.36554218529025));
#75433=CARTESIAN_POINT('Ctrl Pts',(0.212637121153248,0.203320177817301,
-1.36643841279008));
#75434=CARTESIAN_POINT('Ctrl Pts',(0.224118809013962,0.191312353119861,
-1.36733439975239));
#75435=CARTESIAN_POINT('Ctrl Pts',(0.234579349172184,0.178329871247663,
-1.36823038671471));
#75436=CARTESIAN_POINT('Ctrl Pts',(0.243862216035669,0.164574784186924,
-1.36912637367702));
#75437=CARTESIAN_POINT('Ctrl Pts',(0.253167382402457,0.150786654358918,
-1.37002451299857));
#75438=CARTESIAN_POINT('Ctrl Pts',(0.261288802265385,0.136222886146696,
-1.37092265232011));
#75439=CARTESIAN_POINT('Ctrl Pts',(0.26811401744516,0.121113639402903,-1.37182079164166));
#75440=CARTESIAN_POINT('Ctrl Pts',(0.274267751358872,0.10749087709448,-1.37263056983277));
#75441=CARTESIAN_POINT('Ctrl Pts',(0.27936826190931,0.0934254245163044,
-1.37344034802389));
#75442=CARTESIAN_POINT('Ctrl Pts',(0.283367751749445,0.0790971381812571,
-1.374250126215));
#75443=CARTESIAN_POINT('Ctrl Pts',(0.28780360383611,0.0632055716619879,
-1.37514825483199));
#75444=CARTESIAN_POINT('Ctrl Pts',(0.290912651841137,0.0468888790454422,
-1.37604638344899));
#75445=CARTESIAN_POINT('Ctrl Pts',(0.292626031829465,0.0303915365807849,
-1.37694451206598));
#75446=CARTESIAN_POINT('Ctrl Pts',(0.294336081219308,0.0139262629065766,
-1.37784089483218));
#75447=CARTESIAN_POINT('Ctrl Pts',(0.294655701078259,-0.00271819228434685,
-1.37873727759837));
#75448=CARTESIAN_POINT('Ctrl Pts',(0.293567075904432,-0.0192876111771652,
-1.37963366036457));
#75449=CARTESIAN_POINT('Ctrl Pts',(0.292478639296118,-0.035854160008702,
-1.38052988786441));
#75450=CARTESIAN_POINT('Ctrl Pts',(0.289982440651052,-0.0523449075233701,
-1.38142611536424));
#75451=CARTESIAN_POINT('Ctrl Pts',(0.286112784133044,-0.0685063117941561,
-1.38232234286407));
#75452=CARTESIAN_POINT('Ctrl Pts',(0.282244166187922,-0.0846633785233022,
-1.38321832982638));
#75453=CARTESIAN_POINT('Ctrl Pts',(0.277003017012444,-0.100490510015907,
-1.38411431678869));
#75454=CARTESIAN_POINT('Ctrl Pts',(0.270474308459799,-0.11574665638019,
-1.38501030375101));
#75455=CARTESIAN_POINT('Ctrl Pts',(0.263929916502435,-0.13103945138883,
-1.38590844307255));
#75456=CARTESIAN_POINT('Ctrl Pts',(0.256092124579347,-0.145757801258977,
-1.3868065823941));
#75457=CARTESIAN_POINT('Ctrl Pts',(0.247093409551672,-0.159682456632311,
-1.38770472171565));
#75458=CARTESIAN_POINT('Ctrl Pts',(0.238980009990367,-0.172237170549782,
-1.38851449990676));
#75459=CARTESIAN_POINT('Ctrl Pts',(0.229923758957237,-0.184146682770158,
-1.38932427809787));
#75460=CARTESIAN_POINT('Ctrl Pts',(0.22004990273473,-0.195273347660237,
-1.39013405628899));
#75461=CARTESIAN_POINT('Ctrl Pts',(0.2090987645949,-0.207613981501867,-1.39103218490598));
#75462=CARTESIAN_POINT('Ctrl Pts',(0.197071263310841,-0.219069977761558,
-1.39193031352297));
#75463=CARTESIAN_POINT('Ctrl Pts',(0.184135533987629,-0.22945096452857,
-1.39282844213996));
#75464=CARTESIAN_POINT('Ctrl Pts',(0.17122495012004,-0.239811771943064,
-1.39372482490616));
#75465=CARTESIAN_POINT('Ctrl Pts',(0.157410211298321,-0.249101176485043,
-1.39462120767236));
#75466=CARTESIAN_POINT('Ctrl Pts',(0.142895306141158,-0.257166427596653,
-1.39551759043856));
#75467=CARTESIAN_POINT('Ctrl Pts',(0.128382915174002,-0.265230281690954,
-1.39641381793839));
#75468=CARTESIAN_POINT('Ctrl Pts',(0.113171262560871,-0.272069973646394,
-1.39731004543822));
#75469=CARTESIAN_POINT('Ctrl Pts',(0.0974920162052542,-0.277576920467525,
-1.39820627293805));
#75470=CARTESIAN_POINT('Ctrl Pts',(0.081816977985442,-0.283082389285213,
-1.39910225990037));
#75471=CARTESIAN_POINT('Ctrl Pts',(0.0656753457450195,-0.287255570874658,
-1.39999824686268));
#75472=CARTESIAN_POINT('Ctrl Pts',(0.0493157494804751,-0.290037233563519,
-1.40089423382499));
#75473=CARTESIAN_POINT('Ctrl Pts',(0.0329168538403857,-0.29282557842258,
-1.40179237314654));
#75474=CARTESIAN_POINT('Ctrl Pts',(0.016299736536797,-0.294215620741398,
-1.40269051246809));
#75475=CARTESIAN_POINT('Ctrl Pts',(-0.00027954726078042,-0.294199867187817,
-1.40358865178963));
#75476=CARTESIAN_POINT('Ctrl Pts',(-0.0152277208029774,-0.294185663507144,
-1.40439842998075));
#75477=CARTESIAN_POINT('Ctrl Pts',(-0.0301446655582793,-0.293029409525153,
-1.40520820817186));
#75478=CARTESIAN_POINT('Ctrl Pts',(-0.0448468247040668,-0.290761762124876,
-1.40601798636298));
#75479=CARTESIAN_POINT('Ctrl Pts',(-0.0611530552314759,-0.288246704241395,
-1.40691611497997));
#75480=CARTESIAN_POINT('Ctrl Pts',(-0.07729919491733,-0.284347626057459,
-1.40781424359696));
#75481=CARTESIAN_POINT('Ctrl Pts',(-0.0930341314336671,-0.279102652062611,
-1.40871237221395));
#75482=CARTESIAN_POINT('Ctrl Pts',(-0.108738481182302,-0.273867873647582,
-1.40960875498015));
#75483=CARTESIAN_POINT('Ctrl Pts',(-0.124032451266787,-0.267292577113482,
-1.41050513774635));
#75484=CARTESIAN_POINT('Ctrl Pts',(-0.138677114729015,-0.259465407810821,
-1.41140152051254));
#75485=CARTESIAN_POINT('Ctrl Pts',(-0.153319241525229,-0.251639594286284,
-1.41229774801237));
#75486=CARTESIAN_POINT('Ctrl Pts',(-0.167311564065965,-0.242562663572469,
-1.41319397551221));
#75487=CARTESIAN_POINT('Ctrl Pts',(-0.180437272370374,-0.232370460126797,
-1.41409020301204));
#75488=CARTESIAN_POINT('Ctrl Pts',(-0.193559457880269,-0.222180992155474,
-1.41498618997435));
#75489=CARTESIAN_POINT('Ctrl Pts',(-0.205814872157734,-0.210877339787728,
-1.41588217693666));
#75490=CARTESIAN_POINT('Ctrl Pts',(-0.217018987017479,-0.198636349326873,
-1.41677816389897));
#75491=CARTESIAN_POINT('Ctrl Pts',(-0.228250016643971,-0.186365953294303,
-1.41767630322052));
#75492=CARTESIAN_POINT('Ctrl Pts',(-0.238424185529855,-0.173154326119332,
-1.41857444254206));
#75493=CARTESIAN_POINT('Ctrl Pts',(-0.24739642205455,-0.159212594836611,
-1.41947258186361));
#75494=CARTESIAN_POINT('Ctrl Pts',(-0.255485948132456,-0.146642484979129,
-1.42028236005473));
#75495=CARTESIAN_POINT('Ctrl Pts',(-0.26259877260222,-0.133479662631015,
-1.42109213824585));
#75496=CARTESIAN_POINT('Ctrl Pts',(-0.26866117713439,-0.119895003652211,
-1.42190191643696));
#75497=CARTESIAN_POINT('Ctrl Pts',(-0.276031327328041,-0.103379943254638,
-1.4228863751382));
#75498=CARTESIAN_POINT('Ctrl Pts',(-0.281889563048866,-0.0861502897819955,
-1.42387083383943));
#75499=CARTESIAN_POINT('Ctrl Pts',(-0.286117995118731,-0.0684845447472487,
-1.42485529254066));
#75500=CARTESIAN_POINT('Ctrl Pts',(-0.290318258654323,-0.0509364835575405,
-1.42583319307607));
#75501=CARTESIAN_POINT('Ctrl Pts',(-0.292910121610845,-0.0329586072094055,
-1.42681109361149));
#75502=CARTESIAN_POINT('Ctrl Pts',(-0.293825270581318,-0.0148442031721232,
-1.4277889941469));
#75503=CARTESIAN_POINT('Ctrl Pts',(-0.294072764678868,-0.00994531979409522,
-1.42805345886064));
#75504=CARTESIAN_POINT('Ctrl Pts',(-0.294197905692056,-0.00503654304993215,
-1.42831792357438));
#75505=CARTESIAN_POINT('Ctrl Pts',(-0.294199973927967,-0.000123857917735108,
-1.42858238828812));
#75506=CARTESIAN_POINT('',(-0.294199884656848,0.000260514677417675,-1.52858238829104));
#75507=CARTESIAN_POINT('Ctrl Pts',(-0.294199973927989,-0.000123857863553138,
-1.42858238829104));
#75508=CARTESIAN_POINT('Ctrl Pts',(-0.29420711687311,0.0168428022082966,
-1.42949575496899));
#75509=CARTESIAN_POINT('Ctrl Pts',(-0.292742206137062,0.0338023587179249,
-1.43040912164694));
#75510=CARTESIAN_POINT('Ctrl Pts',(-0.289834972294292,0.050490878732371,
-1.43132248832489));
#75511=CARTESIAN_POINT('Ctrl Pts',(-0.286925430138747,0.0671926492543543,
-1.43223658020628));
#75512=CARTESIAN_POINT('Ctrl Pts',(-0.282571464413671,0.0836222276575034,
-1.43315067208766));
#75513=CARTESIAN_POINT('Ctrl Pts',(-0.276853623498289,0.0995274392108404,
-1.43406476396905));
#75514=CARTESIAN_POINT('Ctrl Pts',(-0.271119421515831,0.115478162039664,
-1.43498147143887));
#75515=CARTESIAN_POINT('Ctrl Pts',(-0.264013865578162,0.130900841221588,
-1.4358981789087));
#75516=CARTESIAN_POINT('Ctrl Pts',(-0.255665255464979,0.14556413414034,
-1.43681488637852));
#75517=CARTESIAN_POINT('Ctrl Pts',(-0.252717689366375,0.150741166546365,
-1.437138539756));
#75518=CARTESIAN_POINT('Ctrl Pts',(-0.249615575581539,0.155823795936581,
-1.43746219313348));
#75519=CARTESIAN_POINT('Ctrl Pts',(-0.246365814950903,0.160802752537317,
-1.43778584651096));
#75520=CARTESIAN_POINT('Ctrl Pts',(-0.2373478246445,0.174619210875247,-1.43868397512795));
#75521=CARTESIAN_POINT('Ctrl Pts',(-0.227135117003751,0.187718876523039,
-1.43958210374494));
#75522=CARTESIAN_POINT('Ctrl Pts',(-0.215866014277897,0.199888728746207,
-1.44048023236193));
#75523=CARTESIAN_POINT('Ctrl Pts',(-0.20461881729199,0.21203492428397,-1.44137661512813));
#75524=CARTESIAN_POINT('Ctrl Pts',(-0.19231978425414,0.22325427505796,-1.44227299789432));
#75525=CARTESIAN_POINT('Ctrl Pts',(-0.179148232018249,0.233365702203078,
-1.44316938066052));
#75526=CARTESIAN_POINT('Ctrl Pts',(-0.165978961284344,0.243475377903818,
-1.44406560816035));
#75527=CARTESIAN_POINT('Ctrl Pts',(-0.151938064932521,0.252476988365536,
-1.44496183566018));
#75528=CARTESIAN_POINT('Ctrl Pts',(-0.137238731345518,0.260229073353983,
-1.44585806316001));
#75529=CARTESIAN_POINT('Ctrl Pts',(-0.122543342896592,0.267979077768812,
-1.44675405012232));
#75530=CARTESIAN_POINT('Ctrl Pts',(-0.107190573388433,0.274479862674681,
-1.44765003708463));
#75531=CARTESIAN_POINT('Ctrl Pts',(-0.0914176440317826,0.279636289418377,
-1.44854602404694));
#75532=CARTESIAN_POINT('Ctrl Pts',(-0.0756068246035106,0.284805103041784,
-1.44944416336849));
#75533=CARTESIAN_POINT('Ctrl Pts',(-0.059374593239593,0.288622886440156,
-1.45034230269004));
#75534=CARTESIAN_POINT('Ctrl Pts',(-0.0429731215838286,0.291044585624508,
-1.45124044201158));
#75535=CARTESIAN_POINT('Ctrl Pts',(-0.0281852665924153,0.293228032154346,
-1.4520502202027));
#75536=CARTESIAN_POINT('Ctrl Pts',(-0.0132604109650671,0.29427724548344,
-1.45285999839382));
#75537=CARTESIAN_POINT('Ctrl Pts',(0.0016153759589386,0.294195565161189,
-1.45366977658494));
#75538=CARTESIAN_POINT('Ctrl Pts',(0.0181141778322444,0.294104973150113,
-1.45456790520193));
#75539=CARTESIAN_POINT('Ctrl Pts',(0.0346580897687213,0.292621863149287,
-1.45546603381891));
#75540=CARTESIAN_POINT('Ctrl Pts',(0.0509931230950487,0.289747030005509,
-1.4563641624359));
#75541=CARTESIAN_POINT('Ctrl Pts',(0.0672964031397914,0.286877785181295,
-1.45726054520209));
#75542=CARTESIAN_POINT('Ctrl Pts',(0.0833908285708099,0.282622257540847,
-1.45815692796828));
#75543=CARTESIAN_POINT('Ctrl Pts',(0.0990270367417756,0.277033005243316,
-1.45905331073447));
#75544=CARTESIAN_POINT('Ctrl Pts',(0.114660536496952,0.271444721084543,
-1.4599495382343));
#75545=CARTESIAN_POINT('Ctrl Pts',(0.129835215689528,0.264523386482975,
-1.46084576573413));
#75546=CARTESIAN_POINT('Ctrl Pts',(0.144316649727445,0.256371497268019,
-1.46174199323395));
#75547=CARTESIAN_POINT('Ctrl Pts',(0.158794197109105,0.248221795929702,
-1.46263798019626));
#75548=CARTESIAN_POINT('Ctrl Pts',(0.172578184052074,0.238842593409423,
-1.46353396715856));
#75549=CARTESIAN_POINT('Ctrl Pts',(0.185460089444515,0.228381687582942,
-1.46442995412087));
#75550=CARTESIAN_POINT('Ctrl Pts',(0.198372940028361,0.217895652342511,
-1.46532809344241));
#75551=CARTESIAN_POINT('Ctrl Pts',(0.210378780468628,0.206323245486166,
-1.46622623276395));
#75552=CARTESIAN_POINT('Ctrl Pts',(0.221303078006792,0.193851973589953,
-1.4671243720855));
#75553=CARTESIAN_POINT('Ctrl Pts',(0.231152616589269,0.182607655748445,
-1.46793415027664));
#75554=CARTESIAN_POINT('Ctrl Pts',(0.240123198351401,0.170633482417109,
-1.46874392846778));
#75555=CARTESIAN_POINT('Ctrl Pts',(0.248116785828277,0.158087635791812,
-1.46955370665893));
#75556=CARTESIAN_POINT('Ctrl Pts',(0.256982509484536,0.144172981134509,
-1.47045183527593));
#75557=CARTESIAN_POINT('Ctrl Pts',(0.264702412415536,0.129465712993,-1.47134996389294));
#75558=CARTESIAN_POINT('Ctrl Pts',(0.27113950834701,0.114179713668155,-1.47224809250995));
#75559=CARTESIAN_POINT('Ctrl Pts',(0.277564091361269,0.098923428432728,
-1.47314447527617));
#75560=CARTESIAN_POINT('Ctrl Pts',(0.282710452419854,0.083091340341732,
-1.47404085804238));
#75561=CARTESIAN_POINT('Ctrl Pts',(0.286487614189603,0.0669214981597798,
-1.4749372408086));
#75562=CARTESIAN_POINT('Ctrl Pts',(0.290264121700693,0.0507544568266919,
-1.47583346830845));
#75563=CARTESIAN_POINT('Ctrl Pts',(0.292671669559208,0.0342505338207423,
-1.4767296958083));
#75564=CARTESIAN_POINT('Ctrl Pts',(0.29366934391778,0.0176622887220424,
-1.47762592330815));
#75565=CARTESIAN_POINT('Ctrl Pts',(0.29466675051162,0.00107849572432326,
-1.47852191027048));
#75566=CARTESIAN_POINT('Ctrl Pts',(0.294254998032437,-0.0155887834738292,
-1.47941789723281));
#75567=CARTESIAN_POINT('Ctrl Pts',(0.292445283283392,-0.032084206165911,
-1.48031388419514));
#75568=CARTESIAN_POINT('Ctrl Pts',(0.290631221198485,-0.048619254518705,
-1.4812120235167));
#75569=CARTESIAN_POINT('Ctrl Pts',(0.287412602456615,-0.0649808344709505,
-1.48211016283827));
#75570=CARTESIAN_POINT('Ctrl Pts',(0.28285241563517,-0.0809206461253819,
-1.48300830215983));
#75571=CARTESIAN_POINT('Ctrl Pts',(0.278740871082607,-0.0952922603470733,
-1.48381808035086));
#75572=CARTESIAN_POINT('Ctrl Pts',(0.273539589296867,-0.109320761045354,
-1.48462785854189));
#75573=CARTESIAN_POINT('Ctrl Pts',(0.267328372871686,-0.122838027734805,
-1.48543763673292));
#75574=CARTESIAN_POINT('Ctrl Pts',(0.260439484927435,-0.137830088735717,
-1.48633576534989));
#75575=CARTESIAN_POINT('Ctrl Pts',(0.252263485818446,-0.152288777334707,
-1.48723389396687));
#75576=CARTESIAN_POINT('Ctrl Pts',(0.242905879293824,-0.165983052762908,
-1.48813202258385));
#75577=CARTESIAN_POINT('Ctrl Pts',(0.233566462797283,-0.179650708215805,
-1.48902840535003));
#75578=CARTESIAN_POINT('Ctrl Pts',(0.223050384801855,-0.192556216692559,
-1.48992478811622));
#75579=CARTESIAN_POINT('Ctrl Pts',(0.211508393968693,-0.204494105736044,
-1.4908211708824));
#75580=CARTESIAN_POINT('Ctrl Pts',(0.199968402374078,-0.216429926965726,
-1.49171739838222));
#75581=CARTESIAN_POINT('Ctrl Pts',(0.187403360995642,-0.227397857327417,
-1.49261362588204));
#75582=CARTESIAN_POINT('Ctrl Pts',(0.174003346263128,-0.237226633178558,
-1.49350985338186));
#75583=CARTESIAN_POINT('Ctrl Pts',(0.160606927945919,-0.247052771095292,
-1.49440584034416));
#75584=CARTESIAN_POINT('Ctrl Pts',(0.146376625954696,-0.255739901875646,
-1.49530182730646));
#75585=CARTESIAN_POINT('Ctrl Pts',(0.131533098065914,-0.263159047180945,
-1.49619781426876));
#75586=CARTESIAN_POINT('Ctrl Pts',(0.116653912733785,-0.270596014917365,
-1.49709595359029));
#75587=CARTESIAN_POINT('Ctrl Pts',(0.101159282176131,-0.276758581671856,
-1.49799409291183));
#75588=CARTESIAN_POINT('Ctrl Pts',(0.0852920150001993,-0.281565111789806,
-1.49889223223336));
#75589=CARTESIAN_POINT('Ctrl Pts',(0.0709858081516357,-0.285898763787268,
-1.49970201042454));
#75590=CARTESIAN_POINT('Ctrl Pts',(0.056377348170839,-0.289130645766822,
-1.50051178861573));
#75591=CARTESIAN_POINT('Ctrl Pts',(0.0416511737591101,-0.291236707378188,
-1.50132156680691));
#75592=CARTESIAN_POINT('Ctrl Pts',(0.0253183077946819,-0.29357254973952,
-1.50221969542386));
#75593=CARTESIAN_POINT('Ctrl Pts',(0.00873611107200796,-0.294537634849432,
-1.50311782404082));
#75594=CARTESIAN_POINT('Ctrl Pts',(-0.00784407038384531,-0.294095410640515,
-1.50401595265778));
#75595=CARTESIAN_POINT('Ctrl Pts',(-0.0243920220204992,-0.293654046060688,
-1.50491233542394));
#75596=CARTESIAN_POINT('Ctrl Pts',(-0.0409371823563882,-0.29181075690919,
-1.50580871819011));
#75597=CARTESIAN_POINT('Ctrl Pts',(-0.0572251715302886,-0.288580872102309,
-1.50670510095627));
#75598=CARTESIAN_POINT('Ctrl Pts',(-0.0735103393905747,-0.285351546757855,
-1.50760132845607));
#75599=CARTESIAN_POINT('Ctrl Pts',(-0.0895376402263333,-0.280736203957116,
-1.50849755595587));
#75600=CARTESIAN_POINT('Ctrl Pts',(-0.105060128714307,-0.274801763739852,
-1.50939378345567));
#75601=CARTESIAN_POINT('Ctrl Pts',(-0.12057845113855,-0.268868916260516,
-1.51028977041794));
#75602=CARTESIAN_POINT('Ctrl Pts',(-0.135591494493943,-0.261617967001758,
-1.51118575738022));
#75603=CARTESIAN_POINT('Ctrl Pts',(-0.149871275757871,-0.253164453868841,
-1.5120817443425));
#75604=CARTESIAN_POINT('Ctrl Pts',(-0.164185360220829,-0.244690633524058,
-1.51297988366401));
#75605=CARTESIAN_POINT('Ctrl Pts',(-0.177761993823932,-0.235008907174037,
-1.51387802298553));
#75606=CARTESIAN_POINT('Ctrl Pts',(-0.190400975143691,-0.224279086551403,
-1.51477616230704));
#75607=CARTESIAN_POINT('Ctrl Pts',(-0.201796502750187,-0.214604891770623,
-1.51558594049833));
#75608=CARTESIAN_POINT('Ctrl Pts',(-0.212429917431785,-0.20407955774231,
-1.51639571868961));
#75609=CARTESIAN_POINT('Ctrl Pts',(-0.222180992872592,-0.192845135811483,
-1.5172054968809));
#75610=CARTESIAN_POINT('Ctrl Pts',(-0.232910731838629,-0.180483174765868,
-1.51809654819781));
#75611=CARTESIAN_POINT('Ctrl Pts',(-0.242642934871774,-0.167179753567899,
-1.51898759951473));
#75612=CARTESIAN_POINT('Ctrl Pts',(-0.251211342293677,-0.153122504887457,
-1.51987865083165));
#75613=CARTESIAN_POINT('Ctrl Pts',(-0.259762998908044,-0.139092737424413,
-1.52076796018785));
#75614=CARTESIAN_POINT('Ctrl Pts',(-0.267154899328252,-0.124312709262806,
-1.52165726954405));
#75615=CARTESIAN_POINT('Ctrl Pts',(-0.273262529657102,-0.109001054515089,
-1.52254657890025));
#75616=CARTESIAN_POINT('Ctrl Pts',(-0.27936345814298,-0.0937062010962422,
-1.523434912426));
#75617=CARTESIAN_POINT('Ctrl Pts',(-0.284182590563843,-0.0778816129895165,
-1.52432324595175));
#75618=CARTESIAN_POINT('Ctrl Pts',(-0.287642940184411,-0.061767134967291,
-1.5252115794775));
#75619=CARTESIAN_POINT('Ctrl Pts',(-0.291104585625806,-0.0456466224460921,
-1.52610024566359));
#75620=CARTESIAN_POINT('Ctrl Pts',(-0.293206265845959,-0.0292367899534084,
-1.52698891184968));
#75621=CARTESIAN_POINT('Ctrl Pts',(-0.293921926337035,-0.0127883235150905,
-1.52787757803577));
#75622=CARTESIAN_POINT('Ctrl Pts',(-0.294111125559157,-0.00843984110753895,
-1.52811251478753));
#75623=CARTESIAN_POINT('Ctrl Pts',(-0.294203735878343,-0.00408867950520032,
-1.52834745153928));
#75624=CARTESIAN_POINT('Ctrl Pts',(-0.294199884656848,0.000260514677417675,
-1.52858238829104));
#75625=CARTESIAN_POINT('',(-0.294247201503143,-2.16877952208041E-5,-1.62858238829104));
#75626=CARTESIAN_POINT('Ctrl Pts',(-0.294053336475258,0.000261715132789226,
-1.52858246018345));
#75627=CARTESIAN_POINT('Ctrl Pts',(-0.29428999687239,0.0280593677207072,
-1.53008478244059));
#75628=CARTESIAN_POINT('Ctrl Pts',(-0.27791468735522,0.153550929214129,
-1.53688174805573));
#75629=CARTESIAN_POINT('Ctrl Pts',(-0.0993136717012497,0.333300171830814,
-1.54897335702887));
#75630=CARTESIAN_POINT('Ctrl Pts',(0.226279686422242,0.264101710371244,
-1.56485728710286));
#75631=CARTESIAN_POINT('Ctrl Pts',(0.34458731149564,-0.0470297212362109,
-1.58074121717685));
#75632=CARTESIAN_POINT('Ctrl Pts',(0.147232339525018,-0.315079114138717,
-1.59662514725084));
#75633=CARTESIAN_POINT('Ctrl Pts',(-0.184996265602307,-0.294497184254118,
-1.61250907732483));
#75634=CARTESIAN_POINT('Ctrl Pts',(-0.294150424933899,-0.0997705721318655,
-1.6231614910049));
#75635=CARTESIAN_POINT('Ctrl Pts',(-0.294682912919936,-0.00118332006191642,
-1.62851926132696));
#75636=CARTESIAN_POINT('Ctrl Pts',(-0.294681679645924,-2.17198188829926E-5,
-1.62858238829104));
#75637=CARTESIAN_POINT('',(-0.294199895814294,-0.000247594141307502,-1.72858238519529));
#75638=CARTESIAN_POINT('Ctrl Pts',(-0.294199999200868,-2.1684316126153E-5,
-1.62858238829104));
#75639=CARTESIAN_POINT('Ctrl Pts',(-0.29420121277264,0.0164433410297652,
-1.6294786423153));
#75640=CARTESIAN_POINT('Ctrl Pts',(-0.292815900108825,0.0329621383935221,
-1.63037489633957));
#75641=CARTESIAN_POINT('Ctrl Pts',(-0.290043036332427,0.0492816099074137,
-1.63127115036383));
#75642=CARTESIAN_POINT('Ctrl Pts',(-0.2872755512891,0.0655694253111555,
-1.63216566585655));
#75643=CARTESIAN_POINT('Ctrl Pts',(-0.283125922858897,0.0816578962341241,
-1.63306018134926));
#75644=CARTESIAN_POINT('Ctrl Pts',(-0.277644920689935,0.097298191222036,
-1.63395469684197));
#75645=CARTESIAN_POINT('Ctrl Pts',(-0.27216484128538,0.112935853058729,
-1.63484906173685));
#75646=CARTESIAN_POINT('Ctrl Pts',(-0.265354045538873,0.128124723155489,
-1.63574342663173));
#75647=CARTESIAN_POINT('Ctrl Pts',(-0.25731332445106,0.142630617540357,
-1.63663779152661));
#75648=CARTESIAN_POINT('Ctrl Pts',(-0.249274583937638,0.157132938862234,
-1.63753193612331));
#75649=CARTESIAN_POINT('Ctrl Pts',(-0.240006915751063,0.170951928661847,
-1.63842608072001));
#75650=CARTESIAN_POINT('Ctrl Pts',(-0.229656536750084,0.183879077461133,
-1.63932022531671));
#75651=CARTESIAN_POINT('Ctrl Pts',(-0.21928162150504,0.196836870904251,
-1.64021648954111));
#75652=CARTESIAN_POINT('Ctrl Pts',(-0.207819391914967,0.208897996777179,
-1.64111275376552));
#75653=CARTESIAN_POINT('Ctrl Pts',(-0.195455862100078,0.219887803142228,
-1.64200901798992));
#75654=CARTESIAN_POINT('Ctrl Pts',(-0.18502757939023,0.229157389531967,
-1.64276499115088));
#75655=CARTESIAN_POINT('Ctrl Pts',(-0.173958958957302,0.237665280750663,
-1.64352096431184));
#75656=CARTESIAN_POINT('Ctrl Pts',(-0.162378246516628,0.245330277499915,
-1.6442769374728));
#75657=CARTESIAN_POINT('Ctrl Pts',(-0.148619862282732,0.254436623155937,
-1.64517506608728));
#75658=CARTESIAN_POINT('Ctrl Pts',(-0.134049059683587,0.262411104138865,
-1.64607319470175));
#75659=CARTESIAN_POINT('Ctrl Pts',(-0.11887730661778,0.269113035677022,
-1.64697132331623));
#75660=CARTESIAN_POINT('Ctrl Pts',(-0.103735045563376,0.275801939489215,
-1.64786770607977));
#75661=CARTESIAN_POINT('Ctrl Pts',(-0.0879948416570457,0.281222827286779,
-1.64876408884331));
#75662=CARTESIAN_POINT('Ctrl Pts',(-0.0718931256591281,0.285280596050557,
-1.64966047160685));
#75663=CARTESIAN_POINT('Ctrl Pts',(-0.0557941987129142,0.28933766194969,
-1.65055669910384));
#75664=CARTESIAN_POINT('Ctrl Pts',(-0.0393346361284934,0.29203183324509,
-1.65145292660083));
#75665=CARTESIAN_POINT('Ctrl Pts',(-0.0227662478442387,0.293317810504399,
-1.65234915409782));
#75666=CARTESIAN_POINT('Ctrl Pts',(-0.00620230633356539,0.294603442621525,
-1.65324514105718));
#75667=CARTESIAN_POINT('Ctrl Pts',(0.0104696126877779,0.294481580486408,
-1.65414112801655));
#75668=CARTESIAN_POINT('Ctrl Pts',(0.0269940104210207,0.2929589790421,-1.65503711497591));
#75669=CARTESIAN_POINT('Ctrl Pts',(0.043558103417585,0.291432719971885,
-1.6559352542944));
#75670=CARTESIAN_POINT('Ctrl Pts',(0.0599731781454324,0.288499100173501,
-1.6568333936129));
#75671=CARTESIAN_POINT('Ctrl Pts',(0.0759898769403874,0.284216781001025,
-1.65773153293139));
#75672=CARTESIAN_POINT('Ctrl Pts',(0.09043081425966,0.280355766721958,-1.65854131113652));
#75673=CARTESIAN_POINT('Ctrl Pts',(0.104547639415254,0.275399213522471,
-1.65935108934165));
#75674=CARTESIAN_POINT('Ctrl Pts',(0.118170869641054,0.26942398847964,-1.66016086754679));
#75675=CARTESIAN_POINT('Ctrl Pts',(0.133280455635432,0.262796839475768,
-1.66105899620086));
#75676=CARTESIAN_POINT('Ctrl Pts',(0.147879131436968,0.254873498987716,
-1.66195712485493));
#75677=CARTESIAN_POINT('Ctrl Pts',(0.161734056589533,0.24575543725235,-1.662855253509));
#75678=CARTESIAN_POINT('Ctrl Pts',(0.175562049487036,0.236655099897421,
-1.66375163631243));
#75679=CARTESIAN_POINT('Ctrl Pts',(0.188648471582833,0.226365025870775,
-1.66464801911586));
#75680=CARTESIAN_POINT('Ctrl Pts',(0.200785260103042,0.215032368087583,
-1.66554440191929));
#75681=CARTESIAN_POINT('Ctrl Pts',(0.212919946352997,0.203701673287377,
-1.66644062945604));
#75682=CARTESIAN_POINT('Ctrl Pts',(0.224104712626763,0.191329252934774,
-1.66733685699279));
#75683=CARTESIAN_POINT('Ctrl Pts',(0.23416501592168,0.178102176624541,-1.66823308452953));
#75684=CARTESIAN_POINT('Ctrl Pts',(0.244222619141691,0.16487865031631,-1.66912907152865));
#75685=CARTESIAN_POINT('Ctrl Pts',(0.253155887786595,0.150801560128604,
-1.67002505852777));
#75686=CARTESIAN_POINT('Ctrl Pts',(0.260832025983922,0.136089287679533,
-1.67092104552689));
#75687=CARTESIAN_POINT('Ctrl Pts',(0.268526603957315,0.121341673108887,
-1.67181918488429));
#75688=CARTESIAN_POINT('Ctrl Pts',(0.274957675540732,0.105956545726213,
-1.67271732424169));
#75689=CARTESIAN_POINT('Ctrl Pts',(0.280039395205683,0.090175257875071,
-1.67361546359909));
#75690=CARTESIAN_POINT('Ctrl Pts',(0.284621161709583,0.0759465752967122,
-1.67442524160632));
#75691=CARTESIAN_POINT('Ctrl Pts',(0.288106581174604,0.0613965267213745,
-1.67523501961355));
#75692=CARTESIAN_POINT('Ctrl Pts',(0.290468397946582,0.0467092045998036,
-1.67604479762078));
#75693=CARTESIAN_POINT('Ctrl Pts',(0.293087899899455,0.0304194274094599,
-1.67694292617016));
#75694=CARTESIAN_POINT('Ctrl Pts',(0.294341187685413,0.0138565209953559,
-1.67784105471955));
#75695=CARTESIAN_POINT('Ctrl Pts',(0.294187344085231,-0.00272884225966128,
-1.67873918326893));
#75696=CARTESIAN_POINT('Ctrl Pts',(0.294033799537936,-0.0192819656244967,
-1.67963556596775));
#75697=CARTESIAN_POINT('Ctrl Pts',(0.292478494041894,-0.0358566762777647,
-1.68053194866657));
#75698=CARTESIAN_POINT('Ctrl Pts',(0.289532330761364,-0.0521983662952416,
-1.68142833136539));
#75699=CARTESIAN_POINT('Ctrl Pts',(0.286586677794322,-0.0685372257211849,
-1.68232455879916));
#75700=CARTESIAN_POINT('Ctrl Pts',(0.282250733049956,-0.0846423586988476,
-1.68322078623293));
#75701=CARTESIAN_POINT('Ctrl Pts',(0.276587112295275,-0.100265693595371,
-1.6841170136667));
#75702=CARTESIAN_POINT('Ctrl Pts',(0.270925011589871,-0.115884835372345,
-1.68501300056356));
#75703=CARTESIAN_POINT('Ctrl Pts',(0.263936222243119,-0.131021695103706,
-1.68590898746042));
#75704=CARTESIAN_POINT('Ctrl Pts',(0.255732300272781,-0.145446315172273,
-1.68680497435728));
#75705=CARTESIAN_POINT('Ctrl Pts',(0.247508670640721,-0.159905586415461,
-1.68770311361574));
#75706=CARTESIAN_POINT('Ctrl Pts',(0.238064494217003,-0.173648522751832,
-1.6886012528742));
#75707=CARTESIAN_POINT('Ctrl Pts',(0.227556077247711,-0.186472174084054,
-1.68949939213267));
#75708=CARTESIAN_POINT('Ctrl Pts',(0.218081499371173,-0.198034208933238,
-1.69030917065337));
#75709=CARTESIAN_POINT('Ctrl Pts',(0.207742657805406,-0.20884904599276,
-1.69111894917406));
#75710=CARTESIAN_POINT('Ctrl Pts',(0.196679491990959,-0.21879400684246,
-1.69192872769476));
#75711=CARTESIAN_POINT('Ctrl Pts',(0.184409290188552,-0.229824003010781,
-1.69282685631643));
#75712=CARTESIAN_POINT('Ctrl Pts',(0.171169103881296,-0.239853863539452,
-1.6937249849381));
#75713=CARTESIAN_POINT('Ctrl Pts',(0.157147421701379,-0.248713344741711,
-1.69462311355977));
#75714=CARTESIAN_POINT('Ctrl Pts',(0.143152995950657,-0.257555604199888,
-1.69551949632964));
#75715=CARTESIAN_POINT('Ctrl Pts',(0.128380715715764,-0.265231526367482,
-1.6964158790995));
#75716=CARTESIAN_POINT('Ctrl Pts',(0.11305046214597,-0.271612284347713,
-1.69731226186936));
#75717=CARTESIAN_POINT('Ctrl Pts',(0.0977228640231671,-0.277991937077823,
-1.69820848937128));
#75718=CARTESIAN_POINT('Ctrl Pts',(0.0818381924911331,-0.283076518770903,
-1.6991047168732));
#75719=CARTESIAN_POINT('Ctrl Pts',(0.0656388622976581,-0.286784204161019,
-1.70000094437512));
#75720=CARTESIAN_POINT('Ctrl Pts',(0.0494438798402572,-0.290490894445947,
-1.70089693133866));
#75721=CARTESIAN_POINT('Ctrl Pts',(0.0329351805694026,-0.292821255920828,
-1.7017929183022));
#75722=CARTESIAN_POINT('Ctrl Pts',(0.0163664804088447,-0.293744409851536,
-1.70268890526574));
#75723=CARTESIAN_POINT('Ctrl Pts',(-0.000242021414697736,-0.294669781401083,
-1.70358704458708));
#75724=CARTESIAN_POINT('Ctrl Pts',(-0.0169100168106484,-0.294181175863316,
-1.70448518390843));
#75725=CARTESIAN_POINT('Ctrl Pts',(-0.0333822336270742,-0.292299959764054,
-1.70538332322978));
#75726=CARTESIAN_POINT('Ctrl Pts',(-0.0482338734912188,-0.290603822302761,
-1.70619310140944));
#75727=CARTESIAN_POINT('Ctrl Pts',(-0.0629259751805142,-0.287776401659202,
-1.70700287958909));
#75728=CARTESIAN_POINT('Ctrl Pts',(-0.0772795972649593,-0.283868814501639,
-1.70781265776875));
#75729=CARTESIAN_POINT('Ctrl Pts',(-0.0931992682033539,-0.279534890886712,
-1.70871078662273));
#75730=CARTESIAN_POINT('Ctrl Pts',(-0.108804129565062,-0.273843750169649,
-1.70960891547671));
#75731=CARTESIAN_POINT('Ctrl Pts',(-0.123848953646058,-0.266861530912151,
-1.71050704433069));
#75732=CARTESIAN_POINT('Ctrl Pts',(-0.138864532481465,-0.259892884210625,
-1.71140342733516));
#75733=CARTESIAN_POINT('Ctrl Pts',(-0.153321497429455,-0.251638409840476,
-1.71229981033962));
#75734=CARTESIAN_POINT('Ctrl Pts',(-0.166992413577997,-0.242213075219723,
-1.71319619334408));
#75735=CARTESIAN_POINT('Ctrl Pts',(-0.180660961704508,-0.232789373218159,
-1.71409242108062));
#75736=CARTESIAN_POINT('Ctrl Pts',(-0.193543051582717,-0.222195617746181,
-1.71498864881717));
#75737=CARTESIAN_POINT('Ctrl Pts',(-0.205438535842917,-0.210591186878081,
-1.71588487655371));
#75738=CARTESIAN_POINT('Ctrl Pts',(-0.217330827482302,-0.198989870515176,
-1.71678086375231));
#75739=CARTESIAN_POINT('Ctrl Pts',(-0.228236479969677,-0.186378977846106,
-1.71767685095091));
#75740=CARTESIAN_POINT('Ctrl Pts',(-0.237992036393236,-0.172954995919171,
-1.71857283814951));
#75741=CARTESIAN_POINT('Ctrl Pts',(-0.247771027756986,-0.159498766706699,
-1.71947097770165));
#75742=CARTESIAN_POINT('Ctrl Pts',(-0.256393959006673,-0.145226205702012,
-1.72036911725379));
#75743=CARTESIAN_POINT('Ctrl Pts',(-0.263740436603473,-0.130363423168501,
-1.72126725680593));
#75744=CARTESIAN_POINT('Ctrl Pts',(-0.27036413852692,-0.116962900270577,
-1.7220770338182));
#75745=CARTESIAN_POINT('Ctrl Pts',(-0.275950650625105,-0.103083332767034,
-1.72288681083047));
#75746=CARTESIAN_POINT('Ctrl Pts',(-0.280445950538711,-0.0889028055037576,
-1.72369658784274));
#75747=CARTESIAN_POINT('Ctrl Pts',(-0.28642702932571,-0.0700353545143065,
-1.72477401097431));
#75748=CARTESIAN_POINT('Ctrl Pts',(-0.290508007507302,-0.0505380932922465,
-1.72585143410589));
#75749=CARTESIAN_POINT('Ctrl Pts',(-0.292587171686153,-0.0307634030090615,
-1.72692885723746));
#75750=CARTESIAN_POINT('Ctrl Pts',(-0.29365080707009,-0.0206472897624244,
-1.7274800332234));
#75751=CARTESIAN_POINT('Ctrl Pts',(-0.294191302124979,-0.0104589120974399,
-1.72803120920935));
#75752=CARTESIAN_POINT('Ctrl Pts',(-0.294199895814294,-0.000247594141307502,
-1.72858238519529));
#75753=CARTESIAN_POINT('',(-0.293800095830876,0.000157032384922304,-1.82858238829104));
#75754=CARTESIAN_POINT('Ctrl Pts',(-0.293989435543949,-0.000247359708936523,
-1.72858238829104));
#75755=CARTESIAN_POINT('Ctrl Pts',(-0.293449229871738,0.0676232139930559,
-1.7322484314996));
#75756=CARTESIAN_POINT('Ctrl Pts',(-0.23631160546398,0.234336140108229,
-1.74120911806615));
#75757=CARTESIAN_POINT('Ctrl Pts',(0.0410305566082919,0.345352959227952,
-1.75546444799072));
#75758=CARTESIAN_POINT('Ctrl Pts',(0.312471262641183,0.152689102424562,
-1.7713483780647));
#75759=CARTESIAN_POINT('Ctrl Pts',(0.297669529109044,-0.179847460151632,
-1.7872323081387));
#75760=CARTESIAN_POINT('Ctrl Pts',(0.0101848190520429,-0.347632316485115,
-1.80311623821267));
#75761=CARTESIAN_POINT('Ctrl Pts',(-0.247377757960732,-0.216891255039904,
-1.81689959826346));
#75762=CARTESIAN_POINT('Ctrl Pts',(-0.293514181780463,-0.059071809807225,
-1.82538831495625));
#75763=CARTESIAN_POINT('Ctrl Pts',(-0.293800095830876,0.000157032384922304,
-1.82858238829104));
#75764=CARTESIAN_POINT('Ctrl Pts',(-0.293800095830876,0.000157032384922304,
-1.82858238829104));
#75765=CARTESIAN_POINT('Ctrl Pts',(-0.293988126104624,0.0391086522688038,
-1.83068295831425));
#75766=CARTESIAN_POINT('Ctrl Pts',(-0.268652541760571,0.176005752497631,
-1.83807817169543));
#75767=CARTESIAN_POINT('Ctrl Pts',(-0.0611792324801312,0.342355999552018,
-1.85076802843466));
#75768=CARTESIAN_POINT('Ctrl Pts',(0.254561196731867,0.23696743080658,-1.86665195850863));
#75769=CARTESIAN_POINT('Ctrl Pts',(0.337105175546461,-0.0855145454749233,
-1.88253588858261));
#75770=CARTESIAN_POINT('Ctrl Pts',(0.110846680674492,-0.32962749086264,
-1.89841981865661));
#75771=CARTESIAN_POINT('Ctrl Pts',(-0.205921254452606,-0.273790960216194,
-1.91376860488588));
#75772=CARTESIAN_POINT('Ctrl Pts',(-0.293956888266034,-0.0874827880384833,
-1.92382274775716));
#75773=CARTESIAN_POINT('Ctrl Pts',(-0.29455814428141,0.000186008385503332,
-1.92858224727044));
#75774=CARTESIAN_POINT('Origin',(0.,0.,-2.1456589891905));
#75775=CARTESIAN_POINT('',(0.223395701213113,0.0796639272475426,-0.0400000000000001));
#75776=CARTESIAN_POINT('Ctrl Pts',(0.223395701213113,0.0796639272475426,
-0.0400000000000001));
#75777=CARTESIAN_POINT('Ctrl Pts',(0.229242148634165,0.0632691640673004,
-0.0412368761336291));
#75778=CARTESIAN_POINT('Ctrl Pts',(0.233267330333748,0.0462771952834835,
-0.0425283651739515));
#75779=CARTESIAN_POINT('Ctrl Pts',(0.236585845934182,0.0193347385838108,
-0.0444885583085567));
#75780=CARTESIAN_POINT('Ctrl Pts',(0.237180042016459,0.00961060863350905,
-0.0451798378362018));
#75781=CARTESIAN_POINT('Ctrl Pts',(0.237173010784732,-0.00387785704994729,
-0.0461134218510738));
#75782=CARTESIAN_POINT('Ctrl Pts',(0.237081916435321,-0.00763167680734785,
-0.0463705998105068));
#75783=CARTESIAN_POINT('Ctrl Pts',(0.236823643821842,-0.0130073167037052,
-0.0467353421644926));
#75784=CARTESIAN_POINT('Ctrl Pts',(0.236728825808623,-0.0146318767989615,
-0.0468451067693097));
#75785=CARTESIAN_POINT('Ctrl Pts',(0.236534578904014,-0.0174593844560919,
-0.0470353811864949));
#75786=CARTESIAN_POINT('Ctrl Pts',(0.236442674242972,-0.0186627707240716,
-0.0471161192616475));
#75787=CARTESIAN_POINT('Ctrl Pts',(0.236234211652528,-0.0211428780630218,
-0.0472820379831441));
#75788=CARTESIAN_POINT('Ctrl Pts',(0.236116479399246,-0.0224194627869977,
-0.047367179761603));
#75789=CARTESIAN_POINT('Ctrl Pts',(0.23578782996851,-0.0256926126158978,
-0.0475848505698601));
#75790=CARTESIAN_POINT('Ctrl Pts',(0.235561899772033,-0.0276875943320591,
-0.0477169157953027));
#75791=CARTESIAN_POINT('Ctrl Pts',(0.234548202232191,-0.0357245793533611,
-0.0482467916099474));
#75792=CARTESIAN_POINT('Ctrl Pts',(0.23355304297225,-0.0417383567309479,
-0.0486382574837735));
#75793=CARTESIAN_POINT('Ctrl Pts',(0.229072898625128,-0.063555865774956,
-0.0500497146380798));
#75794=CARTESIAN_POINT('Ctrl Pts',(0.224205536799736,-0.0790293111931186,
-0.0510307340489809));
#75795=CARTESIAN_POINT('Ctrl Pts',(0.217490502406841,-0.0946069579237412,
-0.0520824257994189));
#75796=CARTESIAN_POINT('Ctrl Pts',(0.217176625344077,-0.0953252774328842,
-0.0521310789593419));
#75797=CARTESIAN_POINT('Ctrl Pts',(0.213357409630695,-0.103948919518178,
-0.0527172112680231));
#75798=CARTESIAN_POINT('Ctrl Pts',(0.209426160764464,-0.111657573027881,
-0.0532616566732872));
#75799=CARTESIAN_POINT('Ctrl Pts',(0.20409553990101,-0.120834012840443,
-0.0539559133176723));
#75800=CARTESIAN_POINT('Ctrl Pts',(0.203086648436724,-0.1225220824665,-0.0540856382508694));
#75801=CARTESIAN_POINT('Ctrl Pts',(0.201608761797323,-0.124926459356141,
-0.0542736095376432));
#75802=CARTESIAN_POINT('Ctrl Pts',(0.201156666043024,-0.125653128619482,
-0.054330845175309));
#75803=CARTESIAN_POINT('Ctrl Pts',(0.200697140094571,-0.126382904802808,
-0.0543887726460091));
#75804=CARTESIAN_POINT('Ctrl Pts',(0.200693624082134,-0.126388488088569,
-0.054389215857151));
#75805=CARTESIAN_POINT('Ctrl Pts',(0.200686565097341,-0.126399696434068,
-0.0543901056486725));
#75806=CARTESIAN_POINT('Ctrl Pts',(0.200683022120862,-0.126405321492537,
-0.0543905522293519));
#75807=CARTESIAN_POINT('Ctrl Pts',(0.200675908027464,-0.126416615234073,
-0.0543914489080991));
#75808=CARTESIAN_POINT('Ctrl Pts',(0.20067233690698,-0.126422283914579,
-0.0543918990063852));
#75809=CARTESIAN_POINT('Ctrl Pts',(0.200665165308133,-0.126433666807838,
-0.0543928028731065));
#75810=CARTESIAN_POINT('Ctrl Pts',(0.200661564825264,-0.126439381019095,
-0.0543932566418665));
#75811=CARTESIAN_POINT('Ctrl Pts',(0.200654333244772,-0.126450856942442,
-0.0543941680072206));
#75812=CARTESIAN_POINT('Ctrl Pts',(0.200650702143052,-0.12645661865194,
-0.0543946256040756));
#75813=CARTESIAN_POINT('Ctrl Pts',(0.200643408026221,-0.126468191604891,
-0.0543955447885196));
#75814=CARTESIAN_POINT('Ctrl Pts',(0.200639745007662,-0.126474002844255,
-0.0543960063762747));
#75815=CARTESIAN_POINT('Ctrl Pts',(0.200632385716146,-0.126485676955469,
-0.0543969337107085));
#75816=CARTESIAN_POINT('Ctrl Pts',(0.20062868943874,-0.126491539824327,
-0.0543973994576657));
#75817=CARTESIAN_POINT('Ctrl Pts',(0.200621262243384,-0.126503319362767,
-0.0543983352843283));
#75818=CARTESIAN_POINT('Ctrl Pts',(0.2006175313199,-0.126509236030559,-0.0543988053644348));
#75819=CARTESIAN_POINT('Ctrl Pts',(0.200610033396785,-0.126521125411547,
-0.0543997500373972));
#75820=CARTESIAN_POINT('Ctrl Pts',(0.200606266392381,-0.126527098121203,
-0.0544002246305432));
#75821=CARTESIAN_POINT('Ctrl Pts',(0.200598694821391,-0.126539101908473,
-0.0544011785158827));
#75822=CARTESIAN_POINT('Ctrl Pts',(0.200594890249154,-0.126545132983368,
-0.0544016578084608));
#75823=CARTESIAN_POINT('Ctrl Pts',(0.200587242002331,-0.126557255907287,
-0.0544026212857213));
#75824=CARTESIAN_POINT('Ctrl Pts',(0.200583398322663,-0.126563347752089,
-0.0544031054707));
#75825=CARTESIAN_POINT('Ctrl Pts',(0.200575670264262,-0.126575594709312,
-0.0544040789328784));
#75826=CARTESIAN_POINT('Ctrl Pts',(0.200571785880057,-0.126581749817493,
-0.0544045682104059));
#75827=CARTESIAN_POINT('Ctrl Pts',(0.200563974756709,-0.126594125886275,
-0.0544055520651835));
#75828=CARTESIAN_POINT('Ctrl Pts',(0.200560048011122,-0.126600346843506,
-0.0544060466428653));
#75829=CARTESIAN_POINT('Ctrl Pts',(0.200552150445225,-0.126612857293882,
-0.0544070413134324));
#75830=CARTESIAN_POINT('Ctrl Pts',(0.200548179618808,-0.126619146782418,
-0.0544075414066874));
#75831=CARTESIAN_POINT('Ctrl Pts',(0.200540192105282,-0.126631797081026,
-0.0544085473321432));
#75832=CARTESIAN_POINT('Ctrl Pts',(0.200536175410803,-0.126638157887745,
-0.0544090531648523));
#75833=CARTESIAN_POINT('Ctrl Pts',(0.200528094304026,-0.126650953718181,
-0.0544100708018415));
#75834=CARTESIAN_POINT('Ctrl Pts',(0.200524029884712,-0.126657388737192,
-0.0544105826065634));
#75835=CARTESIAN_POINT('Ctrl Pts',(0.20051585139652,-0.126670336002805,
-0.0544116124295171));
#75836=CARTESIAN_POINT('Ctrl Pts',(0.200511737320095,-0.126676848244705,
-0.0544121304482347));
#75837=CARTESIAN_POINT('Ctrl Pts',(0.200503457507019,-0.126689953088422,
-0.0544131729509683));
#75838=CARTESIAN_POINT('Ctrl Pts',(0.20049929176263,-0.126696545684953,
-0.0544136974354696));
#75839=CARTESIAN_POINT('Ctrl Pts',(0.200490906519636,-0.126709814498762,
-0.0544147531319586));
#75840=CARTESIAN_POINT('Ctrl Pts',(0.20048668701253,-0.12671649071102,-0.0544152843445016));
#75841=CARTESIAN_POINT('Ctrl Pts',(0.200478192061428,-0.126729930153859,
-0.0544163537703289));
#75842=CARTESIAN_POINT('Ctrl Pts',(0.200473916608742,-0.12673669337872,
-0.0544168919841648));
#75843=CARTESIAN_POINT('Ctrl Pts',(0.200465307489914,-0.126750310389085,
-0.0544179756975492));
#75844=CARTESIAN_POINT('Ctrl Pts',(0.200460973814824,-0.126757164168214,
-0.0544185211976525));
#75845=CARTESIAN_POINT('Ctrl Pts',(0.2004537838742,-0.126768533887821,-0.054419426193448));
#75846=CARTESIAN_POINT('Ctrl Pts',(0.200450927806819,-0.126773049955175,
-0.0544197856764443));
#75847=CARTESIAN_POINT('Ctrl Pts',(0.200445019548975,-0.126782391504547,
-0.0544205293083176));
#75848=CARTESIAN_POINT('Ctrl Pts',(0.200441967336429,-0.126787216973569,
-0.0544209134586418));
#75849=CARTESIAN_POINT('Ctrl Pts',(0.200435650221673,-0.126797203370224,
-0.0544217085061467));
#75850=CARTESIAN_POINT('Ctrl Pts',(0.200432385295043,-0.126802364280933,
-0.0544221194048575));
#75851=CARTESIAN_POINT('Ctrl Pts',(0.200425624369565,-0.126813050447579,
-0.0544229702578859));
#75852=CARTESIAN_POINT('Ctrl Pts',(0.200422128340668,-0.12681857568648,
-0.0544234102141926));
#75853=CARTESIAN_POINT('Ctrl Pts',(0.200414884750506,-0.12683002264666,
-0.0544243217517066));
#75854=CARTESIAN_POINT('Ctrl Pts',(0.200411137156593,-0.126835944344308,
-0.0544247933349339));
#75855=CARTESIAN_POINT('Ctrl Pts',(0.200403367596856,-0.126848220079705,
-0.0544257709939155));
#75856=CARTESIAN_POINT('Ctrl Pts',(0.200399345590891,-0.126854574092906,
-0.05442627707228));
#75857=CARTESIAN_POINT('Ctrl Pts',(0.200391001625303,-0.126867754602532,
-0.0544273269329174));
#75858=CARTESIAN_POINT('Ctrl Pts',(0.200386679619657,-0.126874581068429,
-0.0544278707181186));
#75859=CARTESIAN_POINT('Ctrl Pts',(0.200377706901994,-0.126888751578943,
-0.0544289996012303));
#75860=CARTESIAN_POINT('Ctrl Pts',(0.200373056134776,-0.126896095589163,
-0.0544295847027166));
#75861=CARTESIAN_POINT('Ctrl Pts',(0.200363393455383,-0.126911352036645,
-0.054430800289052));
#75862=CARTESIAN_POINT('Ctrl Pts',(0.200358381478679,-0.126919264432039,
-0.054431430778038));
#75863=CARTESIAN_POINT('Ctrl Pts',(0.200347959637473,-0.126935715211567,
-0.0544327417492392));
#75864=CARTESIAN_POINT('Ctrl Pts',(0.200342549696038,-0.126944253546433,
-0.0544334222364082));
#75865=CARTESIAN_POINT('Ctrl Pts',(0.200331290129024,-0.126962021642882,
-0.0544348384467625));
#75866=CARTESIAN_POINT('Ctrl Pts',(0.200325440411186,-0.126971251346402,
-0.0544355741759215));
#75867=CARTESIAN_POINT('Ctrl Pts',(0.20031325352696,-0.126990476912724,
-0.054437106860315));
#75868=CARTESIAN_POINT('Ctrl Pts',(0.200306916249913,-0.127000472705921,
-0.0544379038227216));
#75869=CARTESIAN_POINT('Ctrl Pts',(0.20029369939146,-0.127021316219308,
-0.0544395658513579));
#75870=CARTESIAN_POINT('Ctrl Pts',(0.200286819678411,-0.127032163852739,
-0.0544404309260182));
#75871=CARTESIAN_POINT('Ctrl Pts',(0.200272454615401,-0.127054809993787,
-0.0544422371177047));
#75872=CARTESIAN_POINT('Ctrl Pts',(0.200264969103648,-0.127066608399492,
-0.054443178245233));
#75873=CARTESIAN_POINT('Ctrl Pts',(0.200249318899478,-0.127091270893961,
-0.0544451457586584));
#75874=CARTESIAN_POINT('Ctrl Pts',(0.200241154010927,-0.127104134856105,
-0.0544461721572159));
#75875=CARTESIAN_POINT('Ctrl Pts',(0.200226318960041,-0.127127502829,-0.0544480369171733));
#75876=CARTESIAN_POINT('Ctrl Pts',(0.200219649209185,-0.127138007103998,
-0.0544488752519425));
#75877=CARTESIAN_POINT('Ctrl Pts',(0.200202513634127,-0.127164989445355,
-0.0544510289288671));
#75878=CARTESIAN_POINT('Ctrl Pts',(0.200192046604907,-0.127181466740238,
-0.0544523443491516));
#75879=CARTESIAN_POINT('Ctrl Pts',(0.200155105019507,-0.127239604668286,
-0.0544569864645531));
#75880=CARTESIAN_POINT('Ctrl Pts',(0.200128619517845,-0.127281258288021,
-0.0544603138702484));
#75881=CARTESIAN_POINT('Ctrl Pts',(0.199748158275235,-0.127879195497085,
-0.0545081004141175));
#75882=CARTESIAN_POINT('Ctrl Pts',(0.199391891122265,-0.12843398729936,
-0.0545527101709068));
#75883=CARTESIAN_POINT('Ctrl Pts',(0.198536343300947,-0.129754136959971,
-0.0546595072140715));
#75884=CARTESIAN_POINT('Ctrl Pts',(0.198034952730123,-0.130518094905958,
-0.0547218290234923));
#75885=CARTESIAN_POINT('Ctrl Pts',(0.196382370235541,-0.133004653682108,
-0.0549263310661629));
#75886=CARTESIAN_POINT('Ctrl Pts',(0.195213056526881,-0.134715014307767,
-0.0550696094276162));
#75887=CARTESIAN_POINT('Ctrl Pts',(0.187132358221273,-0.146208542816238,
-0.0560491591106425));
#75888=CARTESIAN_POINT('Ctrl Pts',(0.179511437687025,-0.155470396876478,
-0.0569208452468902));
#75889=CARTESIAN_POINT('Ctrl Pts',(0.163902810340877,-0.171755093499542,
-0.0585664861289188));
#75890=CARTESIAN_POINT('Ctrl Pts',(0.156077517866197,-0.178896002122403,
-0.0593382776378411));
#75891=CARTESIAN_POINT('Ctrl Pts',(0.140491598256113,-0.191315033070328,
-0.0607630397227132));
#75892=CARTESIAN_POINT('Ctrl Pts',(0.132843524769311,-0.196702742587695,
-0.0614182504510669));
#75893=CARTESIAN_POINT('Ctrl Pts',(0.123021585651424,-0.202786917464426,
-0.0622071770197591));
#75894=CARTESIAN_POINT('Ctrl Pts',(0.121130583050321,-0.203922109763472,
-0.0623568184425714));
#75895=CARTESIAN_POINT('Ctrl Pts',(0.118087165740926,-0.205691835519322,
-0.0625941627852089));
#75896=CARTESIAN_POINT('Ctrl Pts',(0.11694486925447,-0.206343421478318,
-0.0626824751914192));
#75897=CARTESIAN_POINT('Ctrl Pts',(0.114769190859445,-0.207560595958415,
-0.0628492485818871));
#75898=CARTESIAN_POINT('Ctrl Pts',(0.11373690363406,-0.208128049532983,
-0.0629277742163327));
#75899=CARTESIAN_POINT('Ctrl Pts',(0.111378467038472,-0.209401707059572,
-0.063105837232709));
#75900=CARTESIAN_POINT('Ctrl Pts',(0.110049740122914,-0.210103052600945,
-0.0632052009302801));
#75901=CARTESIAN_POINT('Ctrl Pts',(0.105943058826969,-0.212221045683783,
-0.0635094563079053));
#75902=CARTESIAN_POINT('Ctrl Pts',(0.103143688473451,-0.213595610785489,
-0.0637128835617589));
#75903=CARTESIAN_POINT('Ctrl Pts',(0.0839101043146858,-0.222573469144085,
-0.0650857066937842));
#75904=CARTESIAN_POINT('Ctrl Pts',(0.0666790650596363,-0.228328368378285,
-0.066187684147284));
#75905=CARTESIAN_POINT('Ctrl Pts',(0.0448381780651893,-0.232936169444844,
-0.0675569835304955));
#75906=CARTESIAN_POINT('Ctrl Pts',(0.0406945805117616,-0.233695680349334,
-0.0678158930163265));
#75907=CARTESIAN_POINT('Ctrl Pts',(0.0301696114994126,-0.235336466706992,
-0.0684757787806644));
#75908=CARTESIAN_POINT('Ctrl Pts',(0.023768856740451,-0.236068819383293,
-0.0688791336764089));
#75909=CARTESIAN_POINT('Ctrl Pts',(0.0137275642480068,-0.2368052015335,
-0.069525711002115));
#75910=CARTESIAN_POINT('Ctrl Pts',(0.0101030129709715,-0.236987499939797,
-0.0697619087733305));
#75911=CARTESIAN_POINT('Ctrl Pts',(0.00536486025256381,-0.237116921263174,
-0.0700759910807173));
#75912=CARTESIAN_POINT('Ctrl Pts',(0.00425359434382207,-0.237139458734659,
-0.0701500362865578));
#75913=CARTESIAN_POINT('Ctrl Pts',(0.00243782708816929,-0.237163517233428,
-0.0702717067319259));
#75914=CARTESIAN_POINT('Ctrl Pts',(0.00173338935264927,-0.237169711885553,
-0.0703190775162847));
#75915=CARTESIAN_POINT('Ctrl Pts',(0.000360142134917721,-0.237175669557212,
-0.0704117688757194));
#75916=CARTESIAN_POINT('Ctrl Pts',(-0.000308651197940893,-0.237175742058156,
-0.0704570724444562));
#75917=CARTESIAN_POINT('Ctrl Pts',(-0.0018068708919154,-0.237169567694617,
-0.0705589109484881));
#75918=CARTESIAN_POINT('Ctrl Pts',(-0.00263628093352684,-0.237161798343516,
-0.0706155284544852));
#75919=CARTESIAN_POINT('Ctrl Pts',(-0.0055295702210324,-0.237119516888802,
-0.0708138289541566));
#75920=CARTESIAN_POINT('Ctrl Pts',(-0.00759295480567648,-0.237062413190828,
-0.0709566652065116));
#75921=CARTESIAN_POINT('Ctrl Pts',(-0.0218368899586364,-0.236482070691389,
-0.0719512896540136));
#75922=CARTESIAN_POINT('Ctrl Pts',(-0.0339609371229547,-0.235047260827278,
-0.0728403779867142));
#75923=CARTESIAN_POINT('Ctrl Pts',(-0.0566183719172663,-0.230575934993547,
-0.0745278089015591));
#75924=CARTESIAN_POINT('Ctrl Pts',(-0.0671595412626176,-0.227729073102524,
-0.0753239494707382));
#75925=CARTESIAN_POINT('Ctrl Pts',(-0.0831163325583045,-0.22221469410172,
-0.0765299836855675));
#75926=CARTESIAN_POINT('Ctrl Pts',(-0.0886892828642959,-0.220049804104411,
-0.0769515524117712));
#75927=CARTESIAN_POINT('Ctrl Pts',(-0.0979515320207506,-0.216042612797609,
-0.0776522300415399));
#75928=CARTESIAN_POINT('Ctrl Pts',(-0.101685187203332,-0.214310614720927,
-0.07793470630629));
#75929=CARTESIAN_POINT('Ctrl Pts',(-0.106861138388362,-0.211743808067834,
-0.0783265852228423));
#75930=CARTESIAN_POINT('Ctrl Pts',(-0.108342409660623,-0.210989728822862,
-0.078438770424016));
#75931=CARTESIAN_POINT('Ctrl Pts',(-0.110870918714153,-0.209668875711607,
-0.0786303687796769));
#75932=CARTESIAN_POINT('Ctrl Pts',(-0.11192202284175,-0.2091096816309,-0.0787100465633688));
#75933=CARTESIAN_POINT('Ctrl Pts',(-0.113921145129769,-0.208026743964054,
-0.0788616646966255));
#75934=CARTESIAN_POINT('Ctrl Pts',(-0.11486987053429,-0.20750437687515,
-0.0789336517283876));
#75935=CARTESIAN_POINT('Ctrl Pts',(-0.117083562742454,-0.20626568566774,
-0.0791017204709229));
#75936=CARTESIAN_POINT('Ctrl Pts',(-0.11834559751945,-0.205544188569614,
-0.0791976134647109));
#75937=CARTESIAN_POINT('Ctrl Pts',(-0.122052534778528,-0.203379495597458,
-0.0794795748395817));
#75938=CARTESIAN_POINT('Ctrl Pts',(-0.124478304401009,-0.201903921032023,
-0.0796644700421166));
#75939=CARTESIAN_POINT('Ctrl Pts',(-0.141419652375891,-0.191177230968593,
-0.0809600374885441));
#75940=CARTESIAN_POINT('Ctrl Pts',(-0.154917030248592,-0.18041355612816,
-0.0820098088353067));
#75941=CARTESIAN_POINT('Ctrl Pts',(-0.177082386753192,-0.158399797967705,
-0.0839226617382625));
#75942=CARTESIAN_POINT('Ctrl Pts',(-0.186135571550302,-0.147655340394726,
-0.0847823218684297));
#75943=CARTESIAN_POINT('Ctrl Pts',(-0.195164671528303,-0.134779969224629,
-0.0858137660865564));
#75944=CARTESIAN_POINT('Ctrl Pts',(-0.196128736414607,-0.133373188654349,
-0.0859264932023624));
#75945=CARTESIAN_POINT('Ctrl Pts',(-0.197536819723423,-0.131270206098783,
-0.0860952504988646));
#75946=CARTESIAN_POINT('Ctrl Pts',(-0.197992533731215,-0.13058184671035,
-0.0861505270739946));
#75947=CARTESIAN_POINT('Ctrl Pts',(-0.198767589085154,-0.12939773528402,
-0.0862457044692087));
#75948=CARTESIAN_POINT('Ctrl Pts',(-0.19908868897228,-0.128903150745055,
-0.0862854866995572));
#75949=CARTESIAN_POINT('Ctrl Pts',(-0.199818486361409,-0.127769824842621,
-0.0863767129294122));
#75950=CARTESIAN_POINT('Ctrl Pts',(-0.200225961271355,-0.127130326925791,
-0.0864282347117256));
#75951=CARTESIAN_POINT('Ctrl Pts',(-0.201335775554544,-0.125369995082972,
-0.086570159368804));
#75952=CARTESIAN_POINT('Ctrl Pts',(-0.20203180324681,-0.124245243209492,
-0.0866609536062306));
#75953=CARTESIAN_POINT('Ctrl Pts',(-0.205680085236808,-0.118238053191723,
-0.0871462310204833));
#75954=CARTESIAN_POINT('Ctrl Pts',(-0.208464601193013,-0.113256490952333,
-0.0875498545609662));
#75955=CARTESIAN_POINT('Ctrl Pts',(-0.218702192169865,-0.0932822322136545,
-0.0891595544137602));
#75956=CARTESIAN_POINT('Ctrl Pts',(-0.224739209200121,-0.0776179879845412,
-0.0903992235482619));
#75957=CARTESIAN_POINT('Ctrl Pts',(-0.231860148189455,-0.0510712781021315,
-0.0923759712771183));
#75958=CARTESIAN_POINT('Ctrl Pts',(-0.233935662075728,-0.0405162896788951,
-0.0931327866834833));
#75959=CARTESIAN_POINT('Ctrl Pts',(-0.235575466598854,-0.0275931283719011,
-0.0940229323734671));
#75960=CARTESIAN_POINT('Ctrl Pts',(-0.235829896139041,-0.025326703617522,
-0.0941777402842617));
#75961=CARTESIAN_POINT('Ctrl Pts',(-0.236180811944037,-0.0217341013475974,
-0.0944211502360611));
#75962=CARTESIAN_POINT('Ctrl Pts',(-0.236298899455012,-0.020410226184335,
-0.0945104225554074));
#75963=CARTESIAN_POINT('Ctrl Pts',(-0.236500159912637,-0.0179172661765964,
-0.0946777558405602));
#75964=CARTESIAN_POINT('Ctrl Pts',(-0.236585807552514,-0.0167484272430532,
-0.094755891744372));
#75965=CARTESIAN_POINT('Ctrl Pts',(-0.236759334094774,-0.0141123582010645,
-0.0949314150996178));
#75966=CARTESIAN_POINT('Ctrl Pts',(-0.236842245196064,-0.0126448404025159,
-0.0950286449075528));
#75967=CARTESIAN_POINT('Ctrl Pts',(-0.237046527478915,-0.00831465553332598,
-0.0953141800904135));
#75968=CARTESIAN_POINT('Ctrl Pts',(-0.23712967786779,-0.0054503862617585,
-0.0955012980030014));
#75969=CARTESIAN_POINT('Ctrl Pts',(-0.237376655468488,0.0172067421768256,
-0.0969693134541154));
#75970=CARTESIAN_POINT('Ctrl Pts',(-0.235114231299932,0.0369476174326382,
-0.0981666877287926));
#75971=CARTESIAN_POINT('Ctrl Pts',(-0.228475771996707,0.0641759067051366,
-0.0998914917931622));
#75972=CARTESIAN_POINT('Ctrl Pts',(-0.226111375753752,0.072064906198731,
-0.100401685561311));
#75973=CARTESIAN_POINT('Ctrl Pts',(-0.221915157252005,0.0838070436925666,
-0.101198195648931));
#75974=CARTESIAN_POINT('Ctrl Pts',(-0.220381630715368,0.0877604072705071,
-0.101473017725974));
#75975=CARTESIAN_POINT('Ctrl Pts',(-0.218289092861059,0.0927536110717456,
-0.101831289357));
#75976=CARTESIAN_POINT('Ctrl Pts',(-0.217827049540407,0.0938335589011456,
-0.101909456485216));
#75977=CARTESIAN_POINT('Ctrl Pts',(-0.217068943362879,0.095569726766183,
-0.102036289503191));
#75978=CARTESIAN_POINT('Ctrl Pts',(-0.216777874180959,0.0962281251897154,
-0.10208466075129));
#75979=CARTESIAN_POINT('Ctrl Pts',(-0.216211674285649,0.097493263140531,
-0.102178153874216));
#75980=CARTESIAN_POINT('Ctrl Pts',(-0.215936979035774,0.0981001809090765,
-0.102223249815646));
#75981=CARTESIAN_POINT('Ctrl Pts',(-0.215323984791063,0.0994394944572594,
-0.102323297345094));
#75982=CARTESIAN_POINT('Ctrl Pts',(-0.214984498814626,0.100171336747408,
-0.102378319591914));
#75983=CARTESIAN_POINT('Ctrl Pts',(-0.21376578858428,0.102763822962466,
-0.102574451244748));
#75984=CARTESIAN_POINT('Ctrl Pts',(-0.212866119242487,0.104614675065719,
-0.102716716532706));
#75985=CARTESIAN_POINT('Ctrl Pts',(-0.205445213885111,0.119389250731872,
-0.10386912587332));
#75986=CARTESIAN_POINT('Ctrl Pts',(-0.197777874960259,0.131701813606501,
-0.104931439576513));
#75987=CARTESIAN_POINT('Ctrl Pts',(-0.183224240622791,0.150908902640768,
-0.106690099009823));
#75988=CARTESIAN_POINT('Ctrl Pts',(-0.176949469730423,0.158219882939297,
-0.107388731877561));
#75989=CARTESIAN_POINT('Ctrl Pts',(-0.164550925129815,0.171002670601748,
-0.108655484035029));
#75990=CARTESIAN_POINT('Ctrl Pts',(-0.158553968031887,0.176577425116427,
-0.109226722000924));
#75991=CARTESIAN_POINT('Ctrl Pts',(-0.150655810034008,0.183191966493385,
-0.109929483977509));
#75992=CARTESIAN_POINT('Ctrl Pts',(-0.149013265636112,0.184530530962521,
-0.110073129790207));
#75993=CARTESIAN_POINT('Ctrl Pts',(-0.146340408514578,0.186649766243898,
-0.110302956417574));
#75994=CARTESIAN_POINT('Ctrl Pts',(-0.145321298795663,0.187444313421689,
-0.110389688551851));
#75995=CARTESIAN_POINT('Ctrl Pts',(-0.143362477055389,0.18894592767337,
-0.110554717314766));
#75996=CARTESIAN_POINT('Ctrl Pts',(-0.14242390371116,0.189654409779722,
-0.11063306816178));
#75997=CARTESIAN_POINT('Ctrl Pts',(-0.140275849388458,0.191250929349737,
-0.110810772765256));
#75998=CARTESIAN_POINT('Ctrl Pts',(-0.139063124681192,0.192134534705682,
-0.110909952406068));
#75999=CARTESIAN_POINT('Ctrl Pts',(-0.135223831944562,0.194876493255582,
-0.111220438940319));
#76000=CARTESIAN_POINT('Ctrl Pts',(-0.132567716955189,0.196692995271332,
-0.111430151941891));
#76001=CARTESIAN_POINT('Ctrl Pts',(-0.117474710265588,0.206570347662989,
-0.112595452893011));
#76002=CARTESIAN_POINT('Ctrl Pts',(-0.10434021716574,0.213505990716383,
-0.113508436933499));
#76003=CARTESIAN_POINT('Ctrl Pts',(-0.0797631594554744,0.223670365562725,
-0.115138736986617));
#76004=CARTESIAN_POINT('Ctrl Pts',(-0.0685643471672252,0.227353212336554,
-0.115856262258257));
#76005=CARTESIAN_POINT('Ctrl Pts',(-0.0521091052626759,0.231437863805961,
-0.116930921805025));
#76006=CARTESIAN_POINT('Ctrl Pts',(-0.0470396628855004,0.232521191234172,
-0.117264799246147));
#76007=CARTESIAN_POINT('Ctrl Pts',(-0.0419392741328228,0.233437524640346,
-0.117607182502807));
#76008=CARTESIAN_POINT('',(0.150502666328431,-0.18330555925294,-0.04));
#76009=CARTESIAN_POINT('Origin',(0.,0.,-0.04));
#76010=CARTESIAN_POINT('',(-0.237174906472556,-0.000210629376151607,-0.0759410108039518));
#76011=CARTESIAN_POINT('Ctrl Pts',(-0.237174906472556,-0.000210629376151607,
-0.0759410108039518));
#76012=CARTESIAN_POINT('Ctrl Pts',(-0.237158621928716,-0.0185475073215331,
-0.0747111264345429));
#76013=CARTESIAN_POINT('Ctrl Pts',(-0.235011944072667,-0.0367877728492129,
-0.073481242065133));
#76014=CARTESIAN_POINT('Ctrl Pts',(-0.230823636693189,-0.0545199905422847,
-0.0722513576957233));
#76015=CARTESIAN_POINT('Ctrl Pts',(-0.23027479475933,-0.0568436463221744,
-0.0720901918464742));
#76016=CARTESIAN_POINT('Ctrl Pts',(-0.229690959325625,-0.0591586106164768,
-0.071929025997225));
#76017=CARTESIAN_POINT('Ctrl Pts',(-0.229072388495109,-0.0614639850168034,
-0.0717678601479759));
#76018=CARTESIAN_POINT('Ctrl Pts',(-0.225473876565801,-0.0748754116018108,
-0.0708302840410715));
#76019=CARTESIAN_POINT('Ctrl Pts',(-0.220679734069817,-0.0880206305498771,
-0.0698927079341669));
#76020=CARTESIAN_POINT('Ctrl Pts',(-0.214749523310849,-0.100670864021142,
-0.0689551318272628));
#76021=CARTESIAN_POINT('Ctrl Pts',(-0.208831413436207,-0.113295284073934,
-0.0680194688901394));
#76022=CARTESIAN_POINT('Ctrl Pts',(-0.201782122092558,-0.125425925126062,
-0.0670838059530158));
#76023=CARTESIAN_POINT('Ctrl Pts',(-0.193710062291085,-0.136851716803933,
-0.0661481430158926));
#76024=CARTESIAN_POINT('Ctrl Pts',(-0.185637996783948,-0.148277516558024,
-0.0652124794174042));
#76025=CARTESIAN_POINT('Ctrl Pts',(-0.176543608234863,-0.158997737682083,
-0.0642768158189159));
#76026=CARTESIAN_POINT('Ctrl Pts',(-0.166579315386946,-0.168829240092516,
-0.0633411522204277));
#76027=CARTESIAN_POINT('Ctrl Pts',(-0.156616017366152,-0.178659760933518,
-0.0624055820378537));
#76028=CARTESIAN_POINT('Ctrl Pts',(-0.145783612815802,-0.187601155783707,
-0.0614700118552792));
#76029=CARTESIAN_POINT('Ctrl Pts',(-0.134270399414448,-0.195508159589529,
-0.0605344416727052));
#76030=CARTESIAN_POINT('Ctrl Pts',(-0.122726310093654,-0.203436368249634,
-0.0595963624955889));
#76031=CARTESIAN_POINT('Ctrl Pts',(-0.110498503346432,-0.210324207770786,
-0.0586582833184732));
#76032=CARTESIAN_POINT('Ctrl Pts',(-0.0978025802286634,-0.216070904856753,
-0.0577202041413569));
#76033=CARTESIAN_POINT('Ctrl Pts',(-0.0895185622228277,-0.219820592192808,
-0.0571081127855693));
#76034=CARTESIAN_POINT('Ctrl Pts',(-0.0810357512357401,-0.223085405507269,
-0.0564960214297812));
#76035=CARTESIAN_POINT('Ctrl Pts',(-0.0724175090206001,-0.225848810074907,
-0.0558839300739935));
#76036=CARTESIAN_POINT('Ctrl Pts',(-0.058700685419742,-0.230247054176878,
-0.054909723391777));
#76037=CARTESIAN_POINT('Ctrl Pts',(-0.0445441512454388,-0.233403639176892,
-0.0539355167095605));
#76038=CARTESIAN_POINT('Ctrl Pts',(-0.0301891542800366,-0.235245819492836,
-0.0529613100273441));
#76039=CARTESIAN_POINT('Ctrl Pts',(-0.0158683657925657,-0.237083609826336,
-0.0519894249149523));
#76040=CARTESIAN_POINT('Ctrl Pts',(-0.00135080955263697,-0.237613054939815,
-0.0510175398025608));
#76041=CARTESIAN_POINT('Ctrl Pts',(0.0131117876559467,-0.236812292015143,
-0.0500456546901691));
#76042=CARTESIAN_POINT('Ctrl Pts',(0.0275557422064152,-0.236012561294384,
-0.0490750223625722));
#76043=CARTESIAN_POINT('Ctrl Pts',(0.0419441028805848,-0.233886027421871,
-0.0481043900349758));
#76044=CARTESIAN_POINT('Ctrl Pts',(0.056025401347839,-0.23046287125872,
-0.0471337577073792));
#76045=CARTESIAN_POINT('Ctrl Pts',(0.0700949748608359,-0.22704256542571,
-0.046163933587894));
#76046=CARTESIAN_POINT('Ctrl Pts',(0.0838572370641301,-0.222327955504268,
-0.0451941094684088));
#76047=CARTESIAN_POINT('Ctrl Pts',(0.0970721910482277,-0.216400023914269,
-0.0442242853489239));
#76048=CARTESIAN_POINT('Ctrl Pts',(0.110296407387627,-0.210467937439687,
-0.04325378148015));
#76049=CARTESIAN_POINT('Ctrl Pts',(0.122971840732214,-0.203321153059231,
-0.0422832776113755));
#76050=CARTESIAN_POINT('Ctrl Pts',(0.134879909857446,-0.195088160947422,
-0.0413127737426016));
#76051=CARTESIAN_POINT('Ctrl Pts',(0.140249148447719,-0.191375980702644,
-0.0408751824950676));
#76052=CARTESIAN_POINT('Ctrl Pts',(0.145462740656309,-0.187443580242826,
-0.0404375912475343));
#76053=CARTESIAN_POINT('Ctrl Pts',(0.150502666328431,-0.18330555925294,
-0.0400000000000005));
#76054=CARTESIAN_POINT('Ctrl Pts',(-0.237174906802781,-0.000210257205037135,
-0.0759349427062525));
#76055=CARTESIAN_POINT('Ctrl Pts',(-0.237184871465481,0.0110301088355765,
-0.0766243420965755));
#76056=CARTESIAN_POINT('Ctrl Pts',(-0.236395779708201,0.0222563389972307,
-0.0773177921882711));
#76057=CARTESIAN_POINT('Ctrl Pts',(-0.234160303454425,0.0379800345014828,
-0.0783290024312435));
#76058=CARTESIAN_POINT('Ctrl Pts',(-0.233372123243744,0.0425555912896126,
-0.0786279996175695));
#76059=CARTESIAN_POINT('Ctrl Pts',(-0.232138852293334,0.0486414640296778,
-0.0790334908787454));
#76060=CARTESIAN_POINT('Ctrl Pts',(-0.231812242696509,0.0501749211471305,
-0.0791363285688339));
#76061=CARTESIAN_POINT('Ctrl Pts',(-0.231151157611951,0.0531344351987663,
-0.0793361544101244));
#76062=CARTESIAN_POINT('Ctrl Pts',(-0.230818627185992,0.0545608564178603,
-0.0794330779268147));
#76063=CARTESIAN_POINT('Ctrl Pts',(-0.230192614039309,0.0571380010832394,
-0.0796093424027828));
#76064=CARTESIAN_POINT('Ctrl Pts',(-0.229903657821878,0.0582897826325445,
-0.0796885374281201));
#76065=CARTESIAN_POINT('Ctrl Pts',(-0.22926304781756,0.060764372255098,
-0.0798596117821293));
#76066=CARTESIAN_POINT('Ctrl Pts',(-0.228908569309991,0.0620863978056552,
-0.079951578523863));
#76067=CARTESIAN_POINT('Ctrl Pts',(-0.22791578960818,0.0656648475377874,
-0.0802021039836467));
#76068=CARTESIAN_POINT('Ctrl Pts',(-0.227255448984399,0.0679149437704475,
-0.0803613582399107));
#76069=CARTESIAN_POINT('Ctrl Pts',(-0.223314490021691,0.0806420971034408,
-0.0812722542829496));
#76070=CARTESIAN_POINT('Ctrl Pts',(-0.21934334157729,0.090889749731291,
-0.0820458021824909));
#76071=CARTESIAN_POINT('Ctrl Pts',(-0.209585964487055,0.111665367466873,
-0.0836949756063555));
#76072=CARTESIAN_POINT('Ctrl Pts',(-0.203680656515842,0.122104880727242,
-0.0845712972506596));
#76073=CARTESIAN_POINT('Ctrl Pts',(-0.192340692450215,0.139023187812856,
-0.086044737919071));
#76074=CARTESIAN_POINT('Ctrl Pts',(-0.187301726833644,0.145741140601818,
-0.0866455770107887));
#76075=CARTESIAN_POINT('Ctrl Pts',(-0.180822706082521,0.153486276444645,
-0.0873459029039126));
#76076=CARTESIAN_POINT('Ctrl Pts',(-0.179714534521033,0.154782345818205,
-0.0874633599572446));
#76077=CARTESIAN_POINT('Ctrl Pts',(-0.178024842028212,0.156715922302783,
-0.0876388503564303));
#76078=CARTESIAN_POINT('Ctrl Pts',(-0.177453690138022,0.157362360798179,
-0.0876975651350682));
#76079=CARTESIAN_POINT('Ctrl Pts',(-0.176431219120985,0.158506963088898,
-0.0878015841051318));
#76080=CARTESIAN_POINT('Ctrl Pts',(-0.175981287427686,0.159006348771741,
-0.0878469862438275));
#76081=CARTESIAN_POINT('Ctrl Pts',(-0.174995754780171,0.160090898153959,
-0.0879456209862042));
#76082=CARTESIAN_POINT('Ctrl Pts',(-0.174459333737651,0.160675296110486,
-0.0879987922362712));
#76083=CARTESIAN_POINT('Ctrl Pts',(-0.172930307121767,0.162324392126888,
-0.0881489377149598));
#76084=CARTESIAN_POINT('Ctrl Pts',(-0.171930797592166,0.16338268114712,
-0.0882454148530343));
#76085=CARTESIAN_POINT('Ctrl Pts',(-0.165292232081609,0.170283259705127,
-0.0888758498991717));
#76086=CARTESIAN_POINT('Ctrl Pts',(-0.159365443180029,0.175842531747045,
-0.0893902801404555));
#76087=CARTESIAN_POINT('Ctrl Pts',(-0.140071327184596,0.192161582258995,
-0.0909649355060656));
#76088=CARTESIAN_POINT('Ctrl Pts',(-0.125815890111833,0.201783142663815,
-0.0919949081816021));
#76089=CARTESIAN_POINT('Ctrl Pts',(-0.103740430807673,0.213426518917386,
-0.0935611549519308));
#76090=CARTESIAN_POINT('Ctrl Pts',(-0.0966585351981046,0.216725781169569,
-0.0940591087956679));
#76091=CARTESIAN_POINT('Ctrl Pts',(-0.087521784953452,0.220445346438063,
-0.0947033806385633));
#76092=CARTESIAN_POINT('Ctrl Pts',(-0.085606255171609,0.221196252788198,
-0.094838536730929));
#76093=CARTESIAN_POINT('Ctrl Pts',(-0.082453235290099,0.222385177215646,
-0.0950612662435626));
#76094=CARTESIAN_POINT('Ctrl Pts',(-0.0812214226796713,0.222838020624795,
-0.0951483451909119));
#76095=CARTESIAN_POINT('Ctrl Pts',(-0.078876005780729,0.223678220611693,
-0.095314298212735));
#76096=CARTESIAN_POINT('Ctrl Pts',(-0.0777631440224593,0.224067543409303,
-0.095393104370899));
#76097=CARTESIAN_POINT('Ctrl Pts',(-0.0752199078727373,0.224936038884836,
-0.0955733702939126));
#76098=CARTESIAN_POINT('Ctrl Pts',(-0.0737877840137135,0.225409890815699,
-0.0956750013880507));
#76099=CARTESIAN_POINT('Ctrl Pts',(-0.0693527254060101,0.226830540068804,
-0.095990165247697));
#76100=CARTESIAN_POINT('Ctrl Pts',(-0.0663354882016132,0.227731191929472,
-0.0962051840564345));
#76101=CARTESIAN_POINT('Ctrl Pts',(-0.0562535680305483,0.230523312114176,
-0.0969260105663089));
#76102=CARTESIAN_POINT('Ctrl Pts',(-0.0491251218842478,0.232146520123974,
-0.0974396283497645));
#76103=CARTESIAN_POINT('Ctrl Pts',(-0.0419392282806928,0.233437532878113,
-0.0979609479953583));
#76104=CARTESIAN_POINT('Origin',(3.51939854619125E-17,0.,-0.04));
#76105=CARTESIAN_POINT('',(-0.287838815064698,-0.060847814604559,-0.04));
#76106=CARTESIAN_POINT('Origin',(0.,0.,-0.04));
#76107=CARTESIAN_POINT('Ctrl Pts',(-0.287838815064696,-0.0608478146045586,
-0.0399999999999992));
#76108=CARTESIAN_POINT('Ctrl Pts',(-0.286283540210113,-0.0659045633072947,
-0.0399999999999988));
#76109=CARTESIAN_POINT('Ctrl Pts',(-0.284582373527586,-0.0709112958269072,
-0.0399999999999993));
#76110=CARTESIAN_POINT('Ctrl Pts',(-0.28273331426505,-0.0758621163637482,
-0.0399999999999997));
#76111=CARTESIAN_POINT('Ctrl Pts',(-0.278025520183387,-0.0884671442798089,
-0.0400000000000001));
#76112=CARTESIAN_POINT('Ctrl Pts',(-0.272360008650186,-0.100710598371884,
-0.0400000000000012));
#76113=CARTESIAN_POINT('Ctrl Pts',(-0.265818480752146,-0.112520517868452,
-0.0400000000000015));
#76114=CARTESIAN_POINT('Ctrl Pts',(-0.260688658964569,-0.121781776596889,
-0.0400000000000017));
#76115=CARTESIAN_POINT('Ctrl Pts',(-0.255013694239099,-0.130782755603393,
-0.0400000000000012));
#76116=CARTESIAN_POINT('Ctrl Pts',(-0.248864487923652,-0.139437457683636,
-0.0400000000000016));
#76117=CARTESIAN_POINT('Ctrl Pts',(-0.240894471708758,-0.150654859145894,
-0.0400000000000022));
#76118=CARTESIAN_POINT('Ctrl Pts',(-0.23212064683322,-0.161308101360409,
-0.0400000000000023));
#76119=CARTESIAN_POINT('Ctrl Pts',(-0.222626939812443,-0.171314385878302,
-0.0400000000000022));
#76120=CARTESIAN_POINT('Ctrl Pts',(-0.21832455164424,-0.175849065537495,
-0.0400000000000022));
#76121=CARTESIAN_POINT('Ctrl Pts',(-0.213872397622076,-0.180252249579648,
-0.0400000000000026));
#76122=CARTESIAN_POINT('Ctrl Pts',(-0.209283584109627,-0.184509529763357,
-0.0400000000000031));
#76123=CARTESIAN_POINT('Ctrl Pts',(-0.204476924871702,-0.188968916719908,
-0.0400000000000036));
#76124=CARTESIAN_POINT('Ctrl Pts',(-0.199527853480205,-0.193261361732437,
-0.0400000000000041));
#76125=CARTESIAN_POINT('Ctrl Pts',(-0.194449905572787,-0.197375579987002,
-0.0400000000000039));
#76126=CARTESIAN_POINT('Ctrl Pts',(-0.18165053109359,-0.207745796674809,
-0.0400000000000036));
#76127=CARTESIAN_POINT('Ctrl Pts',(-0.168024374394842,-0.216995232927637,
-0.0400000000000015));
#76128=CARTESIAN_POINT('Ctrl Pts',(-0.153712907451332,-0.224968312253503,
-0.0400000000000022));
#76129=CARTESIAN_POINT('Ctrl Pts',(-0.143239782181528,-0.230803008228101,
-0.0400000000000027));
#76130=CARTESIAN_POINT('Ctrl Pts',(-0.132399065183417,-0.235953385843509,
-0.0400000000000035));
#76131=CARTESIAN_POINT('Ctrl Pts',(-0.121243795560285,-0.240340769520388,
-0.0400000000000029));
#76132=CARTESIAN_POINT('Ctrl Pts',(-0.109335780392514,-0.245024209108684,
-0.0400000000000027));
#76133=CARTESIAN_POINT('Ctrl Pts',(-0.0971496399731909,-0.248806596857885,
-0.040000000000001));
#76134=CARTESIAN_POINT('Ctrl Pts',(-0.0847601082121804,-0.251609660970604,
-0.0400000000000014));
#76135=CARTESIAN_POINT('Ctrl Pts',(-0.0834902268297793,-0.25189696472018,
-0.0400000000000015));
#76136=CARTESIAN_POINT('Ctrl Pts',(-0.0822181843381618,-0.252173969867375,
-0.0400000000000012));
#76137=CARTESIAN_POINT('Ctrl Pts',(-0.0809440531687431,-0.252440581539771,
-0.0400000000000011));
#76138=CARTESIAN_POINT('Ctrl Pts',(-0.0684659059362601,-0.255051631156887,
-0.04));
#76139=CARTESIAN_POINT('Ctrl Pts',(-0.0557870915798686,-0.256667486014179,
-0.0399999999999995));
#76140=CARTESIAN_POINT('Ctrl Pts',(-0.0430126701052795,-0.257314032850501,
-0.0399999999999991));
#76141=CARTESIAN_POINT('Ctrl Pts',(-0.037129326557397,-0.257611804234156,
-0.0399999999999989));
#76142=CARTESIAN_POINT('Ctrl Pts',(-0.0312252572910126,-0.257703706671377,
-0.0399999999999976));
#76143=CARTESIAN_POINT('Ctrl Pts',(-0.0253118328480331,-0.257590874842292,
-0.039999999999998));
#76144=CARTESIAN_POINT('Ctrl Pts',(-0.0194836856989803,-0.257479670157198,
-0.0399999999999984));
#76145=CARTESIAN_POINT('Ctrl Pts',(-0.0136532337202037,-0.257169362129647,
-0.0399999999999976));
#76146=CARTESIAN_POINT('Ctrl Pts',(-0.00784763512537938,-0.256664290536718,
-0.0399999999999974));
#76147=CARTESIAN_POINT('Ctrl Pts',(0.00781580971746332,-0.255301612613277,
-0.0399999999999969));
#76148=CARTESIAN_POINT('Ctrl Pts',(0.0233323927142078,-0.252524616633121,
-0.0399999999999976));
#76149=CARTESIAN_POINT('Ctrl Pts',(0.0385007003554855,-0.248383008519942,
-0.0399999999999976));
#76150=CARTESIAN_POINT('Ctrl Pts',(0.0491632350559369,-0.245471672511548,
-0.0399999999999976));
#76151=CARTESIAN_POINT('Ctrl Pts',(0.059653511041483,-0.241884935280662,
-0.0399999999999978));
#76152=CARTESIAN_POINT('Ctrl Pts',(0.0698923366418034,-0.237627597582937,
-0.0399999999999982));
#76153=CARTESIAN_POINT('Ctrl Pts',(0.0737978347774825,-0.236003678484158,
-0.0399999999999983));
#76154=CARTESIAN_POINT('Ctrl Pts',(0.0776663307490886,-0.234281976313234,
-0.0399999999999973));
#76155=CARTESIAN_POINT('Ctrl Pts',(0.0814808838935122,-0.232468982961978,
-0.0399999999999975));
#76156=CARTESIAN_POINT('Ctrl Pts',(0.0948711124254617,-0.226104831151508,
-0.0399999999999976));
#76157=CARTESIAN_POINT('Ctrl Pts',(0.107640202715245,-0.218602145131227,
-0.0399999999999986));
#76158=CARTESIAN_POINT('Ctrl Pts',(0.119605438277537,-0.209989258535857,
-0.0399999999999986));
#76159=CARTESIAN_POINT('Ctrl Pts',(0.130647229961905,-0.202041090771666,
-0.0399999999999991));
#76160=CARTESIAN_POINT('Ctrl Pts',(0.141004945256145,-0.193146676236034,
-0.0399999999999997));
#76161=CARTESIAN_POINT('Ctrl Pts',(0.150502666328436,-0.183305559252936,
-0.0399999999999996));
#76162=CARTESIAN_POINT('',(0.22249458563984,0.0827040654021107,-0.0398874406537738));
#76163=CARTESIAN_POINT('Ctrl Pts',(0.223395701213113,0.0796639272475427,
-0.04));
#76164=CARTESIAN_POINT('Ctrl Pts',(0.2230414864133,0.0806572257995756,-0.0399624802179247));
#76165=CARTESIAN_POINT('Ctrl Pts',(0.222680646665404,0.081648161864277,
-0.039924960435849));
#76166=CARTESIAN_POINT('Ctrl Pts',(0.222313214070923,0.0826366472847004,
-0.0398874406537737));
#76167=CARTESIAN_POINT('Ctrl Pts',(0.222674980869761,0.0827832056464219,
-0.0400000000000007));
#76168=CARTESIAN_POINT('Ctrl Pts',(0.221331052085945,0.0884148732654746,
-0.0400000000000008));
#76169=CARTESIAN_POINT('Ctrl Pts',(0.219769833377309,0.0939831708252383,
-0.0400000000000001));
#76170=CARTESIAN_POINT('Ctrl Pts',(0.217990451664176,0.099475512510641,
-0.04));
#76171=CARTESIAN_POINT('Ctrl Pts',(0.214256976699871,0.110999470538598,
-0.0399999999999994));
#76172=CARTESIAN_POINT('Ctrl Pts',(0.209564791763102,0.122189312126664,
-0.0400000000000003));
#76173=CARTESIAN_POINT('Ctrl Pts',(0.204016432957559,0.132986817060258,
-0.0399999999999988));
#76174=CARTESIAN_POINT('Ctrl Pts',(0.200496467614902,0.139836922557307,
-0.0399999999999993));
#76175=CARTESIAN_POINT('Ctrl Pts',(0.196628495701105,0.146532151765652,
-0.0399999999999984));
#76176=CARTESIAN_POINT('Ctrl Pts',(0.19245580578463,0.153026708431451,-0.039999999999998));
#76177=CARTESIAN_POINT('Ctrl Pts',(0.186915308542496,0.161650180104644,
-0.0399999999999974));
#76178=CARTESIAN_POINT('Ctrl Pts',(0.180832662499186,0.169931866194158,
-0.0399999999999965));
#76179=CARTESIAN_POINT('Ctrl Pts',(0.174264480746233,0.177837483950101,
-0.0399999999999971));
#76180=CARTESIAN_POINT('Ctrl Pts',(0.16975483858615,0.183265395124708,-0.0399999999999975));
#76181=CARTESIAN_POINT('Ctrl Pts',(0.165014946191758,0.188517133640017,
-0.0399999999999955));
#76182=CARTESIAN_POINT('Ctrl Pts',(0.160064174348171,0.193576884039022,
-0.0399999999999964));
#76183=CARTESIAN_POINT('Ctrl Pts',(0.156162208776054,0.197564741384135,
-0.0399999999999971));
#76184=CARTESIAN_POINT('Ctrl Pts',(0.152134390718043,0.201427900135178,
-0.0399999999999966));
#76185=CARTESIAN_POINT('Ctrl Pts',(0.147995497593573,0.205155973605731,
-0.0399999999999967));
#76186=CARTESIAN_POINT('Ctrl Pts',(0.136081349924499,0.215887542774968,
-0.0399999999999971));
#76187=CARTESIAN_POINT('Ctrl Pts',(0.123234372878606,0.225517729201755,
-0.0399999999999972));
#76188=CARTESIAN_POINT('Ctrl Pts',(0.109642260298283,0.233917545345877,
-0.0399999999999972));
#76189=CARTESIAN_POINT('Ctrl Pts',(0.100917414355191,0.239309429894705,
-0.0399999999999972));
#76190=CARTESIAN_POINT('Ctrl Pts',(0.09188516178185,0.24419367893778,-0.0399999999999965));
#76191=CARTESIAN_POINT('Ctrl Pts',(0.0825842917960279,0.248529743097262,
-0.0399999999999971));
#76192=CARTESIAN_POINT('Ctrl Pts',(0.0772852871455863,0.251000138251773,
-0.0399999999999974));
#76193=CARTESIAN_POINT('Ctrl Pts',(0.0719034015557044,0.253289849721424,
-0.0399999999999972));
#76194=CARTESIAN_POINT('Ctrl Pts',(0.0664655282955866,0.255384798311809,
-0.0399999999999977));
#76195=CARTESIAN_POINT('Ctrl Pts',(0.0572749031145685,0.258925500043301,
-0.0399999999999985));
#76196=CARTESIAN_POINT('Ctrl Pts',(0.0479118585129067,0.261916421959981,
-0.0399999999999984));
#76197=CARTESIAN_POINT('Ctrl Pts',(0.0384166442040826,0.264327757183461,
-0.0399999999999985));
#76198=CARTESIAN_POINT('Ctrl Pts',(0.0229887101002665,0.268245722562663,
-0.0399999999999994));
#76199=CARTESIAN_POINT('Ctrl Pts',(0.00721254038154319,0.270636624867907,
-0.0399999999999979));
#76200=CARTESIAN_POINT('Ctrl Pts',(-0.0087328601544421,0.271586817233884,
-0.0400000000000007));
#76201=CARTESIAN_POINT('Ctrl Pts',(-0.0117870319733156,0.271768816471854,
-0.0400000000000012));
#76202=CARTESIAN_POINT('Ctrl Pts',(-0.0148474612088789,0.271897813973021,
-0.0400000000000012));
#76203=CARTESIAN_POINT('Ctrl Pts',(-0.017912944060836,0.271974210463001,
-0.0400000000000013));
#76204=CARTESIAN_POINT('Ctrl Pts',(-0.023389560269392,0.2721106960594,-0.0400000000000013));
#76205=CARTESIAN_POINT('Ctrl Pts',(-0.0288790425251526,0.272078878082152,
-0.0400000000000002));
#76206=CARTESIAN_POINT('Ctrl Pts',(-0.034355927104671,0.271882901390066,
-0.0400000000000005));
#76207=CARTESIAN_POINT('Ctrl Pts',(-0.0515834758169103,0.271266456409283,
-0.0400000000000017));
#76208=CARTESIAN_POINT('Ctrl Pts',(-0.0687348278204772,0.269032047713159,
-0.0400000000000022));
#76209=CARTESIAN_POINT('Ctrl Pts',(-0.0855927959851901,0.265288603456289,
-0.0400000000000021));
#76210=CARTESIAN_POINT('Ctrl Pts',(-0.0939029519891339,0.263443268036106,
-0.040000000000002));
#76211=CARTESIAN_POINT('Ctrl Pts',(-0.102142100636434,0.261230327336921,
-0.0400000000000021));
#76212=CARTESIAN_POINT('Ctrl Pts',(-0.110284812020322,0.258657679335378,
-0.0400000000000021));
#76213=CARTESIAN_POINT('Ctrl Pts',(-0.11652245142853,0.256686929077716,
-0.040000000000002));
#76214=CARTESIAN_POINT('Ctrl Pts',(-0.122706184972723,0.254503953011045,
-0.0400000000000007));
#76215=CARTESIAN_POINT('Ctrl Pts',(-0.128815207409699,0.252114660253398,
-0.0400000000000013));
#76216=CARTESIAN_POINT('Ctrl Pts',(-0.135399388890598,0.24953952858714,
-0.0400000000000019));
#76217=CARTESIAN_POINT('Ctrl Pts',(-0.141881668799996,0.246730834774574,
-0.0400000000000011));
#76218=CARTESIAN_POINT('Ctrl Pts',(-0.148245421000419,0.243696854595293,
-0.0400000000000011));
#76219=CARTESIAN_POINT('Ctrl Pts',(-0.16393852661808,0.236215015281659,
-0.0400000000000013));
#76220=CARTESIAN_POINT('Ctrl Pts',(-0.178918800966714,0.227363679838949,
-0.0399999999999997));
#76221=CARTESIAN_POINT('Ctrl Pts',(-0.192978433199048,0.217213213525256,
-0.0399999999999996));
#76222=CARTESIAN_POINT('Ctrl Pts',(-0.203047642906921,0.209943665342464,
-0.0399999999999995));
#76223=CARTESIAN_POINT('Ctrl Pts',(-0.212644773119861,0.202006682473912,
-0.0399999999999999));
#76224=CARTESIAN_POINT('Ctrl Pts',(-0.221686865784453,0.193412961144454,
-0.04));
#76225=CARTESIAN_POINT('Ctrl Pts',(-0.103676804647749,0.212843510916694,
-1.99397142723206));
#76226=CARTESIAN_POINT('Ctrl Pts',(-0.174500313671441,0.178346644274193,
-1.98867562368504));
#76227=CARTESIAN_POINT('Ctrl Pts',(-0.277757662224097,0.0337041756151036,
-1.97808517678002));
#76228=CARTESIAN_POINT('Ctrl Pts',(-0.178659324738769,-0.215666118176939,
-1.96220008651701));
#76229=CARTESIAN_POINT('Ctrl Pts',(0.0843322378632243,-0.266777789429326,
-1.94631615644302));
#76230=CARTESIAN_POINT('Ctrl Pts',(0.269948356849218,-0.0738434778211555,
-1.93043222636904));
#76231=CARTESIAN_POINT('Ctrl Pts',(0.208339268208791,0.18691124507345,-1.91454829629505));
#76232=CARTESIAN_POINT('Ctrl Pts',(-0.0441543487728196,0.276352467078339,
-1.89866436622106));
#76233=CARTESIAN_POINT('Ctrl Pts',(-0.256182511614628,0.112686240256283,
-1.88278043614707));
#76234=CARTESIAN_POINT('Ctrl Pts',(-0.233541289554458,-0.154232428936108,
-1.86689650607308));
#76235=CARTESIAN_POINT('Ctrl Pts',(0.00304250668361687,-0.279851820056704,
-1.8510125759991));
#76236=CARTESIAN_POINT('Ctrl Pts',(0.236836682863679,-0.149117080380604,
-1.8351286459251));
#76237=CARTESIAN_POINT('Ctrl Pts',(0.253675595533036,0.118221431597056,
-1.81924471585112));
#76238=CARTESIAN_POINT('Ctrl Pts',(0.0381317971162815,0.277260151070568,
-1.80336078577713));
#76239=CARTESIAN_POINT('Ctrl Pts',(-0.212342650053903,0.182312969274217,
-1.78747685570314));
#76240=CARTESIAN_POINT('Ctrl Pts',(-0.268298711511727,-0.0796443191042248,
-1.77159292562915));
#76241=CARTESIAN_POINT('Ctrl Pts',(-0.0784770000832964,-0.268642374478244,
-1.75570899555517));
#76242=CARTESIAN_POINT('Ctrl Pts',(0.183234287828566,-0.21154808143558,
-1.73982506548118));
#76243=CARTESIAN_POINT('Ctrl Pts',(0.277092030570221,0.0393369872510852,
-1.72394113540719));
#76244=CARTESIAN_POINT('Ctrl Pts',(0.117116878322258,0.254186982850244,
-1.7080572053332));
#76245=CARTESIAN_POINT('Ctrl Pts',(-0.150144335198661,0.236186512280278,
-1.69217327525921));
#76246=CARTESIAN_POINT('Ctrl Pts',(-0.279864357098656,0.00182505268549074,
-1.67628934518523));
#76247=CARTESIAN_POINT('Ctrl Pts',(-0.153211879123455,-0.234208258795446,
-1.66040541511124));
#76248=CARTESIAN_POINT('Ctrl Pts',(0.113791847079068,-0.255692793405017,
-1.64452148503725));
#76249=CARTESIAN_POINT('Ctrl Pts',(0.27655543274757,-0.0429474273786092,
-1.62863755496326));
#76250=CARTESIAN_POINT('Ctrl Pts',(0.185977692986568,0.209140351247083,
-1.61275362488927));
#76251=CARTESIAN_POINT('Ctrl Pts',(-0.0749667420769754,0.269643053845345,
-1.59686969481528));
#76252=CARTESIAN_POINT('Ctrl Pts',(-0.26723715555904,0.0831365837885122,
-1.5809857647413));
#76253=CARTESIAN_POINT('Ctrl Pts',(-0.214702343360205,-0.179527971695799,
-1.56510183466731));
#76254=CARTESIAN_POINT('Ctrl Pts',(0.0345126628622819,-0.277734162431102,
-1.54921790459332));
#76255=CARTESIAN_POINT('Ctrl Pts',(0.252112004718534,-0.121519241072826,
-1.53333397451933));
#76256=CARTESIAN_POINT('Ctrl Pts',(0.238761664170276,0.146014576655516,
-1.51745004444534));
#76257=CARTESIAN_POINT('Ctrl Pts',(0.00669135203703449,0.279790304841033,
-1.50156611437136));
#76258=CARTESIAN_POINT('Ctrl Pts',(-0.231508638966162,0.157261371475424,
-1.48568218429737));
#76259=CARTESIAN_POINT('Ctrl Pts',(-0.257632863479559,-0.109328388488873,
-1.46979825422338));
#76260=CARTESIAN_POINT('Ctrl Pts',(-0.0477499686083177,-0.275766802520549,
-1.45391432414939));
#76261=CARTESIAN_POINT('Ctrl Pts',(0.205874754808538,-0.189586323892037,
-1.4380303940754));
#76262=CARTESIAN_POINT('Ctrl Pts',(0.270905883525229,0.0702665720367265,
-1.42214646400142));
#76263=CARTESIAN_POINT('Ctrl Pts',(0.0877710122536518,0.265751083313652,
-1.40626253392743));
#76264=CARTESIAN_POINT('Ctrl Pts',(-0.175767358353134,0.217791700052944,
-1.39037860385344));
#76265=CARTESIAN_POINT('Ctrl Pts',(-0.278292311003068,-0.0296779128471706,
-1.37449467377945));
#76266=CARTESIAN_POINT('Ctrl Pts',(-0.125884854100124,-0.249960781689022,
-1.35861074370546));
#76267=CARTESIAN_POINT('Ctrl Pts',(0.141840661955398,-0.241264617153963,
-1.34272681363148));
#76268=CARTESIAN_POINT('Ctrl Pts',(0.27963164408674,-0.0115556263240567,
-1.32684288355749));
#76269=CARTESIAN_POINT('Ctrl Pts',(0.161263307416486,0.228739009693342,
-1.3109589534835));
#76270=CARTESIAN_POINT('Ctrl Pts',(-0.10483186864783,0.259495025366958,
-1.29507502340951));
#76271=CARTESIAN_POINT('Ctrl Pts',(-0.274894780018969,0.0525380699371205,
-1.27919109333552));
#76272=CARTESIAN_POINT('Ctrl Pts',(-0.193137623522783,-0.202546901369451,
-1.26330716326153));
#76273=CARTESIAN_POINT('Ctrl Pts',(0.0655451532412157,-0.272086790860894,
-1.24742323318755));
#76274=CARTESIAN_POINT('Ctrl Pts',(0.264184647493857,-0.0923788985804749,
-1.23153930311356));
#76275=CARTESIAN_POINT('Ctrl Pts',(0.220815196153506,0.171953592640814,
-1.21565537303957));
#76276=CARTESIAN_POINT('Ctrl Pts',(-0.0248341881767495,0.278766303508864,
-1.19977144296558));
#76277=CARTESIAN_POINT('Ctrl Pts',(-0.247733970089428,0.130212399325583,
-1.18388751289159));
#76278=CARTESIAN_POINT('Ctrl Pts',(-0.24369461130014,-0.137623854391846,
-1.16800358281761));
#76279=CARTESIAN_POINT('Ctrl Pts',(-0.0164164061701999,-0.279388422241956,
-1.15211965274362));
#76280=CARTESIAN_POINT('Ctrl Pts',(0.225900209349461,-0.165216477054391,
-1.13623572266963));
#76281=CARTESIAN_POINT('Ctrl Pts',(0.261278715510704,0.10030364746843,-1.12035179259564));
#76282=CARTESIAN_POINT('Ctrl Pts',(0.0573102836629663,0.273939628861662,
-1.10446786252165));
#76283=CARTESIAN_POINT('Ctrl Pts',(-0.199157797397855,0.196630518002749,
-1.08858393244767));
#76284=CARTESIAN_POINT('Ctrl Pts',(-0.273185418681399,-0.0608039134781932,
-1.07270000237368));
#76285=CARTESIAN_POINT('Ctrl Pts',(-0.0969588493689412,-0.262538321780736,
-1.05681607229969));
#76286=CARTESIAN_POINT('Ctrl Pts',(0.168087827865316,-0.223771917357639,
-1.0409321422257));
#76287=CARTESIAN_POINT('Ctrl Pts',(0.279155996603362,0.019982953604956,
-1.02504821215171));
#76288=CARTESIAN_POINT('Ctrl Pts',(0.134500568096756,0.245432243309726,
-1.00916428207772));
#76289=CARTESIAN_POINT('Ctrl Pts',(-0.133365429137207,0.246050911775273,
-0.993280352003735));
#76290=CARTESIAN_POINT('Ctrl Pts',(-0.279060712856098,0.0212722216667855,
-0.977396421929748));
#76291=CARTESIAN_POINT('Ctrl Pts',(-0.169119684944492,-0.2229930963924,
-0.961512491855758));
#76292=CARTESIAN_POINT('Ctrl Pts',(0.0957450942929234,-0.262983394519946,
-0.945628561781772));
#76293=CARTESIAN_POINT('Ctrl Pts',(0.272901637887803,-0.062065166660125,
-0.929744631707783));
#76294=CARTESIAN_POINT('Ctrl Pts',(0.200063951074714,0.195708467764605,
-0.913860701633795));
#76295=CARTESIAN_POINT('Ctrl Pts',(-0.0560442865067918,0.274201434759812,
-0.897976771559806));
#76296=CARTESIAN_POINT('Ctrl Pts',(-0.260812604026003,0.101509479634023,
-0.88209284148582));
#76297=CARTESIAN_POINT('Ctrl Pts',(-0.226660969547766,-0.164171233040571,
-0.86620891141183));
#76298=CARTESIAN_POINT('Ctrl Pts',(0.0151256761535035,-0.279461272442701,
-0.850324981337842));
#76299=CARTESIAN_POINT('Ctrl Pts',(0.243056297396063,-0.138748063664006,
-0.834441051263854));
#76300=CARTESIAN_POINT('Ctrl Pts',(0.248332806030034,0.129066673946625,
-0.818557121189867));
#76301=CARTESIAN_POINT('Ctrl Pts',(0.0261216044068271,0.27864861502905,
-0.802673191115877));
#76302=CARTESIAN_POINT('Ctrl Pts',(-0.220018549938132,0.172971750749988,
-0.786789261041891));
#76303=CARTESIAN_POINT('Ctrl Pts',(-0.264608546896811,-0.0911575876356607,
-0.770905330967901));
#76304=CARTESIAN_POINT('Ctrl Pts',(-0.0668012810437667,-0.271781120987654,
-0.755021400893914));
#76305=CARTESIAN_POINT('Ctrl Pts',(0.192199955552935,-0.203436884462588,
-0.739137470819925));
#76306=CARTESIAN_POINT('Ctrl Pts',(0.275134531851118,0.0512677116464285,
-0.723253540745937));
#76307=CARTESIAN_POINT('Ctrl Pts',(0.106029413257268,0.259008016089684,
-0.70736961067195));
#76308=CARTESIAN_POINT('Ctrl Pts',(-0.160204992551617,0.229481479069509,
-0.69148568059796));
#76309=CARTESIAN_POINT('Ctrl Pts',(-0.279682038710943,-0.0102638246714771,
-0.675601750523973));
#76310=CARTESIAN_POINT('Ctrl Pts',(-0.142953601577338,-0.240606850838584,
-0.659717820449986));
#76311=CARTESIAN_POINT('Ctrl Pts',(0.124728888771074,-0.25053960401566,
-0.643833890375996));
#76312=CARTESIAN_POINT('Ctrl Pts',(0.278152253379934,-0.0309630879286156,
-0.627949960302009));
#76313=CARTESIAN_POINT('Ctrl Pts',(0.176771509599478,0.216977469494643,
-0.612066030228021));
#76314=CARTESIAN_POINT('Ctrl Pts',(-0.0865425147664667,0.266153681192405,
-0.596182100154032));
#76315=CARTESIAN_POINT('Ctrl Pts',(-0.270578417007657,0.071517194604748,
-0.580298170080044));
#76316=CARTESIAN_POINT('Ctrl Pts',(-0.206748298185121,-0.188633321743026,
-0.564414240006056));
#76317=CARTESIAN_POINT('Ctrl Pts',(0.0464756333408657,-0.275984427785086,
-0.548530309932067));
#76318=CARTESIAN_POINT('Ctrl Pts',(0.25712510368365,-0.110517283403066,
-0.53264637985808));
#76319=CARTESIAN_POINT('Ctrl Pts',(0.232232592993323,0.156190305796638,
-0.516762449784092));
#76320=CARTESIAN_POINT('Ctrl Pts',(-0.00539886938617793,0.279818228647572,
-0.500878519710104));
#76321=CARTESIAN_POINT('Ctrl Pts',(-0.238084644363667,0.147115910075619,
-0.484994589636116));
#76322=CARTESIAN_POINT('Ctrl Pts',(-0.25267063837447,-0.1203533853658,-0.469110659562128));
#76323=CARTESIAN_POINT('Ctrl Pts',(-0.0357952081938611,-0.277571778006463,
-0.453226729488138));
#76324=CARTESIAN_POINT('Ctrl Pts',(0.21387077475615,-0.180517812444876,
-0.437342799414151));
#76325=CARTESIAN_POINT('Ctrl Pts',(0.267618330028949,0.0819012713019475,
-0.421458869340163));
#76326=CARTESIAN_POINT('Ctrl Pts',(0.0762114814842632,0.269293889627319,
-0.405574939266175));
#76327=CARTESIAN_POINT('Ctrl Pts',(-0.185009645352496,0.20999719090376,
-0.389691009192186));
#76328=CARTESIAN_POINT('Ctrl Pts',(-0.276750864670533,-0.0416695007967132,
-0.373807079118198));
#76329=CARTESIAN_POINT('Ctrl Pts',(-0.114971734614638,-0.255164436062807,
-0.357923149044211));
#76330=CARTESIAN_POINT('Ctrl Pts',(0.152128390037859,-0.234913479646994,
-0.342039218970221));
#76331=CARTESIAN_POINT('Ctrl Pts',(0.279869794930341,0.000532281982961198,
-0.326155288896234));
#76332=CARTESIAN_POINT('Ctrl Pts',(0.151233742192331,0.235490439708333,
-0.310271358822245));
#76333=CARTESIAN_POINT('Ctrl Pts',(-0.115941509278813,0.254725266554512,
-0.294387428748259));
#76334=CARTESIAN_POINT('Ctrl Pts',(-0.276907321688116,0.0406165003772714,
-0.27850349867427));
#76335=CARTESIAN_POINT('Ctrl Pts',(-0.184209608056035,-0.210699398348146,
-0.262619568600281));
#76336=CARTESIAN_POINT('Ctrl Pts',(0.0772354167140077,-0.269002063565523,
-0.246735638526293));
#76337=CARTESIAN_POINT('Ctrl Pts',(0.267927629451405,-0.0808826971579307,
-0.230851708452305));
#76338=CARTESIAN_POINT('Ctrl Pts',(0.213183148962925,0.18132997451097,-0.214967778378317));
#76339=CARTESIAN_POINT('Ctrl Pts',(-0.0368518537260703,0.277433701788479,
-0.199083848304329));
#76340=CARTESIAN_POINT('Ctrl Pts',(-0.253124531452511,0.119391245964334,
-0.183199918230341));
#76341=CARTESIAN_POINT('Ctrl Pts',(-0.237527290585313,-0.148020141499362,
-0.167315988156352));
#76342=CARTESIAN_POINT('Ctrl Pts',(-0.00432689865297213,-0.279837356241662,
-0.151432058082364));
#76343=CARTESIAN_POINT('Ctrl Pts',(0.232810568914152,-0.155304641198214,
-0.135548128008376));
#76344=CARTESIAN_POINT('Ctrl Pts',(0.256730473028442,0.111492279693591,
-0.119664197934388));
#76345=CARTESIAN_POINT('Ctrl Pts',(0.0453727461737449,0.276163517661131,
-0.1037802678604));
#76346=CARTESIAN_POINT('Ctrl Pts',(-0.207363196613034,0.187837216669757,
-0.0878963377864122));
#76347=CARTESIAN_POINT('Ctrl Pts',(-0.270500560251008,-0.0725291372450606,
-0.0720124077124241));
#76348=CARTESIAN_POINT('Ctrl Pts',(-0.0850981096593689,-0.266552231679603,
-0.0561258829081893));
#76349=CARTESIAN_POINT('Ctrl Pts',(0.0894476313883584,-0.232940382224155,
-0.0455340014619504));
#76350=CARTESIAN_POINT('Ctrl Pts',(0.150323359639724,-0.182904692841898,
-0.0402367633737074));
#76351=CARTESIAN_POINT('Ctrl Pts',(-0.112118529268456,0.230173966967767,
-1.98284177580134));
#76352=CARTESIAN_POINT('Ctrl Pts',(-0.188708733763536,0.192868245929506,
-1.97754597225432));
#76353=CARTESIAN_POINT('Ctrl Pts',(-0.300373653368441,0.0364484863611533,
-1.9669555253493));
#76354=CARTESIAN_POINT('Ctrl Pts',(-0.193206385920782,-0.233226400690007,
-1.95107043508629));
#76355=CARTESIAN_POINT('Ctrl Pts',(0.0911988608374564,-0.288499761291163,
-1.9351865050123));
#76356=CARTESIAN_POINT('Ctrl Pts',(0.291928487294752,-0.0798560696146595,
-1.91930257493831));
#76357=CARTESIAN_POINT('Ctrl Pts',(0.225302973213726,0.202130206197729,
-1.90341864486432));
#76358=CARTESIAN_POINT('Ctrl Pts',(-0.0477495488217895,0.298854042365646,
-1.88753471479033));
#76359=CARTESIAN_POINT('Ctrl Pts',(-0.277041779249657,0.121861544337256,
-1.87165078471634));
#76360=CARTESIAN_POINT('Ctrl Pts',(-0.252557030449273,-0.166790567635357,
-1.85576685464236));
#76361=CARTESIAN_POINT('Ctrl Pts',(0.00329023811850059,-0.302638324786948,
-1.83988292456837));
#76362=CARTESIAN_POINT('Ctrl Pts',(0.256120746098554,-0.16125870967844,
-1.82399899449438));
#76363=CARTESIAN_POINT('Ctrl Pts',(0.274330741375541,0.127847430133554,
-1.80811506442039));
#76364=CARTESIAN_POINT('Ctrl Pts',(0.041236620144366,0.299835633133174,
-1.7922311343464));
#76365=CARTESIAN_POINT('Ctrl Pts',(-0.229632324278302,0.197157522852288,
-1.77634720427242));
#76366=CARTESIAN_POINT('Ctrl Pts',(-0.29014452211872,-0.0861292354918946,
-1.76046327419843));
#76367=CARTESIAN_POINT('Ctrl Pts',(-0.0848668693121321,-0.290516167314583,
-1.74457934412444));
#76368=CARTESIAN_POINT('Ctrl Pts',(0.198153858355219,-0.228773059130311,
-1.72869541405045));
#76369=CARTESIAN_POINT('Ctrl Pts',(0.29965382367924,0.0425399410352991,
-1.71281148397646));
#76370=CARTESIAN_POINT('Ctrl Pts',(0.126652940304422,0.274883767619805,
-1.69692755390248));
#76371=CARTESIAN_POINT('Ctrl Pts',(-0.162369607142684,0.255417636373752,
-1.68104362382849));
#76372=CARTESIAN_POINT('Ctrl Pts',(-0.302651882638292,0.00197365479800523,
-1.6651596937545));
#76373=CARTESIAN_POINT('Ctrl Pts',(-0.165686921121286,-0.253278306636561,
-1.64927576368051));
#76374=CARTESIAN_POINT('Ctrl Pts',(0.123057173497901,-0.276512186486802,
-1.63339183360652));
#76375=CARTESIAN_POINT('Ctrl Pts',(0.299073534202835,-0.0464443557063105,
-1.61750790353254));
#76376=CARTESIAN_POINT('Ctrl Pts',(0.201120641065663,0.226169283208327,
-1.60162397345855));
#76377=CARTESIAN_POINT('Ctrl Pts',(-0.081070793937711,0.291598325462588,
-1.58574004338456));
#76378=CARTESIAN_POINT('Ctrl Pts',(-0.288996530602623,0.0899058524656643,
-1.56985611331057));
#76379=CARTESIAN_POINT('Ctrl Pts',(-0.232184151988719,-0.194145761122461,
-1.55397218323658));
#76380=CARTESIAN_POINT('Ctrl Pts',(0.0373228034409807,-0.300348240140887,
-1.5380882531626));
#76381=CARTESIAN_POINT('Ctrl Pts',(0.27263983757989,-0.131413758682043,
-1.52220432308861));
#76382=CARTESIAN_POINT('Ctrl Pts',(0.258202466052199,0.157903589351488,
-1.50632039301462));
#76383=CARTESIAN_POINT('Ctrl Pts',(0.00723618510195202,0.302571800789299,
-1.49043646294063));
#76384=CARTESIAN_POINT('Ctrl Pts',(-0.250358874407996,0.170066137169941,
-1.47455253286664));
#76385=CARTESIAN_POINT('Ctrl Pts',(-0.278610223788148,-0.118230284645726,
-1.45866860279265));
#76386=CARTESIAN_POINT('Ctrl Pts',(-0.0516379364812537,-0.298220690970535,
-1.44278467271867));
#76387=CARTESIAN_POINT('Ctrl Pts',(0.222637790594162,-0.205023099201488,
-1.42690074264468));
#76388=CARTESIAN_POINT('Ctrl Pts',(0.292963979110057,0.075987919769137,
-1.41101681257069));
#76389=CARTESIAN_POINT('Ctrl Pts',(0.094917632152324,0.287389457206547,
-1.3951328824967));
#76390=CARTESIAN_POINT('Ctrl Pts',(-0.190078945612864,0.235525054806396,
-1.37924895242271));
#76391=CARTESIAN_POINT('Ctrl Pts',(-0.300951835103278,-0.0320943913297411,
-1.36336502234873));
#76392=CARTESIAN_POINT('Ctrl Pts',(-0.136134835046605,-0.270313454518445,
-1.34748109227474));
#76393=CARTESIAN_POINT('Ctrl Pts',(0.15338982005604,-0.260909218139248,
-1.33159716220075));
#76394=CARTESIAN_POINT('Ctrl Pts',(0.302400221326715,-0.0124965254536081,
-1.31571323212676));
#76395=CARTESIAN_POINT('Ctrl Pts',(0.174393924599955,0.247363732324456,
-1.29982930205277));
#76396=CARTESIAN_POINT('Ctrl Pts',(-0.113367642581119,0.280624009347843,
-1.28394537197879));
#76397=CARTESIAN_POINT('Ctrl Pts',(-0.297277665375771,0.0568159016085323,
-1.2680614419048));
#76398=CARTESIAN_POINT('Ctrl Pts',(-0.208863557951579,-0.21903897179878,
-1.25217751183081));
#76399=CARTESIAN_POINT('Ctrl Pts',(0.0708820666980315,-0.294241040012223,
-1.23629358175682));
#76400=CARTESIAN_POINT('Ctrl Pts',(0.285695476755416,-0.0999007085478101,
-1.22040965168283));
#76401=CARTESIAN_POINT('Ctrl Pts',(0.23879473443431,0.18595464988353,-1.20452572160884));
#76402=CARTESIAN_POINT('Ctrl Pts',(-0.0268562738156637,0.301464421721033,
-1.18864179153486));
#76403=CARTESIAN_POINT('Ctrl Pts',(-0.267905328203665,0.140814743997017,
-1.17275786146087));
#76404=CARTESIAN_POINT('Ctrl Pts',(-0.263537070827475,-0.148829665411615,
-1.15687393138688));
#76405=CARTESIAN_POINT('Ctrl Pts',(-0.0177530868349023,-0.302137195516692,
-1.14099000131289));
#76406=CARTESIAN_POINT('Ctrl Pts',(0.244293787021608,-0.178668975005457,
-1.1251060712389));
#76407=CARTESIAN_POINT('Ctrl Pts',(0.282552933722652,0.108470717945358,
-1.10922214116491));
#76408=CARTESIAN_POINT('Ctrl Pts',(0.0619766855091786,0.296244742502134,
-1.09333821109093));
#76409=CARTESIAN_POINT('Ctrl Pts',(-0.215373915240332,0.212640856001168,
-1.07745428101694));
#76410=CARTESIAN_POINT('Ctrl Pts',(-0.295429121916048,-0.0657547787675702,
-1.06157035094295));
#76411=CARTESIAN_POINT('Ctrl Pts',(-0.104853574796624,-0.283915101499071,
-1.04568642086896));
#76412=CARTESIAN_POINT('Ctrl Pts',(0.181774121147142,-0.241992202122388,
-1.02980249079498));
#76413=CARTESIAN_POINT('Ctrl Pts',(0.30188584497737,0.0216100349180264,
-1.01391856072098));
#76414=CARTESIAN_POINT('Ctrl Pts',(0.145452070325817,0.265416186855271,
-0.998034630647006));
#76415=CARTESIAN_POINT('Ctrl Pts',(-0.144224504419512,0.266085229450651,
-0.982150700573014));
#76416=CARTESIAN_POINT('Ctrl Pts',(-0.301782802897294,0.0230042796520985,
-0.966266770499029));
#76417=CARTESIAN_POINT('Ctrl Pts',(-0.182889995604558,-0.241149966855945,
-0.950382840425037));
#76418=CARTESIAN_POINT('Ctrl Pts',(0.103540991577281,-0.284396413602654,
-0.934498910351052));
#76419=CARTESIAN_POINT('Ctrl Pts',(0.295122234707084,-0.0671187275531662,
-0.918614980277062));
#76420=CARTESIAN_POINT('Ctrl Pts',(0.216353851088915,0.211643729238206,
-0.902731050203075));
#76421=CARTESIAN_POINT('Ctrl Pts',(-0.0606076064785213,0.296527865543533,
-0.886847120129086));
#76422=CARTESIAN_POINT('Ctrl Pts',(-0.28204886982603,0.10977473314346,-0.870963190055099));
#76423=CARTESIAN_POINT('Ctrl Pts',(-0.245116490950899,-0.177538623602801,
-0.85507925998111));
#76424=CARTESIAN_POINT('Ctrl Pts',(0.0163572611085327,-0.30221597743317,
-0.839195329907123));
#76425=CARTESIAN_POINT('Ctrl Pts',(0.262846783193899,-0.15004541169752,
-0.823311399833134));
#76426=CARTESIAN_POINT('Ctrl Pts',(0.268552923441213,0.139575729688357,
-0.807427469759146));
#76427=CARTESIAN_POINT('Ctrl Pts',(0.0282485159354271,0.301337150637463,
-0.791543539685159));
#76428=CARTESIAN_POINT('Ctrl Pts',(-0.237933222524112,0.187055709953346,
-0.77565960961117));
#76429=CARTESIAN_POINT('Ctrl Pts',(-0.286153891516353,-0.0985799542346567,
-0.759775679537182));
#76430=CARTESIAN_POINT('Ctrl Pts',(-0.0722404727781009,-0.293910481438916,
-0.743891749463194));
#76431=CARTESIAN_POINT('Ctrl Pts',(0.20784954180709,-0.220001420398691,
-0.728007819389205));
#76432=CARTESIAN_POINT('Ctrl Pts',(0.29753693863271,0.0554421063446759,
-0.712123889315217));
#76433=CARTESIAN_POINT('Ctrl Pts',(0.114662695421532,0.280097346087977,
-0.696239959241229));
#76434=CARTESIAN_POINT('Ctrl Pts',(-0.173249438072272,0.248166656129505,
-0.680356029167241));
#76435=CARTESIAN_POINT('Ctrl Pts',(-0.302454719255812,-0.0110995408350489,
-0.664472099093253));
#76436=CARTESIAN_POINT('Ctrl Pts',(-0.154593379077758,-0.260197894211651,
-0.648588169019265));
#76437=CARTESIAN_POINT('Ctrl Pts',(0.13488474701564,-0.270939406564237,
-0.632704238945277));
#76438=CARTESIAN_POINT('Ctrl Pts',(0.30080037350324,-0.0334842098187864,
-0.616820308871289));
#76439=CARTESIAN_POINT('Ctrl Pts',(0.191164858332551,0.234644526775151,
-0.600936378797301));
#76440=CARTESIAN_POINT('Ctrl Pts',(-0.0935891061436223,0.287824835999382,
-0.585052448723312));
#76441=CARTESIAN_POINT('Ctrl Pts',(-0.292609849134122,0.0773403723594089,
-0.569168518649325));
#76442=CARTESIAN_POINT('Ctrl Pts',(-0.223582460898843,-0.203992500315843,
-0.553284588575336));
#76443=CARTESIAN_POINT('Ctrl Pts',(0.0502598404214115,-0.298456036038071,
-0.537400658501348));
#76444=CARTESIAN_POINT('Ctrl Pts',(0.278061120430529,-0.119515983502741,
-0.52151672842736));
#76445=CARTESIAN_POINT('Ctrl Pts',(0.251141775280176,0.168907861612897,
-0.505632798353372));
#76446=CARTESIAN_POINT('Ctrl Pts',(-0.00583846403587734,0.302601998248909,
-0.489748868279384));
#76447=CARTESIAN_POINT('Ctrl Pts',(-0.257470320947409,0.159094597154208,
-0.473864938205395));
#76448=CARTESIAN_POINT('Ctrl Pts',(-0.27324395712347,-0.130152974964262,
-0.457981008131408));
#76449=CARTESIAN_POINT('Ctrl Pts',(-0.038709778056815,-0.300172633813816,
-0.442097078057419));
#76450=CARTESIAN_POINT('Ctrl Pts',(0.231284874187964,-0.195216198134616,
-0.426213147983432));
#76451=CARTESIAN_POINT('Ctrl Pts',(0.289408741618445,0.0885699565567235,
-0.410329217909442));
#76452=CARTESIAN_POINT('Ctrl Pts',(0.0824168843399205,0.291220731084257,
-0.394445287835456));
#76453=CARTESIAN_POINT('Ctrl Pts',(-0.20007377163944,0.22709588971836,-0.378561357761467));
#76454=CARTESIAN_POINT('Ctrl Pts',(-0.299284878870036,-0.0450623759147606,
-0.362677427687479));
#76455=CARTESIAN_POINT('Ctrl Pts',(-0.124333131564319,-0.275940808459303,
-0.34679349761349));
#76456=CARTESIAN_POINT('Ctrl Pts',(0.164515210600611,-0.254040949013069,
-0.330909567539503));
#76457=CARTESIAN_POINT('Ctrl Pts',(0.302657763237072,0.000575622226092337,
-0.315025637465514));
#76458=CARTESIAN_POINT('Ctrl Pts',(0.163547717428012,0.254664887161466,
-0.299141707391526));
#76459=CARTESIAN_POINT('Ctrl Pts',(-0.125381868641413,0.27546588024815,
-0.283257777317538));
#76460=CARTESIAN_POINT('Ctrl Pts',(-0.299454075160033,0.0439236365530725,
-0.26737384724355));
#76461=CARTESIAN_POINT('Ctrl Pts',(-0.19920859253459,-0.227855273325648,
-0.251489917169562));
#76462=CARTESIAN_POINT('Ctrl Pts',(0.08352419192347,-0.290905143533485,
-0.235605987095574));
#76463=CARTESIAN_POINT('Ctrl Pts',(0.289743225271439,-0.0874684465770746,
-0.219722057021586));
#76464=CARTESIAN_POINT('Ctrl Pts',(0.230541259520392,0.196094489249849,
-0.203838126947598));
#76465=CARTESIAN_POINT('Ctrl Pts',(-0.0398524593289804,0.300023314951801,
-0.18795419687361));
#76466=CARTESIAN_POINT('Ctrl Pts',(-0.273734807748427,0.129112494839419,
-0.172070266799621));
#76467=CARTESIAN_POINT('Ctrl Pts',(-0.256867585493483,-0.160072454233161,
-0.156186336725633));
#76468=CARTESIAN_POINT('Ctrl Pts',(-0.00467920973175626,-0.302622683277977,
-0.140302406651645));
#76469=CARTESIAN_POINT('Ctrl Pts',(0.251766812002862,-0.167950083134505,
-0.124418476577657));
#76470=CARTESIAN_POINT('Ctrl Pts',(0.277634357580187,0.120570367369091,
-0.108534546503669));
#76471=CARTESIAN_POINT('Ctrl Pts',(0.0490671523602165,0.298649708032275,
-0.0926506164296805));
#76472=CARTESIAN_POINT('Ctrl Pts',(-0.224247426487058,0.203131573609421,
-0.0767666863556922));
#76473=CARTESIAN_POINT('Ctrl Pts',(-0.292525653010615,-0.078434710875347,
-0.0608827562817043));
#76474=CARTESIAN_POINT('Ctrl Pts',(-0.0920270925685949,-0.288255837848017,
-0.0449962314774693));
#76475=CARTESIAN_POINT('Ctrl Pts',(0.0967307674255891,-0.251907195162304,
-0.0344043500312305));
#76476=CARTESIAN_POINT('Ctrl Pts',(0.162563208373966,-0.197797426602863,
-0.0291071119429875));
#76477=CARTESIAN_POINT('Ctrl Pts',(-0.120560253889163,0.247504423018841,
-1.97171212437062));
#76478=CARTESIAN_POINT('Ctrl Pts',(-0.202917153855632,0.207389847584819,
-1.9664163208236));
#76479=CARTESIAN_POINT('Ctrl Pts',(-0.322989644512786,0.0391927971072032,
-1.95582587391858));
#76480=CARTESIAN_POINT('Ctrl Pts',(-0.207753447102797,-0.250786683203076,
-1.93994078365557));
#76481=CARTESIAN_POINT('Ctrl Pts',(0.0980654838116881,-0.310221733153001,
-1.92405685358158));
#76482=CARTESIAN_POINT('Ctrl Pts',(0.313908617740286,-0.0858686614081634,
-1.90817292350759));
#76483=CARTESIAN_POINT('Ctrl Pts',(0.242266678218659,0.217349167322007,
-1.89228899343361));
#76484=CARTESIAN_POINT('Ctrl Pts',(-0.0513447488707591,0.321355617652953,
-1.87640506335962));
#76485=CARTESIAN_POINT('Ctrl Pts',(-0.297901046884685,0.131036848418228,
-1.86052113328563));
#76486=CARTESIAN_POINT('Ctrl Pts',(-0.271572771344087,-0.179348706334606,
-1.84463720321164));
#76487=CARTESIAN_POINT('Ctrl Pts',(0.00353796955338376,-0.325424829517193,
-1.82875327313765));
#76488=CARTESIAN_POINT('Ctrl Pts',(0.27540480933343,-0.173400338976277,
-1.81286934306366));
#76489=CARTESIAN_POINT('Ctrl Pts',(0.294985887218045,0.137473428670053,
-1.79698541298968));
#76490=CARTESIAN_POINT('Ctrl Pts',(0.0443414431724512,0.32241111519578,
-1.78110148291569));
#76491=CARTESIAN_POINT('Ctrl Pts',(-0.246921998502703,0.212002076430359,
-1.7652175528417));
#76492=CARTESIAN_POINT('Ctrl Pts',(-0.311990332725711,-0.0926141518795645,
-1.74933362276771));
#76493=CARTESIAN_POINT('Ctrl Pts',(-0.0912567385409681,-0.312389960150921,
-1.73344969269373));
#76494=CARTESIAN_POINT('Ctrl Pts',(0.213073428881872,-0.245998036825041,
-1.71756576261974));
#76495=CARTESIAN_POINT('Ctrl Pts',(0.322215616788258,0.0457428948195131,
-1.70168183254575));
#76496=CARTESIAN_POINT('Ctrl Pts',(0.136189002286588,0.295580552389366,
-1.68579790247176));
#76497=CARTESIAN_POINT('Ctrl Pts',(-0.174594879086708,0.274648760467226,
-1.66991397239777));
#76498=CARTESIAN_POINT('Ctrl Pts',(-0.325439408177928,0.00212225691052003,
-1.65403004232379));
#76499=CARTESIAN_POINT('Ctrl Pts',(-0.178161963119117,-0.272348354477677,
-1.63814611224979));
#76500=CARTESIAN_POINT('Ctrl Pts',(0.132322499916734,-0.297331579568586,
-1.62226218217581));
#76501=CARTESIAN_POINT('Ctrl Pts',(0.321591635658101,-0.0499412840340122,
-1.60637825210182));
#76502=CARTESIAN_POINT('Ctrl Pts',(0.216263589144758,0.243198215169573,
-1.59049432202783));
#76503=CARTESIAN_POINT('Ctrl Pts',(-0.087174845798447,0.313553597079832,
-1.57461039195384));
#76504=CARTESIAN_POINT('Ctrl Pts',(-0.310755905646206,0.0966751211428172,
-1.55872646187986));
#76505=CARTESIAN_POINT('Ctrl Pts',(-0.249665960617232,-0.208763550549125,
-1.54284253180586));
#76506=CARTESIAN_POINT('Ctrl Pts',(0.0401329440196797,-0.322962317850671,
-1.52695860173188));
#76507=CARTESIAN_POINT('Ctrl Pts',(0.293167670441246,-0.14130827629126,
-1.51107467165789));
#76508=CARTESIAN_POINT('Ctrl Pts',(0.27764326793412,0.169792602047461,-1.4951907415839));
#76509=CARTESIAN_POINT('Ctrl Pts',(0.00778101816686971,0.325353296737565,
-1.47930681150992));
#76510=CARTESIAN_POINT('Ctrl Pts',(-0.269209109849831,0.182870902864458,
-1.46342288143592));
#76511=CARTESIAN_POINT('Ctrl Pts',(-0.299587584096736,-0.12713218080258,
-1.44753895136194));
#76512=CARTESIAN_POINT('Ctrl Pts',(-0.0555259043541897,-0.320674579420522,
-1.43165502128795));
#76513=CARTESIAN_POINT('Ctrl Pts',(0.239400826379785,-0.220459874510939,
-1.41577109121396));
#76514=CARTESIAN_POINT('Ctrl Pts',(0.315022074694887,0.0817092675015477,
-1.39988716113997));
#76515=CARTESIAN_POINT('Ctrl Pts',(0.102064252050996,0.309027831099441,
-1.38400323106599));
#76516=CARTESIAN_POINT('Ctrl Pts',(-0.204390532872595,0.253258409559849,
-1.368119300992));
#76517=CARTESIAN_POINT('Ctrl Pts',(-0.323611359203487,-0.0345108698123119,
-1.35223537091801));
#76518=CARTESIAN_POINT('Ctrl Pts',(-0.146384815993087,-0.290666127347867,
-1.33635144084402));
#76519=CARTESIAN_POINT('Ctrl Pts',(0.164938978156682,-0.280553819124534,
-1.32046751077003));
#76520=CARTESIAN_POINT('Ctrl Pts',(0.32516879856669,-0.0134374245831591,
-1.30458358069605));
#76521=CARTESIAN_POINT('Ctrl Pts',(0.187524541783422,0.26598845495557,-1.28869965062206));
#76522=CARTESIAN_POINT('Ctrl Pts',(-0.12190341651441,0.301752993328728,
-1.27281572054807));
#76523=CARTESIAN_POINT('Ctrl Pts',(-0.319660550732573,0.0610937332799438,
-1.25693179047408));
#76524=CARTESIAN_POINT('Ctrl Pts',(-0.224589492380374,-0.235531042228108,
-1.24104786040009));
#76525=CARTESIAN_POINT('Ctrl Pts',(0.0762189801548472,-0.316395289163552,
-1.2251639303261));
#76526=CARTESIAN_POINT('Ctrl Pts',(0.307206306016977,-0.107422518515145,
-1.20928000025212));
#76527=CARTESIAN_POINT('Ctrl Pts',(0.256774272715115,0.199955707126246,
-1.19339607017813));
#76528=CARTESIAN_POINT('Ctrl Pts',(-0.0288783594545779,0.324162539933202,
-1.17751214010414));
#76529=CARTESIAN_POINT('Ctrl Pts',(-0.288076686317903,0.151417088668452,
-1.16162821003015));
#76530=CARTESIAN_POINT('Ctrl Pts',(-0.28337953035481,-0.160035476431385,
-1.14574427995616));
#76531=CARTESIAN_POINT('Ctrl Pts',(-0.0190897674996043,-0.324885968791427,
-1.12986034988218));
#76532=CARTESIAN_POINT('Ctrl Pts',(0.262687364693754,-0.192121472956523,
-1.11397641980818));
#76533=CARTESIAN_POINT('Ctrl Pts',(0.303827151934601,0.116637788422287,
-1.0980924897342));
#76534=CARTESIAN_POINT('Ctrl Pts',(0.0666430873553909,0.318549856142606,
-1.08220855966021));
#76535=CARTESIAN_POINT('Ctrl Pts',(-0.231590033082807,0.228651193999587,
-1.06632462958623));
#76536=CARTESIAN_POINT('Ctrl Pts',(-0.317672825150698,-0.0707056440569471,
-1.05044069951223));
#76537=CARTESIAN_POINT('Ctrl Pts',(-0.112748300224307,-0.305291881217406,
-1.03455676943825));
#76538=CARTESIAN_POINT('Ctrl Pts',(0.19546041442897,-0.260212486887136,
-1.01867283936426));
#76539=CARTESIAN_POINT('Ctrl Pts',(0.324615693351377,0.0232371162310966,
-1.00278890929027));
#76540=CARTESIAN_POINT('Ctrl Pts',(0.156403572554879,0.285400130400817,
-0.986904979216284));
#76541=CARTESIAN_POINT('Ctrl Pts',(-0.155083579701816,0.286119547126029,
-0.971021049142295));
#76542=CARTESIAN_POINT('Ctrl Pts',(-0.32450489293849,0.0247363376374115,
-0.955137119068307));
#76543=CARTESIAN_POINT('Ctrl Pts',(-0.196660306264625,-0.259306837319491,
-0.939253188994319));
#76544=CARTESIAN_POINT('Ctrl Pts',(0.111336888861641,-0.305809432685363,
-0.92336925892033));
#76545=CARTESIAN_POINT('Ctrl Pts',(0.317342831526365,-0.0721722884462076,
-0.907485328846344));
#76546=CARTESIAN_POINT('Ctrl Pts',(0.232643751103116,0.227578990711806,
-0.891601398772354));
#76547=CARTESIAN_POINT('Ctrl Pts',(-0.0651709264502512,0.318854296327255,
-0.875717468698368));
#76548=CARTESIAN_POINT('Ctrl Pts',(-0.303285135626059,0.118039986652897,
-0.859833538624378));
#76549=CARTESIAN_POINT('Ctrl Pts',(-0.263572012354034,-0.19090601416503,
-0.843949608550391));
#76550=CARTESIAN_POINT('Ctrl Pts',(0.017588846063562,-0.324970682423638,
-0.828065678476401));
#76551=CARTESIAN_POINT('Ctrl Pts',(0.282637268991736,-0.161342759731034,
-0.812181748402415));
#76552=CARTESIAN_POINT('Ctrl Pts',(0.288773040852392,0.15008478543009,-0.796297818328426));
#76553=CARTESIAN_POINT('Ctrl Pts',(0.0303754274640274,0.324025686245876,
-0.780413888254438));
#76554=CARTESIAN_POINT('Ctrl Pts',(-0.255847895110093,0.201139669156703,
-0.76452995818045));
#76555=CARTESIAN_POINT('Ctrl Pts',(-0.307699236135894,-0.106002320833652,
-0.748646028106462));
#76556=CARTESIAN_POINT('Ctrl Pts',(-0.0776796645124351,-0.316039841890178,
-0.732762098032473));
#76557=CARTESIAN_POINT('Ctrl Pts',(0.223499128061244,-0.236565956334796,
-0.716878167958486));
#76558=CARTESIAN_POINT('Ctrl Pts',(0.319939345414303,0.0596165010429236,
-0.700994237884497));
#76559=CARTESIAN_POINT('Ctrl Pts',(0.123295977585797,0.30118667608627,-0.68511030781051));
#76560=CARTESIAN_POINT('Ctrl Pts',(-0.186293883592927,0.2668518331895,-0.669226377736521));
#76561=CARTESIAN_POINT('Ctrl Pts',(-0.325227399800682,-0.011935256998621,
-0.653342447662532));
#76562=CARTESIAN_POINT('Ctrl Pts',(-0.16623315657818,-0.279788937584717,
-0.637458517588546));
#76563=CARTESIAN_POINT('Ctrl Pts',(0.145040605260206,-0.291339209112815,
-0.621574587514556));
#76564=CARTESIAN_POINT('Ctrl Pts',(0.323448493626547,-0.0360053317089568,
-0.605690657440569));
#76565=CARTESIAN_POINT('Ctrl Pts',(0.205558207065626,0.252311584055658,
-0.58980672736658));
#76566=CARTESIAN_POINT('Ctrl Pts',(-0.100635697520777,0.30949599080636,
-0.573922797292592));
#76567=CARTESIAN_POINT('Ctrl Pts',(-0.314641281260587,0.0831635501140697,
-0.558038867218604));
#76568=CARTESIAN_POINT('Ctrl Pts',(-0.240416623612565,-0.21935167888866,
-0.542154937144616));
#76569=CARTESIAN_POINT('Ctrl Pts',(0.0540440475019573,-0.320927644291056,
-0.526271007070628));
#76570=CARTESIAN_POINT('Ctrl Pts',(0.298997137177409,-0.128514683602414,
-0.51038707699664));
#76571=CARTESIAN_POINT('Ctrl Pts',(0.27005095756703,0.181625417429157,-0.494503146922652));
#76572=CARTESIAN_POINT('Ctrl Pts',(-0.00627805868557644,0.325385767850246,
-0.478619216848664));
#76573=CARTESIAN_POINT('Ctrl Pts',(-0.276855997531152,0.171073284232798,
-0.462735286774675));
#76574=CARTESIAN_POINT('Ctrl Pts',(-0.293817275872469,-0.139952564562724,
-0.446851356700688));
#76575=CARTESIAN_POINT('Ctrl Pts',(-0.0416243479197691,-0.322773489621168,
-0.430967426626699));
#76576=CARTESIAN_POINT('Ctrl Pts',(0.248698973619779,-0.209914583824356,
-0.415083496552711));
#76577=CARTESIAN_POINT('Ctrl Pts',(0.311199153207941,0.0952386418114992,
-0.399199566478723));
#76578=CARTESIAN_POINT('Ctrl Pts',(0.0886222871955774,0.313147572541195,
-0.383315636404735));
#76579=CARTESIAN_POINT('Ctrl Pts',(-0.215137897926383,0.24419458853296,
-0.367431706330747));
#76580=CARTESIAN_POINT('Ctrl Pts',(-0.32181889306954,-0.0484552510328077,
-0.351547776256759));
#76581=CARTESIAN_POINT('Ctrl Pts',(-0.133694528514001,-0.296717180855799,
-0.33566384618277));
#76582=CARTESIAN_POINT('Ctrl Pts',(0.176902031163362,-0.273168418379144,
-0.319779916108783));
#76583=CARTESIAN_POINT('Ctrl Pts',(0.325445731543802,0.000618962469223088,
-0.303895986034794));
#76584=CARTESIAN_POINT('Ctrl Pts',(0.175861692663694,0.2738393346146,-0.288012055960806));
#76585=CARTESIAN_POINT('Ctrl Pts',(-0.134822228004013,0.296206493941789,
-0.272128125886818));
#76586=CARTESIAN_POINT('Ctrl Pts',(-0.32200082863195,0.0472307727288739,
-0.25624419581283));
#76587=CARTESIAN_POINT('Ctrl Pts',(-0.214207577013145,-0.245011148303151,
-0.240360265738842));
#76588=CARTESIAN_POINT('Ctrl Pts',(0.0898129671329327,-0.312808223501447,
-0.224476335664854));
#76589=CARTESIAN_POINT('Ctrl Pts',(0.311558821091472,-0.0940541959962185,
-0.208592405590866));
#76590=CARTESIAN_POINT('Ctrl Pts',(0.247899370077859,0.210859003988727,
-0.192708475516877));
#76591=CARTESIAN_POINT('Ctrl Pts',(-0.0428530649318907,0.322612928115123,
-0.17682454544289));
#76592=CARTESIAN_POINT('Ctrl Pts',(-0.294345084044343,0.138833743714504,
-0.160940615368901));
#76593=CARTESIAN_POINT('Ctrl Pts',(-0.276207880401654,-0.17212476696696,
-0.145056685294913));
#76594=CARTESIAN_POINT('Ctrl Pts',(-0.00503152081054036,-0.325408010314291,
-0.129172755220925));
#76595=CARTESIAN_POINT('Ctrl Pts',(0.270723055091573,-0.180595525070797,
-0.113288825146937));
#76596=CARTESIAN_POINT('Ctrl Pts',(0.298538242131932,0.129648455044593,
-0.0974048950729486));
#76597=CARTESIAN_POINT('Ctrl Pts',(0.0527615585466883,0.321135898403419,
-0.0815209649989606));
#76598=CARTESIAN_POINT('Ctrl Pts',(-0.241131656361081,0.218425930549086,
-0.0656370349249724));
#76599=CARTESIAN_POINT('Ctrl Pts',(-0.314550745770222,-0.0843402845056338,
-0.0497531048509844));
#76600=CARTESIAN_POINT('Ctrl Pts',(-0.098956075477821,-0.309959444016429,
-0.0338665800467495));
#76601=CARTESIAN_POINT('Ctrl Pts',(0.104013903462819,-0.270874008100452,
-0.0232746986005106));
#76602=CARTESIAN_POINT('Ctrl Pts',(0.174803057108209,-0.212690160363829,
-0.0179774605122677));
#76603=CARTESIAN_POINT('Ctrl Pts',(-0.129001978509869,0.264834879069913,
-1.9605824729399));
#76604=CARTESIAN_POINT('Ctrl Pts',(-0.217125573947727,0.221911449240131,
-1.95528666939287));
#76605=CARTESIAN_POINT('Ctrl Pts',(-0.34560563565713,0.0419371078532527,
-1.94469622248786));
#76606=CARTESIAN_POINT('Ctrl Pts',(-0.222300508284811,-0.268346965716144,
-1.92881113222485));
#76607=CARTESIAN_POINT('Ctrl Pts',(0.10493210678592,-0.331943705014839,
-1.91292720215086));
#76608=CARTESIAN_POINT('Ctrl Pts',(0.33588874818582,-0.0918812532016676,
-1.89704327207688));
#76609=CARTESIAN_POINT('Ctrl Pts',(0.259230383223593,0.232568128446287,
-1.88115934200289));
#76610=CARTESIAN_POINT('Ctrl Pts',(-0.0549399489197289,0.343857192940258,
-1.8652754119289));
#76611=CARTESIAN_POINT('Ctrl Pts',(-0.318760314519713,0.140212152499201,
-1.84939148185491));
#76612=CARTESIAN_POINT('Ctrl Pts',(-0.290588512238902,-0.191906845033854,
-1.83350755178092));
#76613=CARTESIAN_POINT('Ctrl Pts',(0.00378570098826755,-0.348211334247439,
-1.81762362170694));
#76614=CARTESIAN_POINT('Ctrl Pts',(0.294688872568306,-0.185541968274115,
-1.80173969163295));
#76615=CARTESIAN_POINT('Ctrl Pts',(0.31564103306055,0.14709942720655,-1.78585576155896));
#76616=CARTESIAN_POINT('Ctrl Pts',(0.0474462662005358,0.344986597258388,
-1.76997183148497));
#76617=CARTESIAN_POINT('Ctrl Pts',(-0.264211672727102,0.22684663000843,
-1.75408790141098));
#76618=CARTESIAN_POINT('Ctrl Pts',(-0.333836143332704,-0.0990990682672344,
-1.73820397133699));
#76619=CARTESIAN_POINT('Ctrl Pts',(-0.0976466077698041,-0.33426375298726,
-1.72232004126301));
#76620=CARTESIAN_POINT('Ctrl Pts',(0.227992999408525,-0.263223014519772,
-1.70643611118902));
#76621=CARTESIAN_POINT('Ctrl Pts',(0.344777409897277,0.0489458486037273,
-1.69055218111503));
#76622=CARTESIAN_POINT('Ctrl Pts',(0.145725064268752,0.316277337158927,
-1.67466825104104));
#76623=CARTESIAN_POINT('Ctrl Pts',(-0.186820151030732,0.2938798845607,-1.65878432096705));
#76624=CARTESIAN_POINT('Ctrl Pts',(-0.348226933717562,0.00227085902303463,
-1.64290039089307));
#76625=CARTESIAN_POINT('Ctrl Pts',(-0.190637005116948,-0.291418402318793,
-1.62701646081908));
#76626=CARTESIAN_POINT('Ctrl Pts',(0.141587826335567,-0.31815097265037,
-1.61113253074509));
#76627=CARTESIAN_POINT('Ctrl Pts',(0.344109737113365,-0.0534382123617138,
-1.5952486006711));
#76628=CARTESIAN_POINT('Ctrl Pts',(0.231406537223853,0.260227147130818,
-1.57936467059712));
#76629=CARTESIAN_POINT('Ctrl Pts',(-0.0932788976591828,0.335508868697075,
-1.56348074052312));
#76630=CARTESIAN_POINT('Ctrl Pts',(-0.33251528068979,0.10344438981997,-1.54759681044914));
#76631=CARTESIAN_POINT('Ctrl Pts',(-0.267147769245746,-0.223381339975787,
-1.53171288037515));
#76632=CARTESIAN_POINT('Ctrl Pts',(0.0429430845983787,-0.345576395560456,
-1.51582895030116));
#76633=CARTESIAN_POINT('Ctrl Pts',(0.313695503302601,-0.151202793900476,
-1.49994502022717));
#76634=CARTESIAN_POINT('Ctrl Pts',(0.297084069816041,0.181681614743433,
-1.48406109015319));
#76635=CARTESIAN_POINT('Ctrl Pts',(0.00832585123178702,0.348134792685833,
-1.4681771600792));
#76636=CARTESIAN_POINT('Ctrl Pts',(-0.288059345291665,0.195675668558975,
-1.45229323000521));
#76637=CARTESIAN_POINT('Ctrl Pts',(-0.320564944405325,-0.136034076959434,
-1.43640929993122));
#76638=CARTESIAN_POINT('Ctrl Pts',(-0.0594138722271255,-0.343128467870509,
-1.42052536985723));
#76639=CARTESIAN_POINT('Ctrl Pts',(0.256163862165409,-0.23589664982039,
-1.40464143978325));
#76640=CARTESIAN_POINT('Ctrl Pts',(0.337080170279715,0.0874306152339582,
-1.38875750970926));
#76641=CARTESIAN_POINT('Ctrl Pts',(0.109210871949668,0.330666204992337,
-1.37287357963527));
#76642=CARTESIAN_POINT('Ctrl Pts',(-0.218702120132325,0.270991764313301,
-1.35698964956128));
#76643=CARTESIAN_POINT('Ctrl Pts',(-0.346270883303697,-0.0369273482948824,
-1.34110571948729));
#76644=CARTESIAN_POINT('Ctrl Pts',(-0.156634796939567,-0.311018800177289,
-1.32522178941331));
#76645=CARTESIAN_POINT('Ctrl Pts',(0.176488136257323,-0.300198420109819,
-1.30933785933932));
#76646=CARTESIAN_POINT('Ctrl Pts',(0.347937375806666,-0.0143783237127102,
-1.29345392926533));
#76647=CARTESIAN_POINT('Ctrl Pts',(0.20065515896689,0.284613177586684,-1.27756999919134));
#76648=CARTESIAN_POINT('Ctrl Pts',(-0.130439190447699,0.322881977309613,
-1.26168606911735));
#76649=CARTESIAN_POINT('Ctrl Pts',(-0.342043436089377,0.0653715649513554,
-1.24580213904337));
#76650=CARTESIAN_POINT('Ctrl Pts',(-0.240315426809168,-0.252023112657438,
-1.22991820896938));
#76651=CARTESIAN_POINT('Ctrl Pts',(0.0815558936116627,-0.338549538314881,
-1.21403427889539));
#76652=CARTESIAN_POINT('Ctrl Pts',(0.328717135278538,-0.114944328482481,
-1.1981503488214));
#76653=CARTESIAN_POINT('Ctrl Pts',(0.274753810995919,0.213956764368961,
-1.18226641874741));
#76654=CARTESIAN_POINT('Ctrl Pts',(-0.030900445093492,0.346860658145371,
-1.16638248867342));
#76655=CARTESIAN_POINT('Ctrl Pts',(-0.30824804443214,0.162019433339887,
-1.15049855859943));
#76656=CARTESIAN_POINT('Ctrl Pts',(-0.303221989882145,-0.171241287451154,
-1.13461462852545));
#76657=CARTESIAN_POINT('Ctrl Pts',(-0.0204264481643065,-0.347634742066163,
-1.11873069845146));
#76658=CARTESIAN_POINT('Ctrl Pts',(0.2810809423659,-0.205573970907589,-1.10284676837747));
#76659=CARTESIAN_POINT('Ctrl Pts',(0.32510137014655,0.124804858899214,-1.08696283830348));
#76660=CARTESIAN_POINT('Ctrl Pts',(0.0713094892016032,0.340854969783078,
-1.0710789082295));
#76661=CARTESIAN_POINT('Ctrl Pts',(-0.247806150925284,0.244661531998007,
-1.05519497815551));
#76662=CARTESIAN_POINT('Ctrl Pts',(-0.339916528385347,-0.0756565093463238,
-1.03931104808152));
#76663=CARTESIAN_POINT('Ctrl Pts',(-0.12064302565199,-0.32666866093574,
-1.02342711800753));
#76664=CARTESIAN_POINT('Ctrl Pts',(0.209146707710798,-0.278432771651885,
-1.00754318793354));
#76665=CARTESIAN_POINT('Ctrl Pts',(0.347345541725384,0.0248641975441668,
-0.991659257859552));
#76666=CARTESIAN_POINT('Ctrl Pts',(0.16735507478394,0.305384073946364,-0.975775327785563));
#76667=CARTESIAN_POINT('Ctrl Pts',(-0.16594265498412,0.306153864801407,
-0.959891397711576));
#76668=CARTESIAN_POINT('Ctrl Pts',(-0.347226982979686,0.0264683956227249,
-0.944007467637586));
#76669=CARTESIAN_POINT('Ctrl Pts',(-0.21043061692469,-0.277463707783037,
-0.928123537563599));
#76670=CARTESIAN_POINT('Ctrl Pts',(0.119132786145999,-0.327222451768071,
-0.912239607489611));
#76671=CARTESIAN_POINT('Ctrl Pts',(0.339563428345645,-0.0772258493392489,
-0.896355677415623));
#76672=CARTESIAN_POINT('Ctrl Pts',(0.248933651117318,0.243514252185408,
-0.880471747341634));
#76673=CARTESIAN_POINT('Ctrl Pts',(-0.0697342464219807,0.341180727110977,
-0.864587817267647));
#76674=CARTESIAN_POINT('Ctrl Pts',(-0.324521401426087,0.126305240162334,
-0.848703887193659));
#76675=CARTESIAN_POINT('Ctrl Pts',(-0.282027533757167,-0.204273404727259,
-0.83281995711967));
#76676=CARTESIAN_POINT('Ctrl Pts',(0.018820431018591,-0.347725387414107,
-0.816936027045682));
#76677=CARTESIAN_POINT('Ctrl Pts',(0.302427754789573,-0.172640107764547,
-0.801052096971694));
#76678=CARTESIAN_POINT('Ctrl Pts',(0.308993158263571,0.160593841171823,
-0.785168166897706));
#76679=CARTESIAN_POINT('Ctrl Pts',(0.0325023389926279,0.346714221854288,
-0.769284236823718));
#76680=CARTESIAN_POINT('Ctrl Pts',(-0.273762567696073,0.215223628360061,
-0.75340030674973));
#76681=CARTESIAN_POINT('Ctrl Pts',(-0.329244580755436,-0.113424687432649,
-0.737516376675742));
#76682=CARTESIAN_POINT('Ctrl Pts',(-0.0831188562467696,-0.338169202341438,
-0.721632446601753));
#76683=CARTESIAN_POINT('Ctrl Pts',(0.239148714315398,-0.253130492270901,
-0.705748516527766));
#76684=CARTESIAN_POINT('Ctrl Pts',(0.342341752195895,0.0637908957411709,
-0.689864586453776));
#76685=CARTESIAN_POINT('Ctrl Pts',(0.131929259750061,0.322276006084563,
-0.67398065637979));
#76686=CARTESIAN_POINT('Ctrl Pts',(-0.199338329113583,0.285537010249495,
-0.658096726305801));
#76687=CARTESIAN_POINT('Ctrl Pts',(-0.348000080345551,-0.012770973162193,
-0.642212796231813));
#76688=CARTESIAN_POINT('Ctrl Pts',(-0.177872934078603,-0.299379980957783,
-0.626328866157825));
#76689=CARTESIAN_POINT('Ctrl Pts',(0.155196463504772,-0.311739011661393,
-0.610444936083836));
#76690=CARTESIAN_POINT('Ctrl Pts',(0.346096613749853,-0.0385264535991275,
-0.594561006009849));
#76691=CARTESIAN_POINT('Ctrl Pts',(0.219951555798699,0.269978641336165,
-0.578677075935861));
#76692=CARTESIAN_POINT('Ctrl Pts',(-0.107682288897933,0.331167145613336,
-0.562793145861872));
#76693=CARTESIAN_POINT('Ctrl Pts',(-0.336672713387052,0.0889867278687308,
-0.546909215787884));
#76694=CARTESIAN_POINT('Ctrl Pts',(-0.257250786326287,-0.234710857461478,
-0.531025285713896));
#76695=CARTESIAN_POINT('Ctrl Pts',(0.0578282545825028,-0.34339925254404,
-0.515141355639908));
#76696=CARTESIAN_POINT('Ctrl Pts',(0.319933153924289,-0.13751338370209,
-0.49925742556592));
#76697=CARTESIAN_POINT('Ctrl Pts',(0.288960139853882,0.194342973245417,
-0.483373495491932));
#76698=CARTESIAN_POINT('Ctrl Pts',(-0.00671765333527564,0.348169537451584,
-0.467489565417944));
#76699=CARTESIAN_POINT('Ctrl Pts',(-0.296241674114894,0.183051971311387,
-0.451605635343955));
#76700=CARTESIAN_POINT('Ctrl Pts',(-0.314390594621468,-0.149752154161186,
-0.435721705269968));
#76701=CARTESIAN_POINT('Ctrl Pts',(-0.0445389177827234,-0.345374345428521,
-0.419837775195979));
#76702=CARTESIAN_POINT('Ctrl Pts',(0.266113073051594,-0.224612969514096,
-0.403953845121992));
#76703=CARTESIAN_POINT('Ctrl Pts',(0.332989564797437,0.101907327066275,
-0.388069915048003));
#76704=CARTESIAN_POINT('Ctrl Pts',(0.0948276900512347,0.335074413998132,
-0.372185984974015));
#76705=CARTESIAN_POINT('Ctrl Pts',(-0.230202024213326,0.26129328734756,
-0.356302054900027));
#76706=CARTESIAN_POINT('Ctrl Pts',(-0.344352907269043,-0.0518481261508553,
-0.340418124826038));
#76707=CARTESIAN_POINT('Ctrl Pts',(-0.143055925463681,-0.317493553252295,
-0.324534194752051));
#76708=CARTESIAN_POINT('Ctrl Pts',(0.189288851726114,-0.292295887745218,
-0.308650264678062));
#76709=CARTESIAN_POINT('Ctrl Pts',(0.348233699850533,0.000662302712354398,
-0.292766334604074));
#76710=CARTESIAN_POINT('Ctrl Pts',(0.188175667899375,0.293013782067735,
-0.276882404530086));
#76711=CARTESIAN_POINT('Ctrl Pts',(-0.144262587366613,0.316947107635427,
-0.260998474456099));
#76712=CARTESIAN_POINT('Ctrl Pts',(-0.344547582103868,0.050537908904675,
-0.24511454438211));
#76713=CARTESIAN_POINT('Ctrl Pts',(-0.2292065614917,-0.262167023280654,
-0.229230614308122));
#76714=CARTESIAN_POINT('Ctrl Pts',(0.0961017423423954,-0.334711303469409,
-0.213346684234133));
#76715=CARTESIAN_POINT('Ctrl Pts',(0.333374416911505,-0.100639945415362,
-0.197462754160146));
#76716=CARTESIAN_POINT('Ctrl Pts',(0.265257480635327,0.225623518727604,
-0.181578824086157));
#76717=CARTESIAN_POINT('Ctrl Pts',(-0.0458536705348012,0.345202541278447,
-0.16569489401217));
#76718=CARTESIAN_POINT('Ctrl Pts',(-0.314955360340258,0.148554992589589,
-0.149810963938181));
#76719=CARTESIAN_POINT('Ctrl Pts',(-0.295548175309825,-0.18417707970076,
-0.133927033864193));
#76720=CARTESIAN_POINT('Ctrl Pts',(-0.00538383188932432,-0.348193337350606,
-0.118043103790205));
#76721=CARTESIAN_POINT('Ctrl Pts',(0.289679298180285,-0.193240967007088,
-0.102159173716217));
#76722=CARTESIAN_POINT('Ctrl Pts',(0.319442126683677,0.138726542720093,
-0.0862752436422287));
#76723=CARTESIAN_POINT('Ctrl Pts',(0.05645596473316,0.343622088774564,-0.0703913135682407));
#76724=CARTESIAN_POINT('Ctrl Pts',(-0.258015886235105,0.23372028748875,
-0.0545073834942526));
#76725=CARTESIAN_POINT('Ctrl Pts',(-0.336575838529829,-0.0902458581359205,
-0.0386234534202645));
#76726=CARTESIAN_POINT('Ctrl Pts',(-0.105885058387047,-0.331663050184843,
-0.0227369286160296));
#76727=CARTESIAN_POINT('Ctrl Pts',(0.11129703950005,-0.289840821038601,
-0.0121450471697907));
#76728=CARTESIAN_POINT('Ctrl Pts',(0.187042905842451,-0.227582894124795,
-0.00684780908154777));
#76729=CARTESIAN_POINT('Ctrl Pts',(-0.289034808525452,-0.0555371045866529,
-0.04));
#76730=CARTESIAN_POINT('Ctrl Pts',(-0.288636144038534,-0.0573073412592883,
-0.04));
#76731=CARTESIAN_POINT('Ctrl Pts',(-0.288237479551616,-0.0590775779319236,
-0.04));
#76732=CARTESIAN_POINT('Ctrl Pts',(-0.287838815064698,-0.060847814604559,
-0.04));
#76733=CARTESIAN_POINT('Ctrl Pts',(-0.138000239402477,-0.193373078029398,
-1.9608));
#76734=CARTESIAN_POINT('Ctrl Pts',(-0.143086395765402,-0.190606700707026,
-1.9608));
#76735=CARTESIAN_POINT('Ctrl Pts',(-0.148054697801646,-0.187647084738665,
-1.9608));
#76736=CARTESIAN_POINT('Ctrl Pts',(-0.152892767683467,-0.184496670108783,
-1.9608));
#76737=CARTESIAN_POINT('Ctrl Pts',(-0.163043940938266,-0.177886512439802,
-1.9608));
#76738=CARTESIAN_POINT('Ctrl Pts',(-0.172622493969985,-0.170437982864818,
-1.9608));
#76739=CARTESIAN_POINT('Ctrl Pts',(-0.181598967428321,-0.162265254850832,
-1.9608));
#76740=CARTESIAN_POINT('Ctrl Pts',(-0.187293781374843,-0.157080349476667,
-1.9608));
#76741=CARTESIAN_POINT('Ctrl Pts',(-0.192748306396003,-0.151599882545997,
-1.9608));
#76742=CARTESIAN_POINT('Ctrl Pts',(-0.197929623010393,-0.145877589802222,
-1.9608));
#76743=CARTESIAN_POINT('Ctrl Pts',(-0.2048094626486,-0.138279432930144,
-1.9608));
#76744=CARTESIAN_POINT('Ctrl Pts',(-0.21121792230437,-0.130247035676296,
-1.9608));
#76745=CARTESIAN_POINT('Ctrl Pts',(-0.217136672188152,-0.121843996423096,
-1.9608));
#76746=CARTESIAN_POINT('Ctrl Pts',(-0.221200409818485,-0.116074577628095,
-1.9608));
#76747=CARTESIAN_POINT('Ctrl Pts',(-0.225034010493672,-0.110128828935726,
-1.9608));
#76748=CARTESIAN_POINT('Ctrl Pts',(-0.228627257789668,-0.10402957803314,
-1.9608));
#76749=CARTESIAN_POINT('Ctrl Pts',(-0.231459374288426,-0.0992222859966238,
-1.9608));
#76750=CARTESIAN_POINT('Ctrl Pts',(-0.234138268440307,-0.0943260187649396,
-1.9608));
#76751=CARTESIAN_POINT('Ctrl Pts',(-0.236657767742044,-0.0893577521864006,
-1.9608));
#76752=CARTESIAN_POINT('Ctrl Pts',(-0.243910061937438,-0.0750567635558887,
-1.9608));
#76753=CARTESIAN_POINT('Ctrl Pts',(-0.249855778463453,-0.060142531185048,
-1.9608));
#76754=CARTESIAN_POINT('Ctrl Pts',(-0.25441935181254,-0.0448298972586075,
-1.9608));
#76755=CARTESIAN_POINT('Ctrl Pts',(-0.257348678655569,-0.0350008211888239,
-1.9608));
#76756=CARTESIAN_POINT('Ctrl Pts',(-0.259707778490682,-0.0250074014029279,
-1.9608));
#76757=CARTESIAN_POINT('Ctrl Pts',(-0.261467624497603,-0.0148976599763562,
-1.9608));
#76758=CARTESIAN_POINT('Ctrl Pts',(-0.262470243263279,-0.00913794212005506,
-1.9608));
#76759=CARTESIAN_POINT('Ctrl Pts',(-0.26327682977629,-0.00334534667317961,
-1.9608));
#76760=CARTESIAN_POINT('Ctrl Pts',(-0.263880808002415,0.00245049521744596,
-1.9608));
#76761=CARTESIAN_POINT('Ctrl Pts',(-0.264901640441406,0.012246516261413,
-1.9608));
#76762=CARTESIAN_POINT('Ctrl Pts',(-0.265346751527308,0.0220655810592102,
-1.9608));
#76763=CARTESIAN_POINT('Ctrl Pts',(-0.265197864941953,0.0318610581547499,
-1.9608));
#76764=CARTESIAN_POINT('Ctrl Pts',(-0.265021292489645,0.0434780309543282,
-1.9608));
#76765=CARTESIAN_POINT('Ctrl Pts',(-0.264009847886286,0.0550619824997758,
-1.9608));
#76766=CARTESIAN_POINT('Ctrl Pts',(-0.262216867534709,0.0665542493180926,
-1.9608));
#76767=CARTESIAN_POINT('Ctrl Pts',(-0.261115413480366,0.0736141169120082,
-1.9608));
#76768=CARTESIAN_POINT('Ctrl Pts',(-0.259718714489693,0.0806394477428598,
-1.9608));
#76769=CARTESIAN_POINT('Ctrl Pts',(-0.258036389767163,0.0876167385651326,
-1.9608));
#76770=CARTESIAN_POINT('Ctrl Pts',(-0.256725636355855,0.0930529707172855,
-1.9608));
#76771=CARTESIAN_POINT('Ctrl Pts',(-0.255241512393281,0.0984579649283385,
-1.9608));
#76772=CARTESIAN_POINT('Ctrl Pts',(-0.253595547443031,0.103805521125184,
-1.9608));
#76773=CARTESIAN_POINT('Ctrl Pts',(-0.248517117827109,0.120304771463862,
-1.9608));
#76774=CARTESIAN_POINT('Ctrl Pts',(-0.241891167152933,0.13630805743798,
-1.9608));
#76775=CARTESIAN_POINT('Ctrl Pts',(-0.233880496481478,0.151633352688369,
-1.9608));
#76776=CARTESIAN_POINT('Ctrl Pts',(-0.229912443575941,0.159224674918506,
-1.9608));
#76777=CARTESIAN_POINT('Ctrl Pts',(-0.225603661083085,0.166649682158028,
-1.9608));
#76778=CARTESIAN_POINT('Ctrl Pts',(-0.220968694610218,0.173885464859617,
-1.9608));
#76779=CARTESIAN_POINT('Ctrl Pts',(-0.217449048122994,0.17938008867557,
-1.9608));
#76780=CARTESIAN_POINT('Ctrl Pts',(-0.213739562626335,0.184767816744313,
-1.9608));
#76781=CARTESIAN_POINT('Ctrl Pts',(-0.209851120783383,0.190030463551426,
-1.9608));
#76782=CARTESIAN_POINT('Ctrl Pts',(-0.205687585120815,0.1956654244293,-1.9608));
#76783=CARTESIAN_POINT('Ctrl Pts',(-0.201328524903064,0.201144177852673,
-1.9608));
#76784=CARTESIAN_POINT('Ctrl Pts',(-0.196786165510293,0.206452912344335,
-1.9608));
#76785=CARTESIAN_POINT('Ctrl Pts',(-0.18548209900297,0.219664171642526,
-1.9608));
#76786=CARTESIAN_POINT('Ctrl Pts',(-0.173040875473831,0.231830875283052,
-1.9608));
#76787=CARTESIAN_POINT('Ctrl Pts',(-0.15958491798273,0.24277084955155,-1.9608));
#76788=CARTESIAN_POINT('Ctrl Pts',(-0.149872809851103,0.250666996155991,
-1.9608));
#76789=CARTESIAN_POINT('Ctrl Pts',(-0.139630976873493,0.257923930314965,
-1.9608));
#76790=CARTESIAN_POINT('Ctrl Pts',(-0.128892185405331,0.264462557919713,
-1.9608));
#76791=CARTESIAN_POINT('Origin',(-3.51939854619125E-17,0.,-1.9608));
#76792=CARTESIAN_POINT('',(-0.2942,-3.60291088309151E-17,-1.9608));
#76793=CARTESIAN_POINT('Origin',(0.,0.,-1.9608));
#76794=CARTESIAN_POINT('',(0.133821547094406,0.262002735736212,-1.9608));
#76795=CARTESIAN_POINT('Origin',(0.,0.,-1.9608));
#76796=CARTESIAN_POINT('Ctrl Pts',(0.133821547094406,0.262002735736212,
-1.9608));
#76797=CARTESIAN_POINT('Ctrl Pts',(0.138297615113376,0.259182261595568,
-1.9608));
#76798=CARTESIAN_POINT('Ctrl Pts',(0.142687341570814,0.256233989666448,
-1.9608));
#76799=CARTESIAN_POINT('Ctrl Pts',(0.146984512649617,0.253157526346722,
-1.9608));
#76800=CARTESIAN_POINT('Ctrl Pts',(0.156416973582358,0.246404567355291,
-1.9608));
#76801=CARTESIAN_POINT('Ctrl Pts',(0.165404046449669,0.239034332280283,
-1.9608));
#76802=CARTESIAN_POINT('Ctrl Pts',(0.173915563696922,0.231109827924898,
-1.9608));
#76803=CARTESIAN_POINT('Ctrl Pts',(0.178983715958836,0.226391210373337,
-1.9608));
#76804=CARTESIAN_POINT('Ctrl Pts',(0.183884248765666,0.221474694998783,
-1.9608));
#76805=CARTESIAN_POINT('Ctrl Pts',(0.188605652765418,0.216376747084418,
-1.9608));
#76806=CARTESIAN_POINT('Ctrl Pts',(0.194496179098994,0.210016436372108,
-1.9608));
#76807=CARTESIAN_POINT('Ctrl Pts',(0.200097635413564,0.203384895024988,
-1.9608));
#76808=CARTESIAN_POINT('Ctrl Pts',(0.205392638302791,0.196515230368162,
-1.9608));
#76809=CARTESIAN_POINT('Ctrl Pts',(0.212203122093379,0.187679401423239,
-1.9608));
#76810=CARTESIAN_POINT('Ctrl Pts',(0.218510175211099,0.178446116869452,
-1.9608));
#76811=CARTESIAN_POINT('Ctrl Pts',(0.224281484638061,0.168869554768253,
-1.9608));
#76812=CARTESIAN_POINT('Ctrl Pts',(0.22751782490307,0.163499367305478,-1.9608));
#76813=CARTESIAN_POINT('Ctrl Pts',(0.230586998760227,0.158018286713927,
-1.9608));
#76814=CARTESIAN_POINT('Ctrl Pts',(0.233476785545442,0.152446119292306,
-1.9608));
#76815=CARTESIAN_POINT('Ctrl Pts',(0.237406871706289,0.144868017620003,
-1.9608));
#76816=CARTESIAN_POINT('Ctrl Pts',(0.240998077474448,0.137136337286731,
-1.9608));
#76817=CARTESIAN_POINT('Ctrl Pts',(0.244237996620259,0.129277760874839,
-1.9608));
#76818=CARTESIAN_POINT('Ctrl Pts',(0.250537692111831,0.113997552893049,
-1.9608));
#76819=CARTESIAN_POINT('Ctrl Pts',(0.255513873420495,0.0982344656391996,
-1.9608));
#76820=CARTESIAN_POINT('Ctrl Pts',(0.259043884351174,0.0821679460335087,
-1.9608));
#76821=CARTESIAN_POINT('Ctrl Pts',(0.260467944208438,0.0756864687617066,
-1.9608));
#76822=CARTESIAN_POINT('Ctrl Pts',(0.261656067894151,0.0691556200203403,
-1.9608));
#76823=CARTESIAN_POINT('Ctrl Pts',(0.262597734038404,0.0625875582041159,
-1.9608));
#76824=CARTESIAN_POINT('Ctrl Pts',(0.263470407024643,0.0565007193027163,
-1.9608));
#76825=CARTESIAN_POINT('Ctrl Pts',(0.264131287375213,0.0503777548586035,
-1.9608));
#76826=CARTESIAN_POINT('Ctrl Pts',(0.26456994765883,0.0442583426162408,
-1.9608));
#76827=CARTESIAN_POINT('Ctrl Pts',(0.265334619145271,0.0335909988190579,
-1.9608));
#76828=CARTESIAN_POINT('Ctrl Pts',(0.265427901586744,0.022920104419746,
-1.9608));
#76829=CARTESIAN_POINT('Ctrl Pts',(0.264815004423569,0.0122950415847356,
-1.9608));
#76830=CARTESIAN_POINT('Ctrl Pts',(0.263869571843309,-0.00409478883881043,
-1.9608));
#76831=CARTESIAN_POINT('Ctrl Pts',(0.261245615493676,-0.0203764095907301,
-1.9608));
#76832=CARTESIAN_POINT('Ctrl Pts',(0.257049826563265,-0.0363442073303925,
-1.9608));
#76833=CARTESIAN_POINT('Ctrl Pts',(0.25528111713989,-0.0430753358025595,
-1.9608));
#76834=CARTESIAN_POINT('Ctrl Pts',(0.253229675597862,-0.0497567776443664,
-1.9608));
#76835=CARTESIAN_POINT('Ctrl Pts',(0.250916504864508,-0.0563328026274767,
-1.9608));
#76836=CARTESIAN_POINT('Ctrl Pts',(0.245894613969703,-0.0706093449987376,
-1.9608));
#76837=CARTESIAN_POINT('Ctrl Pts',(0.239635781072895,-0.0844231946567744,
-1.9608));
#76838=CARTESIAN_POINT('Ctrl Pts',(0.232232690107956,-0.097615126217959,
-1.9608));
#76839=CARTESIAN_POINT('Ctrl Pts',(0.226848422394677,-0.107209617426709,
-1.9608));
#76840=CARTESIAN_POINT('Ctrl Pts',(0.220857960469645,-0.11647482010455,
-1.9608));
#76841=CARTESIAN_POINT('Ctrl Pts',(0.214287232483329,-0.125338313944058,
-1.9608));
#76842=CARTESIAN_POINT('Ctrl Pts',(0.210193048601064,-0.130861107414408,
-1.9608));
#76843=CARTESIAN_POINT('Ctrl Pts',(0.205869486213015,-0.136231200486207,
-1.9608));
#76844=CARTESIAN_POINT('Ctrl Pts',(0.201350239334785,-0.141399126486128,
-1.9608));
#76845=CARTESIAN_POINT('Ctrl Pts',(0.191610974505686,-0.152536336133355,
-1.9608));
#76846=CARTESIAN_POINT('Ctrl Pts',(0.180942748192052,-0.162770241399539,
-1.9608));
#76847=CARTESIAN_POINT('Ctrl Pts',(0.169418754522685,-0.17192999128596,
-1.9608));
#76848=CARTESIAN_POINT('Ctrl Pts',(0.159472693097453,-0.179835534938963,
-1.9608));
#76849=CARTESIAN_POINT('Ctrl Pts',(0.148888342042439,-0.186940774148992,
-1.9608));
#76850=CARTESIAN_POINT('Ctrl Pts',(0.137702479013108,-0.19310620885576,
-1.9608));
#76851=CARTESIAN_POINT('Ctrl Pts',(0.170904093888077,-0.23991444519679,
-1.99394055716378));
#76852=CARTESIAN_POINT('Ctrl Pts',(0.250758961454554,-0.183034120394509,
-1.9886433188887));
#76853=CARTESIAN_POINT('Ctrl Pts',(0.347776689926164,0.0157071971072416,
-1.97805143725563));
#76854=CARTESIAN_POINT('Ctrl Pts',(0.174902784065685,0.301363500003521,
-1.96216491226457));
#76855=CARTESIAN_POINT('Ctrl Pts',(-0.158317247439313,0.310026665536666,
-1.94628098219058));
#76856=CARTESIAN_POINT('Ctrl Pts',(-0.346428810985269,0.035126883458298,
-1.9303970521166));
#76857=CARTESIAN_POINT('Ctrl Pts',(-0.217232984403476,-0.272179277325897,
-1.91451312204261));
#76858=CARTESIAN_POINT('Ctrl Pts',(0.110983315678744,-0.330033805723321,
-1.89862919196862));
#76859=CARTESIAN_POINT('Ctrl Pts',(0.337520707764598,-0.0856199548585268,
-1.88274526189463));
#76860=CARTESIAN_POINT('Ctrl Pts',(0.254874981231195,0.237259528375207,
-1.86686133182064));
#76861=CARTESIAN_POINT('Ctrl Pts',(-0.0612546449745717,0.342778004190948,
-1.85097740174666));
#76862=CARTESIAN_POINT('Ctrl Pts',(-0.321269693814492,0.134300259451662,
-1.83509347167267));
#76863=CARTESIAN_POINT('Ctrl Pts',(-0.28698334628375,-0.197209240948837,
-1.81920954159868));
#76864=CARTESIAN_POINT('Ctrl Pts',(0.0101973733548513,-0.34806082496865,
-1.80332561152469));
#76865=CARTESIAN_POINT('Ctrl Pts',(0.298036451033343,-0.180069148869172,
-1.7874416814507));
#76866=CARTESIAN_POINT('Ctrl Pts',(0.312856429901399,0.152877314430839,
-1.77155775137671));
#76867=CARTESIAN_POINT('Ctrl Pts',(0.041081132865898,0.345778658064987,
-1.75567382130273));
#76868=CARTESIAN_POINT('Ctrl Pts',(-0.268326906005064,0.22192624403291,
-1.73978989122873));
#76869=CARTESIAN_POINT('Ctrl Pts',(-0.331931460478688,-0.105223985707714,
-1.72390596115475));
#76870=CARTESIAN_POINT('Ctrl Pts',(-0.0914669254283658,-0.335982697609461,
-1.70802203108076));
#76871=CARTESIAN_POINT('Ctrl Pts',(0.232786781689362,-0.258961180118152,
-1.69213810100677));
#76872=CARTESIAN_POINT('Ctrl Pts',(0.34379386966368,0.0552842881121883,
-1.67625417093279));
#76873=CARTESIAN_POINT('Ctrl Pts',(0.139865199476729,0.31888603304783,-1.6603702408588));
#76874=CARTESIAN_POINT('Ctrl Pts',(-0.192188362092366,0.290369093748387,
-1.64448631078481));
#76875=CARTESIAN_POINT('Ctrl Pts',(-0.348185884034223,-0.00414331274272311,
-1.62860238071082));
#76876=CARTESIAN_POINT('Ctrl Pts',(-0.18522430098761,-0.294860195792014,
-1.61271845063683));
#76877=CARTESIAN_POINT('Ctrl Pts',(0.14741382526022,-0.315467495963393,
-1.59683452056285));
#76878=CARTESIAN_POINT('Ctrl Pts',(0.345012066558079,-0.0470876923556176,
-1.58095059048886));
#76879=CARTESIAN_POINT('Ctrl Pts',(0.226558609757863,0.264427254971228,
-1.56506666041487));
#76880=CARTESIAN_POINT('Ctrl Pts',(-0.0994360905582914,0.333711013816492,
-1.54918273034088));
#76881=CARTESIAN_POINT('Ctrl Pts',(-0.334341381795663,0.0972955151030245,
-1.53329880026689));
#76882=CARTESIAN_POINT('Ctrl Pts',(-0.26296996072181,-0.228248497468949,
-1.5174148701929));
#76883=CARTESIAN_POINT('Ctrl Pts',(0.0492976801743824,-0.344703228257538,
-1.50153094011892));
#76884=CARTESIAN_POINT('Ctrl Pts',(0.316405696118587,-0.145389175333612,
-1.48564701004493));
#76885=CARTESIAN_POINT('Ctrl Pts',(0.29366716108482,0.187110062104603,-1.46976307997094));
#76886=CARTESIAN_POINT('Ctrl Pts',(0.00191193381121215,0.34820528621762,
-1.45387914989695));
#76887=CARTESIAN_POINT('Ctrl Pts',(-0.291594739241419,0.190323631972808,
-1.43799521982296));
#76888=CARTESIAN_POINT('Ctrl Pts',(-0.317983182473595,-0.141905857893761,
-1.42211128974898));
#76889=CARTESIAN_POINT('Ctrl Pts',(-0.0530800028323548,-0.344141090455598,
-1.40622735967499));
#76890=CARTESIAN_POINT('Ctrl Pts',(0.260447635646281,-0.231122491174878,
-1.390343429601));
#76891=CARTESIAN_POINT('Ctrl Pts',(0.335389655002547,0.0936181401112829,
-1.37445949952701));
#76892=CARTESIAN_POINT('Ctrl Pts',(0.103094681066654,0.332598953059679,
-1.35857556945302));
#76893=CARTESIAN_POINT('Ctrl Pts',(-0.223641189786869,0.266899222687776,
-1.34269163937903));
#76894=CARTESIAN_POINT('Ctrl Pts',(-0.345508348378294,-0.0432961665916229,
-1.32680770930505));
#76895=CARTESIAN_POINT('Ctrl Pts',(-0.150869185055043,-0.313829676483047,
-1.31092377923106));
#76896=CARTESIAN_POINT('Ctrl Pts',(0.181975179607525,-0.296876423529109,
-1.29503984915707));
#76897=CARTESIAN_POINT('Ctrl Pts',(0.348119390575748,-0.00796660189769713,
-1.27915591908308));
#76898=CARTESIAN_POINT('Ctrl Pts',(0.195365408734829,0.288241103783793,
-1.26327198900909));
#76899=CARTESIAN_POINT('Ctrl Pts',(-0.136354977936102,0.320402710401569,
-1.24738805893511));
#76900=CARTESIAN_POINT('Ctrl Pts',(-0.343166045501201,0.0590562617822472,
-1.23150412886112));
#76901=CARTESIAN_POINT('Ctrl Pts',(-0.235616480747601,-0.25638925648463,
-1.21562019878713));
#76902=CARTESIAN_POINT('Ctrl Pts',(0.0877718793749992,-0.336966873789705,
-1.19973626871314));
#76903=CARTESIAN_POINT('Ctrl Pts',(0.330755945827384,-0.10886267101472,
-1.18385233863915));
#76904=CARTESIAN_POINT('Ctrl Pts',(0.270747773867585,0.218966252619836,
-1.16796840856517));
#76905=CARTESIAN_POINT('Ctrl Pts',(-0.0372815601730543,0.346208986179863,
-1.15208447849118));
#76906=CARTESIAN_POINT('Ctrl Pts',(-0.31115875421187,0.156303571673662,
-1.13620054841719));
#76907=CARTESIAN_POINT('Ctrl Pts',(-0.299995910030472,-0.176785267501611,
-1.1203166183432));
#76908=CARTESIAN_POINT('Ctrl Pts',(-0.0140188608700629,-0.347928223029595,
-1.10443268826921));
#76909=CARTESIAN_POINT('Ctrl Pts',(0.284800303718939,-0.200348106659949,
-1.08854875819523));
#76910=CARTESIAN_POINT('Ctrl Pts',(0.322725347996934,0.130762863997715,
-1.07266482812124));
#76911=CARTESIAN_POINT('Ctrl Pts',(0.0650146620166612,0.34208722654242,
-1.05678089804725));
#76912=CARTESIAN_POINT('Ctrl Pts',(-0.252253344769326,0.240039219489886,
-1.04089696797326));
#76913=CARTESIAN_POINT('Ctrl Pts',(-0.338442193212666,-0.0818990762708986,
-1.02501303789927));
#76914=CARTESIAN_POINT('Ctrl Pts',(-0.114597740703191,-0.328812917426232,
-1.00912910782529));
#76915=CARTESIAN_POINT('Ctrl Pts',(0.214225099680103,-0.274514450453299,
-0.993245177751293));
#76916=CARTESIAN_POINT('Ctrl Pts',(0.346804929786502,0.0312556797463465,
-0.977361247677308));
#76917=CARTESIAN_POINT('Ctrl Pts',(0.161690691822444,0.308393736996402,
-0.961477317603318));
#76918=CARTESIAN_POINT('Ctrl Pts',(-0.171541895225696,0.303024677250884,
-0.94559338752933));
#76919=CARTESIAN_POINT('Ctrl Pts',(-0.347631841388322,0.020066880514706,
-0.929709457455343));
#76920=CARTESIAN_POINT('Ctrl Pts',(-0.205270218971837,-0.281273379550714,
-0.913825527381354));
#76921=CARTESIAN_POINT('Ctrl Pts',(0.125131207143578,-0.324950392890079,
-0.897941597307366));
#76922=CARTESIAN_POINT('Ctrl Pts',(0.340904959815935,-0.070953401705074,
-0.882057667233379));
#76923=CARTESIAN_POINT('Ctrl Pts',(0.244389369957919,0.248041151207208,
-0.866173737159389));
#76924=CARTESIAN_POINT('Ctrl Pts',(-0.0760015067447896,0.339815167132293,
-0.850289807085402));
#76925=CARTESIAN_POINT('Ctrl Pts',(-0.326770455431364,0.12029815583709,
-0.834405877011414));
#76926=CARTESIAN_POINT('Ctrl Pts',(-0.278198113395417,-0.209419164700504,
-0.818521946937425));
#76927=CARTESIAN_POINT('Ctrl Pts',(0.025220347548139,-0.347295998983832,
-0.802638016863437));
#76928=CARTESIAN_POINT('Ctrl Pts',(0.305535460982617,-0.167028916426965,
-0.78675408678945));
#76929=CARTESIAN_POINT('Ctrl Pts',(0.305961809285915,0.166246648384607,
-0.77087015671546));
#76930=CARTESIAN_POINT('Ctrl Pts',(0.0261088319000491,0.347230335278244,
-0.754986226641474));
#76931=CARTESIAN_POINT('Ctrl Pts',(-0.27766139782707,0.210130257215241,
-0.739102296567485));
#76932=CARTESIAN_POINT('Ctrl Pts',(-0.327077172223595,-0.119461710396439,
-0.723218366493496));
#76933=CARTESIAN_POINT('Ctrl Pts',(-0.0768706849623521,-0.339619602841245,
-0.70733443641951));
#76934=CARTESIAN_POINT('Ctrl Pts',(0.243753949572878,-0.248665616658693,
-0.69145050634552));
#76935=CARTESIAN_POINT('Ctrl Pts',(0.341085380358906,0.0700809542318726,
-0.675566576271533));
#76936=CARTESIAN_POINT('Ctrl Pts',(0.125962192601037,0.324629177486809,
-0.659682646197544));
#76937=CARTESIAN_POINT('Ctrl Pts',(-0.204549901004051,0.281797648747914,
-0.643798716123556));
#76938=CARTESIAN_POINT('Ctrl Pts',(-0.347682045271716,-0.0191773886733094,
-0.627914786049569));
#76939=CARTESIAN_POINT('Ctrl Pts',(-0.172316631198822,-0.302584790518111,
-0.61203085597558));
#76940=CARTESIAN_POINT('Ctrl Pts',(0.160901128269999,-0.30880641794178,
-0.596146925901592));
#76941=CARTESIAN_POINT('Ctrl Pts',(0.346723826115746,-0.032142887929545,
-0.580262995827604));
#76942=CARTESIAN_POINT('Ctrl Pts',(0.214926751705743,0.273965450817477,
-0.564379065753616));
#76943=CARTESIAN_POINT('Ctrl Pts',(-0.113756088221019,0.329105042855812,
-0.548495135679626));
#76944=CARTESIAN_POINT('Ctrl Pts',(-0.338231544314204,0.082764722391689,
-0.532611205605641));
#76945=CARTESIAN_POINT('Ctrl Pts',(-0.252866666444601,-0.239393036323237,
-0.51672727553165));
#76946=CARTESIAN_POINT('Ctrl Pts',(0.0641392091112833,-0.342252448778347,
-0.500843345457664));
#76947=CARTESIAN_POINT('Ctrl Pts',(0.322389731130484,-0.131588138179558,
-0.484959415383675));
#76948=CARTESIAN_POINT('Ctrl Pts',(0.285311967982603,0.199618781062624,
-0.469075485309687));
#76949=CARTESIAN_POINT('Ctrl Pts',(-0.0131286304801114,0.347962951912657,
-0.453191555235699));
#76950=CARTESIAN_POINT('Ctrl Pts',(-0.299542617972748,0.177552237117127,
-0.437307625161711));
#76951=CARTESIAN_POINT('Ctrl Pts',(-0.311557642847234,-0.155506951363366,
-0.421423695087722));
#76952=CARTESIAN_POINT('Ctrl Pts',(-0.0381672241935123,-0.346112467094931,
-0.405539765013735));
#76953=CARTESIAN_POINT('Ctrl Pts',(0.270186656754355,-0.219658251927647,
-0.389655834939746));
#76954=CARTESIAN_POINT('Ctrl Pts',(0.331033390463177,0.108016065916605,
-0.373771904865758));
#76955=CARTESIAN_POINT('Ctrl Pts',(0.0886337337118425,0.336741204159362,
-0.35788797479177));
#76956=CARTESIAN_POINT('Ctrl Pts',(-0.234959734190297,0.25699124857999,
-0.342004044717782));
#76957=CARTESIAN_POINT('Ctrl Pts',(-0.343316011856417,-0.0581780675448442,
-0.326120114643794));
#76958=CARTESIAN_POINT('Ctrl Pts',(-0.137174305814673,-0.320052794782354,
-0.310236184569806));
#76959=CARTESIAN_POINT('Ctrl Pts',(0.194627323824718,-0.288740006056718,
-0.294352254495817));
#76960=CARTESIAN_POINT('Ctrl Pts',(0.348138580916076,0.00707589771753539,
-0.27846832442183));
#76961=CARTESIAN_POINT('Ctrl Pts',(0.182734252248176,0.296409871720789,
-0.262584394347841));
#76962=CARTESIAN_POINT('Ctrl Pts',(-0.150065942415735,0.31421463595112,
-0.246700464273853));
#76963=CARTESIAN_POINT('Ctrl Pts',(-0.34539607339384,0.0441800496300475,
-0.230816534199865));
#76964=CARTESIAN_POINT('Ctrl Pts',(-0.224324033250605,-0.26632621700842,
-0.214932604125877));
#76965=CARTESIAN_POINT('Ctrl Pts',(0.102244728201643,-0.332861519865864,
-0.199048674051889));
#76966=CARTESIAN_POINT('Ctrl Pts',(0.335146456388876,-0.0944761581462219,
-0.183164743977901));
#76967=CARTESIAN_POINT('Ctrl Pts',(0.261043037650893,0.23045579262935,-0.167280813903913));
#76968=CARTESIAN_POINT('Ctrl Pts',(-0.0522087338317124,0.344274967070772,
-0.151396883829924));
#76969=CARTESIAN_POINT('Ctrl Pts',(-0.317601115841721,0.142720497810793,
-0.135512953755936));
#76970=CARTESIAN_POINT('Ctrl Pts',(-0.292115037072835,-0.189579887209652,
-0.119629023681948));
#76971=CARTESIAN_POINT('Ctrl Pts',(0.00108660914303244,-0.348203443840996,
-0.103745093607961));
#76972=CARTESIAN_POINT('Ctrl Pts',(0.293061778238414,-0.187871440927789,
-0.0878611635339722));
#76973=CARTESIAN_POINT('Ctrl Pts',(0.31702060395061,0.144599030699003,-0.0719772334599843));
#76974=CARTESIAN_POINT('Ctrl Pts',(0.04967936712779,0.344541914343505,-0.056093303385996));
#76975=CARTESIAN_POINT('Ctrl Pts',(-0.157537689676105,0.267491347263654,
-0.045504016670004));
#76976=CARTESIAN_POINT('Ctrl Pts',(-0.221960127786206,0.193651371357618,
-0.0402093733120079));
#76977=CARTESIAN_POINT('Ctrl Pts',(0.159723474619028,-0.224219139087579,
-1.98281477796869));
#76978=CARTESIAN_POINT('Ctrl Pts',(0.234354202431277,-0.171059949578467,
-1.97751753969362));
#76979=CARTESIAN_POINT('Ctrl Pts',(0.325024989412419,0.0146796255222407,
-1.96692565806054));
#76980=CARTESIAN_POINT('Ctrl Pts',(0.163460568766758,0.281648170320817,
-1.95103913306949));
#76981=CARTESIAN_POINT('Ctrl Pts',(-0.147960065074204,0.289744587841742,
-1.9351552029955));
#76982=CARTESIAN_POINT('Ctrl Pts',(-0.323765289291095,0.0328288676465,-1.91927127292151));
#76983=CARTESIAN_POINT('Ctrl Pts',(-0.203021509206835,-0.254373192032829,
-1.90338734284752));
#76984=CARTESIAN_POINT('Ctrl Pts',(0.103722739471405,-0.308442852319218,
-1.88750341277353));
#76985=CARTESIAN_POINT('Ctrl Pts',(0.315439958011422,-0.0800186606160754,
-1.87161948269955));
#76986=CARTESIAN_POINT('Ctrl Pts',(0.238200950425248,0.22173790806543,-1.85573555262556));
#76987=CARTESIAN_POINT('Ctrl Pts',(-0.0572473397758462,0.320353319846208,
-1.83985162255157));
#76988=CARTESIAN_POINT('Ctrl Pts',(-0.300252092377886,0.125514278762123,
-1.82396769247758));
#76989=CARTESIAN_POINT('Ctrl Pts',(-0.268208772437333,-0.184307727654305,
-1.8080837624036));
#76990=CARTESIAN_POINT('Ctrl Pts',(0.00953025680760637,-0.325290536218316,
-1.7921998323296));
#76991=CARTESIAN_POINT('Ctrl Pts',(0.278538778324083,-0.168288947764529,
-1.77631590225562));
#76992=CARTESIAN_POINT('Ctrl Pts',(0.292389227805628,0.142876014820982,
-1.76043197218163));
#76993=CARTESIAN_POINT('Ctrl Pts',(0.0383935874989864,0.323157669654262,
-1.74454804210764));
#76994=CARTESIAN_POINT('Ctrl Pts',(-0.250772844499381,0.20740773377436,
-1.72866411203365));
#76995=CARTESIAN_POINT('Ctrl Pts',(-0.310216361684961,-0.098340187342182,
-1.71278018195966));
#76996=CARTESIAN_POINT('Ctrl Pts',(-0.0854831198584704,-0.314002565141601,
-1.69689625188568));
#76997=CARTESIAN_POINT('Ctrl Pts',(0.217557770389958,-0.242019828424955,
-1.68101232181169));
#76998=CARTESIAN_POINT('Ctrl Pts',(0.321302726963141,0.0516675662251906,
-1.6651283917377));
#76999=CARTESIAN_POINT('Ctrl Pts',(0.130715158019189,0.29802437172297,-1.64924446166371));
#77000=CARTESIAN_POINT('Ctrl Pts',(-0.179615316850372,0.271373022847792,
-1.63336053158972));
#77001=CARTESIAN_POINT('Ctrl Pts',(-0.325407413866073,-0.00387225544248687,
-1.61747660151573));
#77002=CARTESIAN_POINT('Ctrl Pts',(-0.173106847615926,-0.275570315065653,
-1.60159267144175));
#77003=CARTESIAN_POINT('Ctrl Pts',(0.137769949459867,-0.294829476803729,
-1.58570874136776));
#77004=CARTESIAN_POINT('Ctrl Pts',(0.322441228893183,-0.0440071952855393,
-1.56982481129377));
#77005=CARTESIAN_POINT('Ctrl Pts',(0.211737048142804,0.247128310312073,
-1.55394088121978));
#77006=CARTESIAN_POINT('Ctrl Pts',(-0.0929309387808109,0.311879495878635,
-1.53805695114579));
#77007=CARTESIAN_POINT('Ctrl Pts',(-0.312468624913705,0.0909304006917473,
-1.52217302107181));
#77008=CARTESIAN_POINT('Ctrl Pts',(-0.245766352878728,-0.213316382673595,
-1.50628909099782));
#77009=CARTESIAN_POINT('Ctrl Pts',(0.0460726047514509,-0.322152594926988,
-1.49040516092383));
#77010=CARTESIAN_POINT('Ctrl Pts',(0.295706299501574,-0.135877753001558,
-1.47452123084984));
#77011=CARTESIAN_POINT('Ctrl Pts',(0.274455329201714,0.174869241430234,
-1.45863730077585));
#77012=CARTESIAN_POINT('Ctrl Pts',(0.0017868542796178,0.325425546750295,
-1.44275337070187));
#77013=CARTESIAN_POINT('Ctrl Pts',(-0.272518486085944,0.177872578176609,
-1.42686944062788));
#77014=CARTESIAN_POINT('Ctrl Pts',(-0.297180586021304,-0.1326223156856,
-1.41098551055389));
#77015=CARTESIAN_POINT('Ctrl Pts',(-0.0496074862356628,-0.321627232421633,
-1.3951015804799));
#77016=CARTESIAN_POINT('Ctrl Pts',(0.243409039393625,-0.216002358476167,
-1.37921765040591));
#77017=CARTESIAN_POINT('Ctrl Pts',(0.313448319636893,0.0874936011523395,
-1.36333372033192));
#77018=CARTESIAN_POINT('Ctrl Pts',(0.0963501827258152,0.310840186614447,
-1.34744979025794));
#77019=CARTESIAN_POINT('Ctrl Pts',(-0.20901048704009,0.249438560838261,
-1.33156586018395));
#77020=CARTESIAN_POINT('Ctrl Pts',(-0.322905043743439,-0.0404637127664561,
-1.31568193010996));
#77021=CARTESIAN_POINT('Ctrl Pts',(-0.140999258131951,-0.293298804177649,
-1.29979800003597));
#77022=CARTESIAN_POINT('Ctrl Pts',(0.170070285152855,-0.277454640317703,
-1.28391406996198));
#77023=CARTESIAN_POINT('Ctrl Pts',(0.325345270438228,-0.0074454233778606,
-1.268030139888));
#77024=CARTESIAN_POINT('Ctrl Pts',(0.18258451973613,0.269384246901198,-1.25214620981401));
#77025=CARTESIAN_POINT('Ctrl Pts',(-0.127434576680288,0.299441827392426,
-1.23626227974002));
#77026=CARTESIAN_POINT('Ctrl Pts',(-0.320715975327185,0.0551927757567259,
-1.22037834966603));
#77027=CARTESIAN_POINT('Ctrl Pts',(-0.220202349319727,-0.239616161140838,
-1.20449441959204));
#77028=CARTESIAN_POINT('Ctrl Pts',(0.082029805305883,-0.314922356093178,
-1.18861048951806));
#77029=CARTESIAN_POINT('Ctrl Pts',(0.309117749707331,-0.101740828292656,
-1.17272655944407));
#77030=CARTESIAN_POINT('Ctrl Pts',(0.253035338145952,0.204641386271602,
-1.15684262937008));
#77031=CARTESIAN_POINT('Ctrl Pts',(-0.0348425844845974,0.323559845518928,
-1.14095869929609));
#77032=CARTESIAN_POINT('Ctrl Pts',(-0.290802614789294,0.146078124842525,
-1.1250747692221));
#77033=CARTESIAN_POINT('Ctrl Pts',(-0.28037004867153,-0.1652198993273,-1.10919083914812));
#77034=CARTESIAN_POINT('Ctrl Pts',(-0.0131017409672661,-0.3251666091551,
-1.09330690907413));
#77035=CARTESIAN_POINT('Ctrl Pts',(0.266168545455288,-0.18724124742165,
-1.07742297900014));
#77036=CARTESIAN_POINT('Ctrl Pts',(0.301612517038136,0.12220830123899,-1.06153904892615));
#77037=CARTESIAN_POINT('Ctrl Pts',(0.0607613748871524,0.319707733168315,
-1.04565511885216));
#77038=CARTESIAN_POINT('Ctrl Pts',(-0.235750822547378,0.224335750592797,
-1.02977118877818));
#77039=CARTESIAN_POINT('Ctrl Pts',(-0.316301159485464,-0.0765412035047192,
-1.01388725870419));
#77040=CARTESIAN_POINT('Ctrl Pts',(-0.107100707257433,-0.307301835059209,
-0.998003328630197));
#77041=CARTESIAN_POINT('Ctrl Pts',(0.200210401594721,-0.256555597130681,
-0.982119398556207));
#77042=CARTESIAN_POINT('Ctrl Pts',(0.324116802238711,0.029210919745057,
-0.96623546848222));
#77043=CARTESIAN_POINT('Ctrl Pts',(0.151112817276033,0.288218486188343,
-0.950351538408232));
#77044=CARTESIAN_POINT('Ctrl Pts',(-0.160319550719043,0.283200672638755,
-0.934467608334243));
#77045=CARTESIAN_POINT('Ctrl Pts',(-0.32488961692817,0.0187540965675897,
-0.918583678260256));
#77046=CARTESIAN_POINT('Ctrl Pts',(-0.191841353030792,-0.262872354181862,
-0.902699748186266));
#77047=CARTESIAN_POINT('Ctrl Pts',(0.116945069796483,-0.303691998538148,
-0.88681581811228));
#77048=CARTESIAN_POINT('Ctrl Pts',(0.318602810839161,-0.0663115996729461,
-0.870931888038291));
#77049=CARTESIAN_POINT('Ctrl Pts',(0.228401312347713,0.231814192498305,
-0.855047957964302));
#77050=CARTESIAN_POINT('Ctrl Pts',(-0.0710294555115186,0.317584312861226,
-0.839164027890315));
#77051=CARTESIAN_POINT('Ctrl Pts',(-0.305392991805803,0.11242819878349,
-0.823280097816326));
#77052=CARTESIAN_POINT('Ctrl Pts',(-0.259998273260052,-0.195718872946862,
-0.807396167742339));
#77053=CARTESIAN_POINT('Ctrl Pts',(0.0235704215729706,-0.324575745478112,
-0.79151223766835));
#77054=CARTESIAN_POINT('Ctrl Pts',(0.285547199819738,-0.156101812932796,
-0.775628307594363));
#77055=CARTESIAN_POINT('Ctrl Pts',(0.285945656233808,0.155370721201957,
-0.759744377520373));
#77056=CARTESIAN_POINT('Ctrl Pts',(0.0244007808967447,0.324514377520363,
-0.743860447446387));
#77057=CARTESIAN_POINT('Ctrl Pts',(-0.259496669854845,0.196383445483687,
-0.727976517372397));
#77058=CARTESIAN_POINT('Ctrl Pts',(-0.305679643053672,-0.111646473963038,
-0.71209258729841));
#77059=CARTESIAN_POINT('Ctrl Pts',(-0.0718417717165509,-0.317401542470144,
-0.696208657224421));
#77060=CARTESIAN_POINT('Ctrl Pts',(0.227807461437338,-0.232397805151584,
-0.680324727150434));
#77061=CARTESIAN_POINT('Ctrl Pts',(0.318771428192673,0.0654962280883837,
-0.664440797076445));
#77062=CARTESIAN_POINT('Ctrl Pts',(0.117721691828191,0.303391797184606,
-0.648556867002457));
#77063=CARTESIAN_POINT('Ctrl Pts',(-0.191168158574021,0.263362325462871,
-0.632672936928469));
#77064=CARTESIAN_POINT('Ctrl Pts',(-0.324936536451937,-0.0179227956647243,
-0.616789006854481));
#77065=CARTESIAN_POINT('Ctrl Pts',(-0.161043603131856,-0.282789563485085,
-0.600905076780493));
#77066=CARTESIAN_POINT('Ctrl Pts',(0.150374907310509,-0.288604169368921,
-0.585021146706504));
#77067=CARTESIAN_POINT('Ctrl Pts',(0.32404100440495,-0.030040086387625,
-0.569137216632518));
#77068=CARTESIAN_POINT('Ctrl Pts',(0.200866151243303,0.256042513286972,
-0.553253286558528));
#77069=CARTESIAN_POINT('Ctrl Pts',(-0.106314116042351,0.307574849517642,
-0.537369356484541));
#77070=CARTESIAN_POINT('Ctrl Pts',(-0.316104291328467,0.0773502186842683,
-0.521485426410552));
#77071=CARTESIAN_POINT('Ctrl Pts',(-0.236324020455074,-0.223731841006614,
-0.505601496336565));
#77072=CARTESIAN_POINT('Ctrl Pts',(0.059943194487078,-0.319862146494561,
-0.489717566262575));
#77073=CARTESIAN_POINT('Ctrl Pts',(0.301298856371324,-0.122979585629188,
-0.473833636188588));
#77074=CARTESIAN_POINT('Ctrl Pts',(0.266646736422932,0.186559634618336,
-0.4579497061146));
#77075=CARTESIAN_POINT('Ctrl Pts',(-0.0122697498320095,0.325199066059707,
-0.442065776040612));
#77076=CARTESIAN_POINT('Ctrl Pts',(-0.279946411175029,0.165936693460959,
-0.426181845966624));
#77077=CARTESIAN_POINT('Ctrl Pts',(-0.291175407958708,-0.145333619775284,
-0.410297915892635));
#77078=CARTESIAN_POINT('Ctrl Pts',(-0.035670307984215,-0.323469640754012,
-0.394413985818648));
#77079=CARTESIAN_POINT('Ctrl Pts',(0.252510929555415,-0.205288114687303,
-0.378530055744659));
#77080=CARTESIAN_POINT('Ctrl Pts',(0.309377043795816,0.100949608463896,
-0.362646125670671));
#77081=CARTESIAN_POINT('Ctrl Pts',(0.0828352767616206,0.314711449867035,
-0.346762195596683));
#77082=CARTESIAN_POINT('Ctrl Pts',(-0.219588567404444,0.240178770654608,
-0.330878265522695));
#77083=CARTESIAN_POINT('Ctrl Pts',(-0.320856130818992,-0.0543720333637462,
-0.314994335448707));
#77084=CARTESIAN_POINT('Ctrl Pts',(-0.128200303776929,-0.299114803403398,
-0.299110405374719));
#77085=CARTESIAN_POINT('Ctrl Pts',(0.181894720658038,-0.26985051077302,
-0.283226475300731));
#77086=CARTESIAN_POINT('Ctrl Pts',(0.325363205338246,0.00661298944795382,
-0.267342545226742));
#77087=CARTESIAN_POINT('Ctrl Pts',(0.170779698935137,0.277018610529187,
-0.251458615152755));
#77088=CARTESIAN_POINT('Ctrl Pts',(-0.140248563971308,0.293658579431881,
-0.235574685078766));
#77089=CARTESIAN_POINT('Ctrl Pts',(-0.322800113836719,0.0412897717966501,
-0.219690755004778));
#77090=CARTESIAN_POINT('Ctrl Pts',(-0.209648658590971,-0.248903041436704,
-0.20380682493079));
#77091=CARTESIAN_POINT('Ctrl Pts',(0.0955558341425081,-0.31108557618733,
-0.187922894856802));
#77092=CARTESIAN_POINT('Ctrl Pts',(0.313221031181045,-0.0882954872786916,
-0.172038964782814));
#77093=CARTESIAN_POINT('Ctrl Pts',(0.243965489943215,0.215379275636006,
-0.156155034708826));
#77094=CARTESIAN_POINT('Ctrl Pts',(-0.0487932160274783,0.321752350771107,
-0.140271104634837));
#77095=CARTESIAN_POINT('Ctrl Pts',(-0.296823514352684,0.13338366150916,
-0.124387174560849));
#77096=CARTESIAN_POINT('Ctrl Pts',(-0.273004745809628,-0.17717748951549,
-0.108503244486861));
#77097=CARTESIAN_POINT('Ctrl Pts',(0.00101552270592162,-0.325423824902742,
-0.0926193144128733));
#77098=CARTESIAN_POINT('Ctrl Pts',(0.273889550761288,-0.175580810523597,
-0.0767353843388852));
#77099=CARTESIAN_POINT('Ctrl Pts',(0.296280979798966,0.135139299968517,
-0.0608514542648971));
#77100=CARTESIAN_POINT('Ctrl Pts',(0.0464293215803309,0.322001834238538,
-0.044967524190909));
#77101=CARTESIAN_POINT('Ctrl Pts',(-0.147231506314883,0.249991948369916,
-0.0343782374749169));
#77102=CARTESIAN_POINT('Ctrl Pts',(-0.207439400837955,0.180982615420753,
-0.0290835941169209));
#77103=CARTESIAN_POINT('Ctrl Pts',(0.14854285534998,-0.208523832978368,
-1.9716889987736));
#77104=CARTESIAN_POINT('Ctrl Pts',(0.217949443407999,-0.159085778762425,
-1.96639176049853));
#77105=CARTESIAN_POINT('Ctrl Pts',(0.302273288898672,0.0136520539372401,
-1.95579987886546));
#77106=CARTESIAN_POINT('Ctrl Pts',(0.15201835346783,0.261932840638111,-1.9399133538744));
#77107=CARTESIAN_POINT('Ctrl Pts',(-0.137602882709094,0.269462510146818,
-1.92402942380041));
#77108=CARTESIAN_POINT('Ctrl Pts',(-0.301101767596918,0.0305308518347021,
-1.90814549372642));
#77109=CARTESIAN_POINT('Ctrl Pts',(-0.188810034010194,-0.23656710673976,
-1.89226156365243));
#77110=CARTESIAN_POINT('Ctrl Pts',(0.0964621632640678,-0.286851898915114,
-1.87637763357845));
#77111=CARTESIAN_POINT('Ctrl Pts',(0.293359208258245,-0.0744173663736239,
-1.86049370350446));
#77112=CARTESIAN_POINT('Ctrl Pts',(0.2215269196193,0.206216287755652,-1.84460977343047));
#77113=CARTESIAN_POINT('Ctrl Pts',(-0.0532400345771204,0.29792863550147,
-1.82872584335648));
#77114=CARTESIAN_POINT('Ctrl Pts',(-0.27923449094128,0.116728298072583,
-1.81284191328249));
#77115=CARTESIAN_POINT('Ctrl Pts',(-0.249434198590917,-0.171406214359773,
-1.79695798320851));
#77116=CARTESIAN_POINT('Ctrl Pts',(0.00886314026036145,-0.302520247467981,
-1.78107405313452));
#77117=CARTESIAN_POINT('Ctrl Pts',(0.259041105614823,-0.156508746659887,
-1.76519012306053));
#77118=CARTESIAN_POINT('Ctrl Pts',(0.271922025709858,0.132874715211126,
-1.74930619298654));
#77119=CARTESIAN_POINT('Ctrl Pts',(0.0357060421320745,0.300536681243538,
-1.73342226291256));
#77120=CARTESIAN_POINT('Ctrl Pts',(-0.233218782993697,0.192889223515808,
-1.71753833283856));
#77121=CARTESIAN_POINT('Ctrl Pts',(-0.288501262891236,-0.0914563889766494,
-1.70165440276458));
#77122=CARTESIAN_POINT('Ctrl Pts',(-0.0794993142885749,-0.29202243267374,
-1.68577047269059));
#77123=CARTESIAN_POINT('Ctrl Pts',(0.202328759090555,-0.225078476731758,
-1.6698865426166));
#77124=CARTESIAN_POINT('Ctrl Pts',(0.298811584262604,0.0480508443381929,
-1.65400261254261));
#77125=CARTESIAN_POINT('Ctrl Pts',(0.121565116561649,0.277162710398109,
-1.63811868246863));
#77126=CARTESIAN_POINT('Ctrl Pts',(-0.167042271608378,0.252376951947197,
-1.62223475239464));
#77127=CARTESIAN_POINT('Ctrl Pts',(-0.302628943697925,-0.00360119814225005,
-1.60635082232065));
#77128=CARTESIAN_POINT('Ctrl Pts',(-0.160989394244243,-0.256280434339293,
-1.59046689224666));
#77129=CARTESIAN_POINT('Ctrl Pts',(0.128126073659514,-0.274191457644064,
-1.57458296217267));
#77130=CARTESIAN_POINT('Ctrl Pts',(0.299870391228289,-0.040926698215461,
-1.55869903209869));
#77131=CARTESIAN_POINT('Ctrl Pts',(0.196915486527744,0.229829365652916,
-1.5428151020247));
#77132=CARTESIAN_POINT('Ctrl Pts',(-0.0864257870033305,0.290047977940778,
-1.52693117195071));
#77133=CARTESIAN_POINT('Ctrl Pts',(-0.290595868031748,0.0845652862804702,
-1.51104724187672));
#77134=CARTESIAN_POINT('Ctrl Pts',(-0.228562745035647,-0.198384267878241,
-1.49516331180273));
#77135=CARTESIAN_POINT('Ctrl Pts',(0.042847529328519,-0.299601961596439,
-1.47927938172874));
#77136=CARTESIAN_POINT('Ctrl Pts',(0.275006902884562,-0.126366330669504,
-1.46339545165476));
#77137=CARTESIAN_POINT('Ctrl Pts',(0.255243497318609,0.162628420755865,
-1.44751152158077));
#77138=CARTESIAN_POINT('Ctrl Pts',(0.00166177474802338,0.302645807282969,
-1.43162759150678));
#77139=CARTESIAN_POINT('Ctrl Pts',(-0.25344223293047,0.165421524380412,
-1.41574366143279));
#77140=CARTESIAN_POINT('Ctrl Pts',(-0.276377989569012,-0.123338773477437,
-1.3998597313588));
#77141=CARTESIAN_POINT('Ctrl Pts',(-0.046134969638971,-0.299113374387668,
-1.38397580128481));
#77142=CARTESIAN_POINT('Ctrl Pts',(0.226370443140969,-0.200882225777455,
-1.36809187121083));
#77143=CARTESIAN_POINT('Ctrl Pts',(0.291506984271239,0.0813690621933957,
-1.35220794113684));
#77144=CARTESIAN_POINT('Ctrl Pts',(0.0896056843849767,0.289081420169215,
-1.33632401106285));
#77145=CARTESIAN_POINT('Ctrl Pts',(-0.194379784293312,0.231977898988746,
-1.32044008098886));
#77146=CARTESIAN_POINT('Ctrl Pts',(-0.300301739108585,-0.037631258941289,
-1.30455615091488));
#77147=CARTESIAN_POINT('Ctrl Pts',(-0.13112933120886,-0.272767931872252,
-1.28867222084089));
#77148=CARTESIAN_POINT('Ctrl Pts',(0.158165390698187,-0.258032857106295,
-1.2727882907669));
#77149=CARTESIAN_POINT('Ctrl Pts',(0.302571150300708,-0.0069242448580246,
-1.25690436069291));
#77150=CARTESIAN_POINT('Ctrl Pts',(0.169803630737432,0.250527390018603,
-1.24102043061892));
#77151=CARTESIAN_POINT('Ctrl Pts',(-0.118514175424474,0.278480944383283,
-1.22513650054494));
#77152=CARTESIAN_POINT('Ctrl Pts',(-0.298265905153167,0.051329289731205,
-1.20925257047095));
#77153=CARTESIAN_POINT('Ctrl Pts',(-0.204788217891854,-0.222843065797045,
-1.19336864039696));
#77154=CARTESIAN_POINT('Ctrl Pts',(0.0762877312367668,-0.292877838396651,
-1.17748471032297));
#77155=CARTESIAN_POINT('Ctrl Pts',(0.287479553587276,-0.0946189855705929,
-1.16160078024898));
#77156=CARTESIAN_POINT('Ctrl Pts',(0.23532290242432,0.190316519923368,-1.14571685017499));
#77157=CARTESIAN_POINT('Ctrl Pts',(-0.0324036087961405,0.300910704857994,
-1.12983292010101));
#77158=CARTESIAN_POINT('Ctrl Pts',(-0.270446475366719,0.135852678011388,
-1.11394899002702));
#77159=CARTESIAN_POINT('Ctrl Pts',(-0.260744187312589,-0.153654531152992,
-1.09806505995303));
#77160=CARTESIAN_POINT('Ctrl Pts',(-0.0121846210644688,-0.302404995280605,
-1.08218112987904));
#77161=CARTESIAN_POINT('Ctrl Pts',(0.247536787191636,-0.174134388183351,
-1.06629719980505));
#77162=CARTESIAN_POINT('Ctrl Pts',(0.280499686079339,0.113653738480264,
-1.05041326973106));
#77163=CARTESIAN_POINT('Ctrl Pts',(0.0565080877576434,0.297328239794208,
-1.03452933965708));
#77164=CARTESIAN_POINT('Ctrl Pts',(-0.219248300325429,0.208632281695709,
-1.01864540958309));
#77165=CARTESIAN_POINT('Ctrl Pts',(-0.29416012575826,-0.0711833307385401,
-1.0027614795091));
#77166=CARTESIAN_POINT('Ctrl Pts',(-0.0996036738116745,-0.285790752692184,
-0.986877549435108));
#77167=CARTESIAN_POINT('Ctrl Pts',(0.186195703509339,-0.238596743808063,
-0.970993619361121));
#77168=CARTESIAN_POINT('Ctrl Pts',(0.30142867469092,0.0271661597437678,
-0.955109689287132));
#77169=CARTESIAN_POINT('Ctrl Pts',(0.140534942729621,0.268043235380283,
-0.939225759213145));
#77170=CARTESIAN_POINT('Ctrl Pts',(-0.14909720621239,0.263376668026626,
-0.923341829139156));
#77171=CARTESIAN_POINT('Ctrl Pts',(-0.302147392468019,0.0174413126204732,
-0.907457899065168));
#77172=CARTESIAN_POINT('Ctrl Pts',(-0.178412487089747,-0.244471328813009,
-0.891573968991181));
#77173=CARTESIAN_POINT('Ctrl Pts',(0.108758932449388,-0.282433604186218,
-0.875690038917191));
#77174=CARTESIAN_POINT('Ctrl Pts',(0.296300661862387,-0.061669797640818,
-0.859806108843205));
#77175=CARTESIAN_POINT('Ctrl Pts',(0.212413254737507,0.215587233789401,
-0.843922178769215));
#77176=CARTESIAN_POINT('Ctrl Pts',(-0.0660574042782473,0.295353458590158,
-0.828038248695228));
#77177=CARTESIAN_POINT('Ctrl Pts',(-0.284015528180242,0.10455824172989,
-0.812154318621239));
#77178=CARTESIAN_POINT('Ctrl Pts',(-0.241798433124689,-0.18201858119322,
-0.796270388547252));
#77179=CARTESIAN_POINT('Ctrl Pts',(0.0219204955978022,-0.301855491972392,
-0.780386458473262));
#77180=CARTESIAN_POINT('Ctrl Pts',(0.265558938656859,-0.145174709438629,
-0.764502528399276));
#77181=CARTESIAN_POINT('Ctrl Pts',(0.2659295031817,0.144494794019306,-0.748618598325286));
#77182=CARTESIAN_POINT('Ctrl Pts',(0.0226927298934404,0.301798419762482,
-0.7327346682513));
#77183=CARTESIAN_POINT('Ctrl Pts',(-0.241331941882621,0.182636633752132,
-0.71685073817731));
#77184=CARTESIAN_POINT('Ctrl Pts',(-0.284282113883749,-0.103831237529635,
-0.700966808103323));
#77185=CARTESIAN_POINT('Ctrl Pts',(-0.0668128584707501,-0.295183482099042,
-0.685082878029334));
#77186=CARTESIAN_POINT('Ctrl Pts',(0.2118609733018,-0.216129993644475,-0.669198947955347));
#77187=CARTESIAN_POINT('Ctrl Pts',(0.29645747602644,0.0609115019448947,
-0.653315017881357));
#77188=CARTESIAN_POINT('Ctrl Pts',(0.109481191055346,0.282154416882402,
-0.637431087807371));
#77189=CARTESIAN_POINT('Ctrl Pts',(-0.177786416143992,0.244927002177829,
-0.621547157733382));
#77190=CARTESIAN_POINT('Ctrl Pts',(-0.302191027632159,-0.0166682026561393,
-0.605663227659394));
#77191=CARTESIAN_POINT('Ctrl Pts',(-0.149770575064891,-0.262994336452061,
-0.589779297585406));
#77192=CARTESIAN_POINT('Ctrl Pts',(0.139848686351021,-0.268401920796062,
-0.573895367511417));
#77193=CARTESIAN_POINT('Ctrl Pts',(0.301358182694155,-0.0279372848457049,
-0.558011437437431));
#77194=CARTESIAN_POINT('Ctrl Pts',(0.186805550780861,0.238119575756467,
-0.542127507363441));
#77195=CARTESIAN_POINT('Ctrl Pts',(-0.0988721438636844,0.286044656179471,
-0.526243577289453));
#77196=CARTESIAN_POINT('Ctrl Pts',(-0.29397703834273,0.0719357149768477,
-0.510359647215465));
#77197=CARTESIAN_POINT('Ctrl Pts',(-0.21978137446555,-0.208070645689991,
-0.494475717141477));
#77198=CARTESIAN_POINT('Ctrl Pts',(0.0557471798628727,-0.297471844210775,
-0.478591787067489));
#77199=CARTESIAN_POINT('Ctrl Pts',(0.280207981612165,-0.114371033078817,
-0.462707856993501));
#77200=CARTESIAN_POINT('Ctrl Pts',(0.247981504863259,0.173500488174049,
-0.446823926919513));
#77201=CARTESIAN_POINT('Ctrl Pts',(-0.0114108691839076,0.302435180206757,
-0.430939996845525));
#77202=CARTESIAN_POINT('Ctrl Pts',(-0.26035020437731,0.154321149804791,
-0.415056066771537));
#77203=CARTESIAN_POINT('Ctrl Pts',(-0.270793173070181,-0.135160288187202,
-0.399172136697548));
#77204=CARTESIAN_POINT('Ctrl Pts',(-0.0331733917749176,-0.300826814413094,
-0.383288206623561));
#77205=CARTESIAN_POINT('Ctrl Pts',(0.234835202356476,-0.19091797744696,
-0.367404276549572));
#77206=CARTESIAN_POINT('Ctrl Pts',(0.287720697128454,0.0938831510111875,
-0.351520346475584));
#77207=CARTESIAN_POINT('Ctrl Pts',(0.0770368198113984,0.292681695574709,
-0.335636416401596));
#77208=CARTESIAN_POINT('Ctrl Pts',(-0.204217400618593,0.223366292729226,
-0.319752486327608));
#77209=CARTESIAN_POINT('Ctrl Pts',(-0.298396249781567,-0.0505659991826476,
-0.30386855625362));
#77210=CARTESIAN_POINT('Ctrl Pts',(-0.119226301739186,-0.278176812024444,
-0.287984626179632));
#77211=CARTESIAN_POINT('Ctrl Pts',(0.169162117491358,-0.250961015489323,
-0.272100696105643));
#77212=CARTESIAN_POINT('Ctrl Pts',(0.302587829760414,0.00615008117837171,
-0.256216766031655));
#77213=CARTESIAN_POINT('Ctrl Pts',(0.158825145622099,0.257627349337584,
-0.240332835957668));
#77214=CARTESIAN_POINT('Ctrl Pts',(-0.13043118552688,0.273102522912643,
-0.224448905883679));
#77215=CARTESIAN_POINT('Ctrl Pts',(-0.3002041542796,0.0383994939632529,
-0.208564975809691));
#77216=CARTESIAN_POINT('Ctrl Pts',(-0.194973283931337,-0.231479865864986,
-0.192681045735703));
#77217=CARTESIAN_POINT('Ctrl Pts',(0.0888669400833733,-0.289309632508797,
-0.176797115661715));
#77218=CARTESIAN_POINT('Ctrl Pts',(0.291295605973215,-0.0821148164111612,
-0.160913185587726));
#77219=CARTESIAN_POINT('Ctrl Pts',(0.226887942235539,0.200302758642664,
-0.145029255513739));
#77220=CARTESIAN_POINT('Ctrl Pts',(-0.0453776982232441,0.299229734471443,
-0.12914532543975));
#77221=CARTESIAN_POINT('Ctrl Pts',(-0.276045912863647,0.124046825207526,
-0.113261395365762));
#77222=CARTESIAN_POINT('Ctrl Pts',(-0.253894454546419,-0.164775091821329,
-0.0973774652917741));
#77223=CARTESIAN_POINT('Ctrl Pts',(0.000944436268810345,-0.302644205964487,
-0.0814935352177862));
#77224=CARTESIAN_POINT('Ctrl Pts',(0.254717323284163,-0.163290180119405,
-0.0656096051437982));
#77225=CARTESIAN_POINT('Ctrl Pts',(0.275541355647321,0.125679569238032,
-0.0497256750698101));
#77226=CARTESIAN_POINT('Ctrl Pts',(0.0431792760328719,0.29946175413357,
-0.0338417449958219));
#77227=CARTESIAN_POINT('Ctrl Pts',(-0.136925322953661,0.23249254947618,
-0.0232524582798299));
#77228=CARTESIAN_POINT('Ctrl Pts',(-0.192918673889705,0.168313859483889,
-0.0179578149218338));
#77229=CARTESIAN_POINT('Ctrl Pts',(0.137362236080932,-0.192828526869157,
-1.96056321957851));
#77230=CARTESIAN_POINT('Ctrl Pts',(0.201544684384722,-0.147111607946385,
-1.95526598130344));
#77231=CARTESIAN_POINT('Ctrl Pts',(0.279521588384925,0.0126244823522396,
-1.94467409967037));
#77232=CARTESIAN_POINT('Ctrl Pts',(0.140576138168903,0.242217510955405,
-1.9287875746793));
#77233=CARTESIAN_POINT('Ctrl Pts',(-0.127245700343985,0.249180432451894,
-1.91290364460532));
#77234=CARTESIAN_POINT('Ctrl Pts',(-0.278438245902744,0.0282328360229038,
-1.89701971453133));
#77235=CARTESIAN_POINT('Ctrl Pts',(-0.174598558813552,-0.218761021446692,
-1.88113578445734));
#77236=CARTESIAN_POINT('Ctrl Pts',(0.0892015870567291,-0.265260945511011,
-1.86525185438335));
#77237=CARTESIAN_POINT('Ctrl Pts',(0.271278458505069,-0.0688160721311721,
-1.84936792430937));
#77238=CARTESIAN_POINT('Ctrl Pts',(0.204852888813353,0.190694667445875,
-1.83348399423537));
#77239=CARTESIAN_POINT('Ctrl Pts',(-0.0492327293783949,0.275503951156731,
-1.81760006416139));
#77240=CARTESIAN_POINT('Ctrl Pts',(-0.258216889504675,0.107942317383044,
-1.8017161340874));
#77241=CARTESIAN_POINT('Ctrl Pts',(-0.2306596247445,-0.158504701065241,
-1.78583220401341));
#77242=CARTESIAN_POINT('Ctrl Pts',(0.00819602371311662,-0.279749958717647,
-1.76994827393942));
#77243=CARTESIAN_POINT('Ctrl Pts',(0.239543432905563,-0.144728545555244,
-1.75406434386544));
#77244=CARTESIAN_POINT('Ctrl Pts',(0.251454823614088,0.122873415601269,
-1.73818041379144));
#77245=CARTESIAN_POINT('Ctrl Pts',(0.0330184967651629,0.277915692832815,
-1.72229648371746));
#77246=CARTESIAN_POINT('Ctrl Pts',(-0.215664721488012,0.178370713257257,
-1.70641255364347));
#77247=CARTESIAN_POINT('Ctrl Pts',(-0.266786164097509,-0.0845725906111169,
-1.69052862356948));
#77248=CARTESIAN_POINT('Ctrl Pts',(-0.0735155087186798,-0.270042300205881,
-1.67464469349549));
#77249=CARTESIAN_POINT('Ctrl Pts',(0.187099747791151,-0.208137125038562,
-1.65876076342151));
#77250=CARTESIAN_POINT('Ctrl Pts',(0.276320441562065,0.0444341224511951,
-1.64287683334751));
#77251=CARTESIAN_POINT('Ctrl Pts',(0.112415075104108,0.256301049073249,
-1.62699290327353));
#77252=CARTESIAN_POINT('Ctrl Pts',(-0.154469226366385,0.233380881046602,
-1.61110897319954));
#77253=CARTESIAN_POINT('Ctrl Pts',(-0.279850473529776,-0.00333014084201356,
-1.59522504312556));
#77254=CARTESIAN_POINT('Ctrl Pts',(-0.14887194087256,-0.236990553612932,
-1.57934111305156));
#77255=CARTESIAN_POINT('Ctrl Pts',(0.118482197859161,-0.2535534384844,-1.56345718297758));
#77256=CARTESIAN_POINT('Ctrl Pts',(0.277299553563392,-0.0378462011453827,
-1.54757325290359));
#77257=CARTESIAN_POINT('Ctrl Pts',(0.182093924912684,0.212530420993761,
-1.5316893228296));
#77258=CARTESIAN_POINT('Ctrl Pts',(-0.0799206352258501,0.268216460002921,
-1.51580539275561));
#77259=CARTESIAN_POINT('Ctrl Pts',(-0.26872311114979,0.0782001718691929,
-1.49992146268163));
#77260=CARTESIAN_POINT('Ctrl Pts',(-0.211359137192565,-0.183452153082888,
-1.48403753260764));
#77261=CARTESIAN_POINT('Ctrl Pts',(0.0396224539055875,-0.27705132826589,
-1.46815360253365));
#77262=CARTESIAN_POINT('Ctrl Pts',(0.25430750626755,-0.116854908337451,
-1.45226967245966));
#77263=CARTESIAN_POINT('Ctrl Pts',(0.236031665435503,0.150387600081495,
-1.43638574238567));
#77264=CARTESIAN_POINT('Ctrl Pts',(0.00153669521642899,0.279866067815646,
-1.42050181231168));
#77265=CARTESIAN_POINT('Ctrl Pts',(-0.234365979774995,0.152970470584214,
-1.4046178822377));
#77266=CARTESIAN_POINT('Ctrl Pts',(-0.255575393116723,-0.114055231269275,
-1.38873395216371));
#77267=CARTESIAN_POINT('Ctrl Pts',(-0.0426624530422791,-0.276599516353704,
-1.37285002208972));
#77268=CARTESIAN_POINT('Ctrl Pts',(0.209331846888312,-0.185762093078744,
-1.35696609201573));
#77269=CARTESIAN_POINT('Ctrl Pts',(0.269565648905586,0.0752445232344523,
-1.34108216194174));
#77270=CARTESIAN_POINT('Ctrl Pts',(0.0828611860441382,0.267322653723983,
-1.32519823186776));
#77271=CARTESIAN_POINT('Ctrl Pts',(-0.179749081546533,0.214517237139231,
-1.30931430179377));
#77272=CARTESIAN_POINT('Ctrl Pts',(-0.277698434473732,-0.0347988051161221,
-1.29343037171978));
#77273=CARTESIAN_POINT('Ctrl Pts',(-0.121259404285768,-0.252237059566854,
-1.27754644164579));
#77274=CARTESIAN_POINT('Ctrl Pts',(0.146260496243518,-0.238611073894888,
-1.2616625115718));
#77275=CARTESIAN_POINT('Ctrl Pts',(0.279797030163189,-0.00640306633818836,
-1.24577858149781));
#77276=CARTESIAN_POINT('Ctrl Pts',(0.157022741738734,0.231670533136009,
-1.22989465142383));
#77277=CARTESIAN_POINT('Ctrl Pts',(-0.10959377416866,0.25752006137414,-1.21401072134984));
#77278=CARTESIAN_POINT('Ctrl Pts',(-0.27581583497915,0.0474658037056839,
-1.19812679127585));
#77279=CARTESIAN_POINT('Ctrl Pts',(-0.189374086463979,-0.206069970453253,
-1.18224286120186));
#77280=CARTESIAN_POINT('Ctrl Pts',(0.0705456571676509,-0.270833320700124,
-1.16635893112788));
#77281=CARTESIAN_POINT('Ctrl Pts',(0.265841357467223,-0.0874971428485293,
-1.15047500105388));
#77282=CARTESIAN_POINT('Ctrl Pts',(0.217610466702688,0.175991653575135,
-1.1345910709799));
#77283=CARTESIAN_POINT('Ctrl Pts',(-0.0299646331076837,0.278261564197058,
-1.11870714090591));
#77284=CARTESIAN_POINT('Ctrl Pts',(-0.250090335944144,0.125627231180252,
-1.10282321083192));
#77285=CARTESIAN_POINT('Ctrl Pts',(-0.241118325953647,-0.142089162978682,
-1.08693928075793));
#77286=CARTESIAN_POINT('Ctrl Pts',(-0.0112675011616718,-0.279643381406111,
-1.07105535068396));
#77287=CARTESIAN_POINT('Ctrl Pts',(0.228905028927986,-0.161027528945051,
-1.05517142060996));
#77288=CARTESIAN_POINT('Ctrl Pts',(0.259386855120543,0.105099175721539,
-1.03928749053597));
#77289=CARTESIAN_POINT('Ctrl Pts',(0.0522548006281345,0.274948746420102,
-1.02340356046198));
#77290=CARTESIAN_POINT('Ctrl Pts',(-0.202745778103481,0.192928812798621,
-1.00751963038799));
#77291=CARTESIAN_POINT('Ctrl Pts',(-0.272019092031057,-0.0658254579723609,
-0.991635700314011));
#77292=CARTESIAN_POINT('Ctrl Pts',(-0.0921066403659162,-0.26427967032516,
-0.975751770240021));
#77293=CARTESIAN_POINT('Ctrl Pts',(0.172181005423957,-0.220637890485445,
-0.959867840166033));
#77294=CARTESIAN_POINT('Ctrl Pts',(0.278740547143128,0.0251213997424785,
-0.943983910092046));
#77295=CARTESIAN_POINT('Ctrl Pts',(0.12995706818321,0.247867984572224,-0.928099980018057));
#77296=CARTESIAN_POINT('Ctrl Pts',(-0.137874861705736,0.243552663414497,
-0.912216049944069));
#77297=CARTESIAN_POINT('Ctrl Pts',(-0.279405168007867,0.0161285286733566,
-0.896332119870082));
#77298=CARTESIAN_POINT('Ctrl Pts',(-0.164983621148702,-0.226070303444157,
-0.880448189796093));
#77299=CARTESIAN_POINT('Ctrl Pts',(0.100572795102292,-0.261175209834287,
-0.864564259722106));
#77300=CARTESIAN_POINT('Ctrl Pts',(0.273998512885612,-0.05702799560869,
-0.848680329648117));
#77301=CARTESIAN_POINT('Ctrl Pts',(0.196425197127302,0.199360275080499,
-0.832796399574128));
#77302=CARTESIAN_POINT('Ctrl Pts',(-0.0610853530449764,0.273122604319091,
-0.816912469500142));
#77303=CARTESIAN_POINT('Ctrl Pts',(-0.26263806455468,0.0966882846762901,
-0.801028539426152));
#77304=CARTESIAN_POINT('Ctrl Pts',(-0.223598592989326,-0.168318289439578,
-0.785144609352165));
#77305=CARTESIAN_POINT('Ctrl Pts',(0.0202705696226342,-0.279135238466673,
-0.769260679278176));
#77306=CARTESIAN_POINT('Ctrl Pts',(0.245570677493981,-0.13424760594446,
-0.753376749204189));
#77307=CARTESIAN_POINT('Ctrl Pts',(0.245913350129593,0.133618866836656,
-0.737492819130199));
#77308=CARTESIAN_POINT('Ctrl Pts',(0.0209846788901358,0.279082462004602,
-0.721608889056213));
#77309=CARTESIAN_POINT('Ctrl Pts',(-0.223167213910397,0.168889822020577,
-0.705724958982223));
#77310=CARTESIAN_POINT('Ctrl Pts',(-0.262884584713825,-0.0960160010962316,
-0.689841028908236));
#77311=CARTESIAN_POINT('Ctrl Pts',(-0.0617839452249487,-0.272965421727941,
-0.673957098834247));
#77312=CARTESIAN_POINT('Ctrl Pts',(0.195914485166261,-0.199862182137365,
-0.65807316876026));
#77313=CARTESIAN_POINT('Ctrl Pts',(0.274143523860207,0.0563267758014057,
-0.642189238686271));
#77314=CARTESIAN_POINT('Ctrl Pts',(0.1012406902825,0.260917036580199,-0.626305308612284));
#77315=CARTESIAN_POINT('Ctrl Pts',(-0.164404673713962,0.226491678892785,
-0.610421378538294));
#77316=CARTESIAN_POINT('Ctrl Pts',(-0.27944551881238,-0.015413609647554,
-0.594537448464308));
#77317=CARTESIAN_POINT('Ctrl Pts',(-0.138497546997926,-0.243199109419036,
-0.578653518390318));
#77318=CARTESIAN_POINT('Ctrl Pts',(0.129322465391532,-0.248199672223202,
-0.562769588316331));
#77319=CARTESIAN_POINT('Ctrl Pts',(0.27867536098336,-0.0258344833037851,
-0.546885658242343));
#77320=CARTESIAN_POINT('Ctrl Pts',(0.172744950318421,0.220196638225962,
-0.531001728168355));
#77321=CARTESIAN_POINT('Ctrl Pts',(-0.0914301716850177,0.264514462841301,
-0.515117798094366));
#77322=CARTESIAN_POINT('Ctrl Pts',(-0.271849785356991,0.0665212112694271,
-0.499233868020378));
#77323=CARTESIAN_POINT('Ctrl Pts',(-0.203238728476024,-0.192409450373368,
-0.483349937946391));
#77324=CARTESIAN_POINT('Ctrl Pts',(0.0515511652386677,-0.275081541926988,
-0.467466007872402));
#77325=CARTESIAN_POINT('Ctrl Pts',(0.259117106853005,-0.105762480528446,
-0.451582077798414));
#77326=CARTESIAN_POINT('Ctrl Pts',(0.229316273303587,0.160441341729761,
-0.435698147724425));
#77327=CARTESIAN_POINT('Ctrl Pts',(-0.0105519885358059,0.279671294353807,
-0.419814217650438));
#77328=CARTESIAN_POINT('Ctrl Pts',(-0.240753997579591,0.142705606148622,
-0.403930287576449));
#77329=CARTESIAN_POINT('Ctrl Pts',(-0.250410938181655,-0.12498695659912,
-0.388046357502461));
#77330=CARTESIAN_POINT('Ctrl Pts',(-0.03067647556562,-0.278183988072175,
-0.372162427428474));
#77331=CARTESIAN_POINT('Ctrl Pts',(0.217159475157536,-0.176547840206616,
-0.356278497354485));
#77332=CARTESIAN_POINT('Ctrl Pts',(0.266064350461092,0.086816693558479,
-0.340394567280497));
#77333=CARTESIAN_POINT('Ctrl Pts',(0.0712383628611763,0.270651941282383,
-0.324510637206509));
#77334=CARTESIAN_POINT('Ctrl Pts',(-0.18884623383274,0.206553814803844,
-0.308626707132521));
#77335=CARTESIAN_POINT('Ctrl Pts',(-0.275936368744142,-0.0467599650015497,
-0.292742777058533));
#77336=CARTESIAN_POINT('Ctrl Pts',(-0.110252299701442,-0.257238820645489,
-0.276858846984545));
#77337=CARTESIAN_POINT('Ctrl Pts',(0.156429514324678,-0.232071520205626,
-0.260974916910556));
#77338=CARTESIAN_POINT('Ctrl Pts',(0.279812454182582,0.00568717290878994,
-0.245090986836568));
#77339=CARTESIAN_POINT('Ctrl Pts',(0.14687059230906,0.238236088145982,-0.229207056762581));
#77340=CARTESIAN_POINT('Ctrl Pts',(-0.120613807082454,0.252546466393404,
-0.213323126688592));
#77341=CARTESIAN_POINT('Ctrl Pts',(-0.277608194722481,0.0355092161298553,
-0.197439196614604));
#77342=CARTESIAN_POINT('Ctrl Pts',(-0.180297909271702,-0.214056690293268,
-0.181555266540616));
#77343=CARTESIAN_POINT('Ctrl Pts',(0.0821780460242392,-0.267533688830265,
-0.165671336466628));
#77344=CARTESIAN_POINT('Ctrl Pts',(0.269370180765385,-0.0759341455436309,
-0.14978740639264));
#77345=CARTESIAN_POINT('Ctrl Pts',(0.209810394527861,0.18522624164932,-0.133903476318652));
#77346=CARTESIAN_POINT('Ctrl Pts',(-0.0419621804190102,0.27670711817178,
-0.118019546244663));
#77347=CARTESIAN_POINT('Ctrl Pts',(-0.255268311374609,0.114709988905893,
-0.102135616170675));
#77348=CARTESIAN_POINT('Ctrl Pts',(-0.234784163283211,-0.152372694127167,
-0.0862516860966871));
#77349=CARTESIAN_POINT('Ctrl Pts',(0.000873349831699318,-0.279864587026233,
-0.0703677560226992));
#77350=CARTESIAN_POINT('Ctrl Pts',(0.235545095807039,-0.150999549715214,
-0.0544838259487111));
#77351=CARTESIAN_POINT('Ctrl Pts',(0.254801731495678,0.116219838507545,
-0.038599895874723));
#77352=CARTESIAN_POINT('Ctrl Pts',(0.0399292304854129,0.276921674028602,
-0.0227159658007349));
#77353=CARTESIAN_POINT('Ctrl Pts',(-0.126619139592439,0.214993150582441,
-0.0121266790847428));
#77354=CARTESIAN_POINT('Ctrl Pts',(-0.178397946941454,0.155645103547024,
-0.00683203572674675));
#77355=CARTESIAN_POINT('Ctrl Pts',(0.133821547094406,0.262002735736212,
-1.9608));
#77356=CARTESIAN_POINT('Ctrl Pts',(0.132194727536144,0.262814729912177,
-1.9608));
#77357=CARTESIAN_POINT('Ctrl Pts',(0.130567907977882,0.263626724088142,
-1.9608));
#77358=CARTESIAN_POINT('Ctrl Pts',(0.12894108841962,0.264438718264107,-1.9608));
#77359=CARTESIAN_POINT('Origin',(0.,0.,-0.04));
#77360=CARTESIAN_POINT('',(-0.3342,4.09276960275046E-17,0.));
#77361=CARTESIAN_POINT('Origin',(0.,0.,0.));
#77362=CARTESIAN_POINT('Origin',(-0.3342,-4.09276960275045E-17,-0.04));
#77363=CARTESIAN_POINT('Origin',(0.48,0.,0.));
#77364=CARTESIAN_POINT('',(-0.48,-5.8783046359073E-17,3.46944695195361E-18));
#77365=CARTESIAN_POINT('Origin',(0.,0.,0.));
#77366=CARTESIAN_POINT('Origin',(0.,0.,0.6066185719505));
#77367=CARTESIAN_POINT('',(-0.25,0.144337567297406,0.588452994616207));
#77368=CARTESIAN_POINT('',(-0.25,-5.3231743852413E-17,0.566123895246948));
#77369=CARTESIAN_POINT('Ctrl Pts',(-0.25,0.144337567297406,0.588452994616208));
#77370=CARTESIAN_POINT('Ctrl Pts',(-0.25,0.0669872981077805,0.566123895246948));
#77371=CARTESIAN_POINT('Ctrl Pts',(-0.25,-7.58473177261421E-17,0.566123895246948));
#77372=CARTESIAN_POINT('',(1.76762539787485E-17,0.288675134594813,0.588452994616207));
#77373=CARTESIAN_POINT('Ctrl Pts',(1.76762539787485E-17,0.288675134594813,
0.588452994616207));
#77374=CARTESIAN_POINT('Ctrl Pts',(-0.125,0.21650635094611,0.546786327949541));
#77375=CARTESIAN_POINT('Ctrl Pts',(-0.25,0.144337567297406,0.588452994616207));
#77376=CARTESIAN_POINT('',(0.25,0.144337567297406,0.588452994616207));
#77377=CARTESIAN_POINT('Ctrl Pts',(0.25,0.144337567297406,0.588452994616207));
#77378=CARTESIAN_POINT('Ctrl Pts',(0.125,0.21650635094611,0.546786327949541));
#77379=CARTESIAN_POINT('Ctrl Pts',(1.76762539787485E-17,0.288675134594813,
0.588452994616207));
#77380=CARTESIAN_POINT('',(0.25,-0.144337567297407,0.588452994616207));
#77381=CARTESIAN_POINT('Ctrl Pts',(0.25,-0.144337567297407,0.588452994616207));
#77382=CARTESIAN_POINT('Ctrl Pts',(0.25,-2.77555756156289E-17,0.546786327949541));
#77383=CARTESIAN_POINT('Ctrl Pts',(0.25,0.144337567297406,0.588452994616207));
#77384=CARTESIAN_POINT('',(-5.30287619362454E-17,-0.288675134594813,0.588452994616207));
#77385=CARTESIAN_POINT('Ctrl Pts',(-5.30287619362454E-17,-0.288675134594813,
0.588452994616207));
#77386=CARTESIAN_POINT('Ctrl Pts',(0.125,-0.21650635094611,0.546786327949541));
#77387=CARTESIAN_POINT('Ctrl Pts',(0.25,-0.144337567297407,0.588452994616207));
#77388=CARTESIAN_POINT('',(-0.25,-0.144337567297406,0.588452994616207));
#77389=CARTESIAN_POINT('Ctrl Pts',(-0.25,-0.144337567297406,0.588452994616207));
#77390=CARTESIAN_POINT('Ctrl Pts',(-0.125,-0.21650635094611,0.546786327949541));
#77391=CARTESIAN_POINT('Ctrl Pts',(-5.30287619362454E-17,-0.288675134594813,
0.588452994616207));
#77392=CARTESIAN_POINT('Ctrl Pts',(-0.25,-7.58473177261421E-17,0.566123895246948));
#77393=CARTESIAN_POINT('Ctrl Pts',(-0.25,-0.0669872981077807,0.566123895246948));
#77394=CARTESIAN_POINT('Ctrl Pts',(-0.25,-0.144337567297406,0.588452994616208));
#77395=CARTESIAN_POINT('',(-0.308675134594813,3.78018015557916E-17,0.6));
#77396=CARTESIAN_POINT('',(-0.320138837486628,-3.92057002610754E-17,0.6066185719505));
#77397=CARTESIAN_POINT('Origin',(0.,0.,0.6));
#77398=CARTESIAN_POINT('Origin',(-5.55111512312578E-17,-0.288675134594813,
0.6));
#77399=CARTESIAN_POINT('',(-5.55111512312578E-17,-0.288675134594813,0.25));
#77400=CARTESIAN_POINT('',(-5.30287619362453E-17,-0.288675134594813,0.6));
#77401=CARTESIAN_POINT('',(-0.25,-0.144337567297406,0.25));
#77402=CARTESIAN_POINT('',(-0.25,-0.144337567297406,0.25));
#77403=CARTESIAN_POINT('',(-0.25,-0.144337567297406,0.6));
#77404=CARTESIAN_POINT('Origin',(0.25,-0.144337567297407,0.6));
#77405=CARTESIAN_POINT('',(0.25,-0.144337567297407,0.25));
#77406=CARTESIAN_POINT('',(0.25,-0.144337567297407,0.6));
#77407=CARTESIAN_POINT('',(-5.30287619362453E-17,-0.288675134594813,0.25));
#77408=CARTESIAN_POINT('Origin',(0.25,0.144337567297406,0.6));
#77409=CARTESIAN_POINT('',(0.25,0.144337567297406,0.25));
#77410=CARTESIAN_POINT('',(0.25,0.144337567297406,0.6));
#77411=CARTESIAN_POINT('',(0.25,-0.144337567297407,0.25));
#77412=CARTESIAN_POINT('Origin',(0.,0.,0.176894574169124));
#77413=CARTESIAN_POINT('',(0.,0.,0.102789148338248));
#77414=CARTESIAN_POINT('',(-0.243346949651439,2.98014062972907E-17,0.25));
#77415=CARTESIAN_POINT('',(-0.1225,-1.50019232895551E-17,0.176894574169124));
#77416=CARTESIAN_POINT('Origin',(0.,0.,0.25));
#77417=CARTESIAN_POINT('Origin',(0.,0.288675134594813,0.6));
#77418=CARTESIAN_POINT('',(2.77555756156289E-17,0.288675134594813,0.25));
#77419=CARTESIAN_POINT('',(1.76762539787485E-17,0.288675134594813,0.6));
#77420=CARTESIAN_POINT('',(0.25,0.144337567297406,0.25));
#77421=CARTESIAN_POINT('Origin',(-0.25,0.144337567297406,0.6));
#77422=CARTESIAN_POINT('',(-0.25,0.144337567297406,0.25));
#77423=CARTESIAN_POINT('',(-0.25,0.144337567297406,0.6));
#77424=CARTESIAN_POINT('',(1.76762539787485E-17,0.288675134594813,0.25));
#77425=CARTESIAN_POINT('Origin',(-0.25,-0.144337567297406,0.6));
#77426=CARTESIAN_POINT('',(-0.25,0.144337567297406,0.25));
#77427=CARTESIAN_POINT('Origin',(0.,0.,0.25));
#77428=CARTESIAN_POINT('Origin',(0.,0.,0.54));
#77429=CARTESIAN_POINT('',(-0.44,-5.38844591624835E-17,0.6));
#77430=CARTESIAN_POINT('Origin',(0.,0.,0.6));
#77431=CARTESIAN_POINT('',(-0.5,-6.12323399573677E-17,0.54));
#77432=CARTESIAN_POINT('Origin',(-0.44,-5.38844591624835E-17,0.54));
#77433=CARTESIAN_POINT('Origin',(0.,0.,0.54));
#77434=CARTESIAN_POINT('Origin',(0.,0.,0.31));
#77435=CARTESIAN_POINT('',(-0.5,-6.12323399573677E-17,0.02));
#77436=CARTESIAN_POINT('',(-0.5,-6.12323399573677E-17,0.31));
#77437=CARTESIAN_POINT('Origin',(0.,0.,0.02));
#77438=CARTESIAN_POINT('Origin',(0.,0.,0.6));
#77439=CARTESIAN_POINT('Origin',(0.255,0.,-2.));
#77440=CARTESIAN_POINT('',(-0.255,-3.12284933782575E-17,-2.));
#77441=CARTESIAN_POINT('Origin',(0.,0.,-2.));
#77442=CARTESIAN_POINT('Origin',(0.,0.,-1.9775));
#77443=CARTESIAN_POINT('',(-0.2775,-3.39839486763391E-17,-1.9775));
#77444=CARTESIAN_POINT('Origin',(0.,0.,0.01));
#77445=CARTESIAN_POINT('',(-0.49,-6.00076931582203E-17,0.01));
#86406=UNCERTAINTY_MEASURE_WITH_UNIT(LENGTH_MEASURE(0.001),#86430,
'DISTANCE_ACCURACY_VALUE',
'Maximum model space distance between geometric entities at asserted c
onnectivities');
#86409=UNCERTAINTY_MEASURE_WITH_UNIT(LENGTH_MEASURE(0.001),#86430,
'DISTANCE_ACCURACY_VALUE',
'Maximum model space distance between geometric entities at asserted c
onnectivities');
#86426=(
GEOMETRIC_REPRESENTATION_CONTEXT(3)
GLOBAL_UNCERTAINTY_ASSIGNED_CONTEXT((#86406))
GLOBAL_UNIT_ASSIGNED_CONTEXT((#86430,#86432,#86433))
REPRESENTATION_CONTEXT('','3D')
);
#86429=(
GEOMETRIC_REPRESENTATION_CONTEXT(3)
GLOBAL_UNCERTAINTY_ASSIGNED_CONTEXT((#86409))
GLOBAL_UNIT_ASSIGNED_CONTEXT((#86430,#86432,#86433))
REPRESENTATION_CONTEXT('','3D')
);
#86430=(
LENGTH_UNIT()
NAMED_UNIT(*)
SI_UNIT(.CENTI.,.METRE.)
);
#86432=(
NAMED_UNIT(*)
PLANE_ANGLE_UNIT()
SI_UNIT($,.RADIAN.)
);
#86433=(
NAMED_UNIT(*)
SI_UNIT($,.STERADIAN.)
SOLID_ANGLE_UNIT()
);
#86450=SHAPE_DEFINITION_REPRESENTATION(#86469,#86517);
#86469=PRODUCT_DEFINITION_SHAPE('',$,#86537);
#86517=SHAPE_REPRESENTATION('',(#17121),#86426);
#86520=PRODUCT_DEFINITION_CONTEXT('part definition',#86579,'design');
#86537=PRODUCT_DEFINITION('ISO 4762 M6x20 A2 SHCS',
'ISO 4762 M6x20 A2 SHCS',#86556,#86520);
#86556=PRODUCT_DEFINITION_FORMATION('',$,#86597);
#86579=APPLICATION_CONTEXT(
'Core Data for Automotive Mechanical Design Process');
#86580=PRODUCT_CONTEXT('part definition',#86579,'mechanical');
#86597=PRODUCT('ISO 4762 M6x20 A2 SHCS','ISO 4762 M6x20 A2 SHCS',$,(#86580));
#86616=PRESENTATION_STYLE_ASSIGNMENT((#86634));
#86634=SURFACE_STYLE_USAGE(.BOTH.,#86652);
#86652=SURFACE_SIDE_STYLE('',(#86670));
#86670=SURFACE_STYLE_FILL_AREA(#86688);
#86688=FILL_AREA_STYLE('Opaque(198,202,208)',(#86706));
#86706=FILL_AREA_STYLE_COLOUR('Opaque(198,202,208)',#86724);
#86724=COLOUR_RGB('Opaque(198,202,208)', 0.40784314, 0.44705882, 0.49803922);
ENDSEC;
END-ISO-10303-21;
